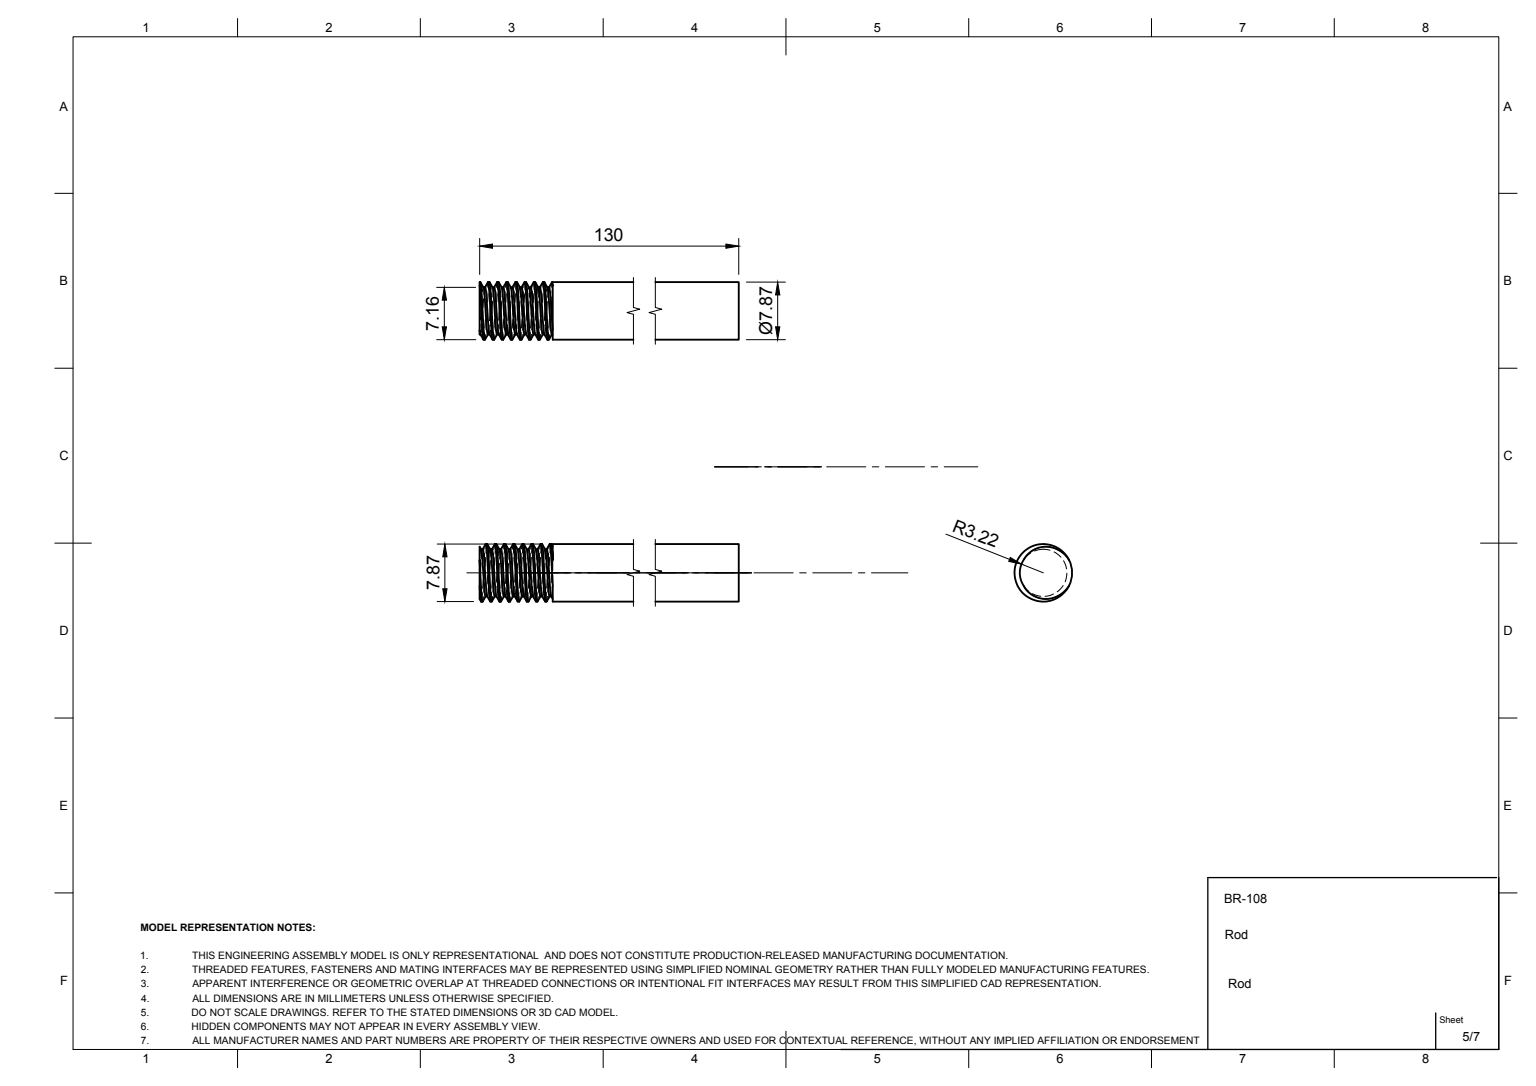
ISO-10303-21;
HEADER;
/* Generated by software containing ST-Developer
 * from STEP Tools, Inc. (www.steptools.com) 
 */

FILE_DESCRIPTION(
/* description */ (''),
/* implementation_level */ '2;1');

FILE_NAME(
/* name */ 'Rod.step',
/* time_stamp */ '2026-11-14T03:52:36-08:00',
/* author */ (''),
/* organization */ (''),
/* preprocessor_version */ 'ST-DEVELOPER v20.2',
/* originating_system */ 'Autodesk Translation Framework v15.17.0.0',
/* authorisation */ '');

FILE_SCHEMA (('AUTOMOTIVE_DESIGN { 1 0 10303 214 3 1 1 }'));
ENDSEC;

DATA;
#10=MECHANICAL_DESIGN_GEOMETRIC_PRESENTATION_REPRESENTATION('',(#193),#19443);
#43=B_SPLINE_SURFACE_WITH_KNOTS('',3,3,((#8954,#8955,#8956,#8957,#8958,
#8959,#8960,#8961,#8962,#8963,#8964,#8965,#8966,#8967,#8968,#8969,#8970,
#8971,#8972,#8973,#8974,#8975,#8976,#8977,#8978,#8979,#8980,#8981,#8982,
#8983,#8984,#8985,#8986,#8987,#8988,#8989,#8990,#8991,#8992,#8993,#8994,
#8995,#8996,#8997,#8998,#8999,#9000,#9001,#9002,#9003,#9004,#9005,#9006,
#9007,#9008,#9009),(#9010,#9011,#9012,#9013,#9014,#9015,#9016,#9017,#9018,
#9019,#9020,#9021,#9022,#9023,#9024,#9025,#9026,#9027,#9028,#9029,#9030,
#9031,#9032,#9033,#9034,#9035,#9036,#9037,#9038,#9039,#9040,#9041,#9042,
#9043,#9044,#9045,#9046,#9047,#9048,#9049,#9050,#9051,#9052,#9053,#9054,
#9055,#9056,#9057,#9058,#9059,#9060,#9061,#9062,#9063,#9064,#9065),(#9066,
#9067,#9068,#9069,#9070,#9071,#9072,#9073,#9074,#9075,#9076,#9077,#9078,
#9079,#9080,#9081,#9082,#9083,#9084,#9085,#9086,#9087,#9088,#9089,#9090,
#9091,#9092,#9093,#9094,#9095,#9096,#9097,#9098,#9099,#9100,#9101,#9102,
#9103,#9104,#9105,#9106,#9107,#9108,#9109,#9110,#9111,#9112,#9113,#9114,
#9115,#9116,#9117,#9118,#9119,#9120,#9121),(#9122,#9123,#9124,#9125,#9126,
#9127,#9128,#9129,#9130,#9131,#9132,#9133,#9134,#9135,#9136,#9137,#9138,
#9139,#9140,#9141,#9142,#9143,#9144,#9145,#9146,#9147,#9148,#9149,#9150,
#9151,#9152,#9153,#9154,#9155,#9156,#9157,#9158,#9159,#9160,#9161,#9162,
#9163,#9164,#9165,#9166,#9167,#9168,#9169,#9170,#9171,#9172,#9173,#9174,
#9175,#9176,#9177)),.UNSPECIFIED.,.F.,.F.,.F.,(4,4),(4,1,1,1,1,1,1,1,1,
1,1,1,1,1,1,1,1,1,1,1,1,1,1,1,1,1,1,1,1,1,1,1,1,1,1,1,1,1,1,1,1,1,1,1,1,
1,1,1,1,1,1,1,1,4),(-0.000657437329809864,0.0823479142293904),(8.31473274985805,
9.30202867542319,10.2893246009883,11.2766205265535,12.2639164521186,13.2512123776837,
14.2385083032489,15.225804228814,16.2131001543792,17.2003960799443,18.1876920055094,
19.1749879310746,20.1622838566397,21.1495797822049,22.13687570777,23.1241716333351,
24.1114675589003,25.0987634844654,26.0860594100306,27.0733553355957,28.0606512611608,
29.047947186726,30.0352431122911,31.0225390378563,32.0098349634214,32.9971308889865,
33.9844268145517,34.9717227401168,35.959018665682,36.9463145912471,37.9336105168122,
38.9209064423774,39.9082023679425,40.8954982935077,41.8827942190728,42.8700901446379,
43.8573860702031,44.8446819957682,45.8319779213334,46.8192738468985,47.8065697724636,
48.7938656980288,49.7811616235939,50.7684575491591,51.7557534747242,52.7430494002893,
53.7303453258545,54.7176412514196,55.7049371769848,56.6922331025499,57.679529028115,
58.6668249536802,59.6541208792453,60.6420742421403),.UNSPECIFIED.);
#44=B_SPLINE_SURFACE_WITH_KNOTS('',3,3,((#9461,#9462,#9463,#9464,#9465,
#9466,#9467,#9468,#9469,#9470,#9471,#9472,#9473,#9474,#9475,#9476,#9477,
#9478,#9479,#9480,#9481,#9482,#9483,#9484,#9485,#9486,#9487,#9488,#9489,
#9490,#9491,#9492,#9493,#9494,#9495,#9496,#9497,#9498,#9499,#9500,#9501,
#9502,#9503,#9504,#9505,#9506,#9507,#9508,#9509,#9510,#9511,#9512,#9513,
#9514,#9515,#9516),(#9517,#9518,#9519,#9520,#9521,#9522,#9523,#9524,#9525,
#9526,#9527,#9528,#9529,#9530,#9531,#9532,#9533,#9534,#9535,#9536,#9537,
#9538,#9539,#9540,#9541,#9542,#9543,#9544,#9545,#9546,#9547,#9548,#9549,
#9550,#9551,#9552,#9553,#9554,#9555,#9556,#9557,#9558,#9559,#9560,#9561,
#9562,#9563,#9564,#9565,#9566,#9567,#9568,#9569,#9570,#9571,#9572),(#9573,
#9574,#9575,#9576,#9577,#9578,#9579,#9580,#9581,#9582,#9583,#9584,#9585,
#9586,#9587,#9588,#9589,#9590,#9591,#9592,#9593,#9594,#9595,#9596,#9597,
#9598,#9599,#9600,#9601,#9602,#9603,#9604,#9605,#9606,#9607,#9608,#9609,
#9610,#9611,#9612,#9613,#9614,#9615,#9616,#9617,#9618,#9619,#9620,#9621,
#9622,#9623,#9624,#9625,#9626,#9627,#9628),(#9629,#9630,#9631,#9632,#9633,
#9634,#9635,#9636,#9637,#9638,#9639,#9640,#9641,#9642,#9643,#9644,#9645,
#9646,#9647,#9648,#9649,#9650,#9651,#9652,#9653,#9654,#9655,#9656,#9657,
#9658,#9659,#9660,#9661,#9662,#9663,#9664,#9665,#9666,#9667,#9668,#9669,
#9670,#9671,#9672,#9673,#9674,#9675,#9676,#9677,#9678,#9679,#9680,#9681,
#9682,#9683,#9684)),.UNSPECIFIED.,.F.,.F.,.F.,(4,4),(4,1,1,1,1,1,1,1,1,
1,1,1,1,1,1,1,1,1,1,1,1,1,1,1,1,1,1,1,1,1,1,1,1,1,1,1,1,1,1,1,1,1,1,1,1,
1,1,1,1,1,1,1,1,4),(-0.00040521448804481,0.0826859266002323),(11.6145409068929,
12.6025101533199,13.589806078885,14.5771020044501,15.5643979300153,16.5516938555804,
17.5389897811456,18.5262857067107,19.5135816322758,20.500877557841,21.4881734834061,
22.4754694089713,23.4627653345364,24.4500612601015,25.4373571856667,26.4246531112318,
27.411949036797,28.3992449623621,29.3865408879273,30.3738368134924,31.3611327390575,
32.3484286646227,33.3357245901878,34.323020515753,35.3103164413181,36.2976123668832,
37.2849082924484,38.2722042180135,39.2595001435787,40.2467960691438,41.2340919947089,
42.2213879202741,43.2086838458392,44.1959797714044,45.1832756969695,46.1705716225347,
47.1578675480998,48.1451634736649,49.1324593992301,50.1197553247952,51.1070512503604,
52.0943471759255,53.0816431014906,54.0689390270558,55.0562349526209,56.0435308781861,
57.0308268037512,58.0181227293163,59.0054186548815,59.9927145804466,60.9800105060118,
61.9673064315769,62.954602357142,63.9418982827072),.UNSPECIFIED.);
#49=B_SPLINE_CURVE_WITH_KNOTS('',3,(#2726,#2727,#2728,#2729,#2730,#2731,
#2732,#2733,#2734,#2735,#2736,#2737,#2738,#2739,#2740,#2741,#2742,#2743,
#2744,#2745,#2746,#2747,#2748,#2749,#2750,#2751,#2752,#2753,#2754,#2755,
#2756,#2757,#2758,#2759,#2760,#2761,#2762,#2763,#2764,#2765,#2766,#2767,
#2768,#2769,#2770,#2771,#2772,#2773,#2774,#2775,#2776,#2777,#2778,#2779,
#2780,#2781,#2782,#2783,#2784,#2785,#2786,#2787,#2788,#2789,#2790,#2791,
#2792,#2793,#2794,#2795,#2796,#2797,#2798,#2799,#2800,#2801,#2802,#2803,
#2804,#2805,#2806,#2807,#2808,#2809,#2810,#2811,#2812,#2813,#2814,#2815,
#2816,#2817,#2818,#2819,#2820,#2821,#2822,#2823,#2824,#2825,#2826,#2827,
#2828,#2829,#2830,#2831,#2832,#2833,#2834,#2835,#2836,#2837),
 .UNSPECIFIED.,.F.,.F.,(4,3,3,3,3,3,3,3,3,3,3,3,3,3,3,3,3,3,3,3,3,3,3,3,
3,3,3,3,3,3,3,3,3,3,3,3,3,4),(10.3764175401129,10.4684762321019,10.560419481767,
10.6522725450313,10.7440770571527,10.8358588565194,10.9276437548813,11.0195141021843,
11.1114281051697,11.2034893563628,11.2766205265535,11.3699699521422,11.4631985738672,
11.5563335991914,11.6494062321449,11.7424472221572,11.8354810277323,11.9285320946886,
12.0216816252994,12.11488490924,12.2082354140953,12.2639164521186,12.3570693480044,
12.4500982166783,12.5430305679426,12.6358970169529,12.7287297400997,12.8215534563738,
12.9143928706346,13.0073296432903,13.1003192457673,13.1934566991756,13.2512123776837,
13.3444476686996,13.4375356185427,13.5305385459024,13.6234740197825,13.6618555532241),
 .UNSPECIFIED.);
#50=B_SPLINE_CURVE_WITH_KNOTS('',3,(#2840,#2841,#2842,#2843,#2844,#2845,
#2846,#2847,#2848,#2849,#2850,#2851,#2852,#2853,#2854,#2855,#2856,#2857,
#2858,#2859,#2860,#2861,#2862,#2863,#2864,#2865,#2866,#2867,#2868,#2869,
#2870,#2871,#2872,#2873,#2874,#2875,#2876,#2877,#2878,#2879,#2880,#2881,
#2882,#2883,#2884,#2885,#2886,#2887,#2888,#2889,#2890,#2891,#2892,#2893,
#2894,#2895,#2896,#2897),.UNSPECIFIED.,.F.,.F.,(4,2,2,2,2,2,2,2,2,2,2,2,
2,2,2,2,2,2,2,2,2,2,2,2,2,2,2,2,4),(-3.35276873050689,-3.34541163931656,
-3.33454410942102,-3.28988621968237,-3.2367451420787,-3.21797771526182,
-3.20584415076294,-3.19380116055654,-3.17568959207908,-3.10036172591383,
-3.06621207860194,-3.05209120789862,-3.04101266877526,-3.03450717101804,
-3.02822963770033,-3.01796361528236,-2.95640611952485,-2.90263005834274,
-2.88767690300836,-2.87719641995359,-2.86629447482556,-2.84906124499233,
-2.78107728025335,-2.72943250313414,-2.7194202959918,-2.71333138514061,
-2.70696516579511,-2.6963401900384,-2.69172026756216),.UNSPECIFIED.);
#51=B_SPLINE_CURVE_WITH_KNOTS('',3,(#2903,#2904,#2905,#2906,#2907,#2908,
#2909,#2910,#2911,#2912,#2913,#2914,#2915,#2916,#2917,#2918,#2919,#2920,
#2921,#2922,#2923,#2924,#2925,#2926,#2927,#2928,#2929,#2930,#2931,#2932,
#2933,#2934,#2935,#2936,#2937,#2938,#2939,#2940,#2941,#2942,#2943,#2944,
#2945,#2946,#2947,#2948,#2949,#2950,#2951,#2952,#2953,#2954,#2955,#2956,
#2957,#2958,#2959,#2960,#2961,#2962,#2963,#2964,#2965,#2966,#2967,#2968,
#2969,#2970,#2971,#2972,#2973,#2974,#2975,#2976,#2977,#2978,#2979,#2980,
#2981,#2982,#2983,#2984,#2985,#2986,#2987,#2988,#2989,#2990,#2991,#2992,
#2993,#2994,#2995,#2996,#2997,#2998,#2999,#3000,#3001,#3002,#3003,#3004,
#3005,#3006,#3007,#3008,#3009,#3010,#3011,#3012,#3013,#3014,#3015,#3016,
#3017,#3018),.UNSPECIFIED.,.F.,.F.,(4,2,2,2,2,2,2,2,2,2,2,2,2,2,2,2,2,2,
2,2,2,2,2,2,2,2,2,2,2,2,2,2,2,2,2,2,2,2,2,2,2,2,2,2,2,2,2,2,2,2,2,2,2,2,
2,2,2,4),(-1.36964803891745,-1.30750439248835,-1.29117702151389,-1.28131054610571,
-1.27046681979769,-1.25480347710278,-1.19411610031767,-1.13876432373534,
-1.12764923556203,-1.12116620037127,-1.11483314340789,-1.10444786024198,
-1.09141491148914,-1.06110808838298,-0.988304024651697,-0.972093214280928,
-0.962245862176411,-0.951384177567935,-0.93561404698589,-0.876136217249594,
-0.819739530316951,-0.808663581702881,-0.802188694069041,-0.795848406891141,
-0.785428692256478,-0.772337850319824,-0.741796767684607,-0.669493053605558,
-0.653213006000507,-0.643353819682297,-0.632501979477615,-0.61679356347468,
-0.598449431655796,-0.560112935304642,-0.500216729476669,-0.489459341196301,
-0.483049710050318,-0.476646785775137,-0.465925187741241,-0.452320896136076,
-0.419631521650988,-0.351744719600656,-0.334921971516567,-0.323870468080585,
-0.312913218242703,-0.296609562925145,-0.237881919328277,-0.18192230055348,
-0.170826288952788,-0.164346905178106,-0.15801332963989,-0.147617386068845,
-0.134565346412738,-0.104177970967796,-0.0340764265464484,-0.0169290231420096,
-0.00796895088548166,-0.000909006770802341),.UNSPECIFIED.);
#52=B_SPLINE_CURVE_WITH_KNOTS('',3,(#3019,#3020,#3021,#3022,#3023,#3024,
#3025,#3026,#3027,#3028,#3029,#3030,#3031,#3032,#3033,#3034,#3035,#3036,
#3037,#3038,#3039,#3040,#3041,#3042,#3043,#3044,#3045,#3046,#3047,#3048,
#3049,#3050,#3051,#3052,#3053,#3054,#3055,#3056,#3057,#3058,#3059,#3060,
#3061,#3062,#3063,#3064,#3065,#3066,#3067,#3068,#3069,#3070,#3071,#3072,
#3073,#3074,#3075,#3076,#3077,#3078,#3079,#3080,#3081,#3082,#3083,#3084,
#3085,#3086,#3087,#3088),.UNSPECIFIED.,.F.,.F.,(4,3,3,3,3,3,3,3,3,3,3,3,
3,3,3,3,3,3,3,3,3,3,3,4),(13.6618555532241,13.7547559501353,13.8476578284241,
13.9453704471303,14.0384037073382,14.1315001278033,14.2247319191675,14.2385083032489,
14.3317395576815,14.4248478824819,14.5178606701666,14.6108086845596,14.7037236383471,
14.7966301491715,14.8895528209867,14.9825730552894,15.0756463542335,15.1688670547424,
15.225804228814,15.3242048935619,15.422335295086,15.5203045747014,15.6180521915914,
15.7079632677538),.UNSPECIFIED.);
#53=B_SPLINE_CURVE_WITH_KNOTS('',3,(#3089,#3090,#3091,#3092,#3093,#3094,
#3095,#3096,#3097,#3098,#3099,#3100,#3101,#3102,#3103,#3104,#3105,#3106,
#3107,#3108,#3109,#3110,#3111,#3112,#3113,#3114,#3115,#3116,#3117,#3118,
#3119,#3120,#3121,#3122,#3123,#3124,#3125,#3126,#3127,#3128,#3129,#3130,
#3131,#3132,#3133,#3134,#3135,#3136,#3137,#3138,#3139,#3140,#3141,#3142,
#3143,#3144,#3145,#3146,#3147,#3148,#3149,#3150,#3151,#3152,#3153,#3154,
#3155,#3156,#3157,#3158,#3159,#3160,#3161,#3162,#3163,#3164,#3165,#3166,
#3167,#3168,#3169,#3170,#3171,#3172,#3173,#3174,#3175,#3176,#3177,#3178,
#3179,#3180,#3181,#3182,#3183,#3184,#3185,#3186,#3187,#3188,#3189,#3190,
#3191,#3192,#3193,#3194,#3195,#3196,#3197,#3198,#3199,#3200,#3201,#3202,
#3203,#3204,#3205,#3206,#3207,#3208,#3209,#3210,#3211,#3212,#3213,#3214,
#3215,#3216,#3217,#3218,#3219,#3220,#3221,#3222,#3223,#3224,#3225,#3226,
#3227,#3228,#3229,#3230,#3231,#3232,#3233,#3234,#3235,#3236,#3237,#3238,
#3239,#3240,#3241,#3242,#3243,#3244,#3245,#3246,#3247,#3248),
 .UNSPECIFIED.,.F.,.F.,(4,2,2,2,2,2,2,2,2,2,2,2,2,2,2,2,2,2,2,2,2,2,2,2,
2,2,2,2,2,2,2,2,2,2,2,2,2,2,2,2,2,2,2,2,2,2,2,2,2,2,2,2,2,2,2,2,2,2,2,2,
2,2,2,2,2,2,2,2,2,2,2,2,2,2,2,2,2,2,2,4),(-2.69172026756216,-2.6352719778585,
-2.58053932952011,-2.56403952316667,-2.55298302906342,-2.54184725993664,
-2.52489765210718,-2.46049400488895,-2.4134571930637,-2.40261993901256,
-2.39612873883492,-2.3896297153635,-2.37859563248551,-2.32113463283633,
-2.26300703893396,-2.24709631499146,-2.23615960029177,-2.2262535246208,
-2.20995871418767,-2.13731879481618,-2.10689703379286,-2.09381670889935,
-2.08339320333483,-2.07703103205796,-2.07055590922739,-2.05943586161933,
-2.00451879050627,-1.94524564423088,-1.92879744188377,-1.91784270207866,
-1.90687315290747,-1.89034526278203,-1.81964968414538,-1.77336629031843,
-1.76352733265447,-1.75731584664119,-1.75069706235437,-1.73893559740849,
-1.67703680599441,-1.62753135510787,-1.61022061477051,-1.59906379949906,
-1.58815412521391,-1.57220494550319,-1.55348415739971,-1.51368071751401,
-1.45693404941784,-1.44588190611916,-1.43940053463916,-1.43303563482373,
-1.4225301442536,-1.37391976247168,-1.30842245398281,-1.29135232087876,
-1.28024526635582,-1.26930938300003,-1.2531824727869,-1.19460878790403,
-1.1380281402389,-1.1269544534409,-1.12047486614745,-1.11412652524273,-1.10368073934768,
-1.09054784637145,-1.05984279983027,-0.987904838680315,-0.97157369331838,
-0.961702447578007,-0.950851274858951,-0.93517204277001,-0.91687745879115,
-0.878744533463983,-0.818394879822658,-0.807684334784296,-0.801282660555561,
-0.794863494461416,-0.784079266325534,-0.736541400956773,-0.670341716572371,
-0.662034792948836),.UNSPECIFIED.);
#54=B_SPLINE_CURVE_WITH_KNOTS('',3,(#3253,#3254,#3255,#3256,#3257,#3258,
#3259,#3260,#3261,#3262,#3263,#3264,#3265,#3266,#3267,#3268,#3269,#3270,
#3271,#3272,#3273,#3274,#3275,#3276,#3277,#3278,#3279,#3280,#3281,#3282,
#3283,#3284,#3285,#3286,#3287,#3288,#3289,#3290,#3291,#3292,#3293,#3294,
#3295,#3296,#3297,#3298,#3299,#3300,#3301,#3302,#3303,#3304,#3305,#3306,
#3307,#3308,#3309,#3310,#3311,#3312,#3313,#3314,#3315,#3316,#3317,#3318,
#3319,#3320,#3321,#3322,#3323,#3324,#3325,#3326,#3327,#3328,#3329,#3330,
#3331,#3332,#3333,#3334,#3335,#3336,#3337,#3338,#3339,#3340,#3341,#3342,
#3343,#3344,#3345,#3346,#3347,#3348,#3349,#3350,#3351,#3352,#3353,#3354,
#3355,#3356,#3357,#3358,#3359,#3360,#3361,#3362,#3363,#3364,#3365,#3366,
#3367,#3368,#3369,#3370,#3371,#3372,#3373,#3374,#3375,#3376,#3377,#3378,
#3379,#3380,#3381,#3382,#3383,#3384,#3385,#3386,#3387,#3388,#3389,#3390,
#3391,#3392,#3393,#3394,#3395,#3396,#3397,#3398,#3399,#3400,#3401,#3402,
#3403,#3404,#3405,#3406,#3407,#3408,#3409,#3410,#3411,#3412,#3413,#3414,
#3415,#3416,#3417,#3418,#3419,#3420,#3421,#3422,#3423,#3424,#3425,#3426,
#3427,#3428,#3429,#3430),.UNSPECIFIED.,.F.,.F.,(4,2,2,2,2,2,2,2,2,2,2,2,
2,2,2,2,2,2,2,2,2,2,2,2,2,2,2,2,2,2,2,2,2,2,2,2,2,2,2,2,2,2,2,2,2,2,2,2,
2,2,2,2,2,2,2,2,2,2,2,2,2,2,2,2,2,2,2,2,2,2,2,2,2,2,2,2,2,2,2,2,2,2,2,2,
2,2,2,2,4),(-3.39903664743057,-3.36922949716159,-3.35907016472613,-3.35278253154188,
-3.34624369901061,-3.33485442673028,-3.28197372785829,-3.21962138318406,
-3.20385669522807,-3.19299651463027,-3.18314892719787,-3.16693426233528,
-3.09411928565292,-3.06379295586029,-3.05075490729438,-3.04036761404322,
-3.03403448904572,-3.02755269167242,-3.01644165787922,-2.96108432315832,
-2.90045754548251,-2.88480463462061,-2.87396358925092,-2.86409652646892,
-2.84776137026498,-2.77584054112386,-2.74509775457727,-2.73195758796762,
-2.72150990534484,-2.7151645690845,-2.70869698255478,-2.69765504586794,
-2.64078732021274,-2.58206388998048,-2.56617714578574,-2.55529582090197,
-2.54415894673355,-2.5268644748549,-2.47932311619691,-2.43272354330095,
-2.41636129984253,-2.40408963303116,-2.39737281942042,-2.3912707165942,
-2.38177347981764,-2.3481760968759,-2.29029580853658,-2.26789630846598,
-2.24972523294346,-2.23842305127295,-2.22776912237473,-2.21260571020353,
-2.16248563807822,-2.11434921241432,-2.09773424810769,-2.08532581046688,
-2.07858164020483,-2.07249240692179,-2.06307048429426,-2.03081936839389,
-1.97559527017083,-1.9405180689747,-1.92767654069113,-1.91700738834137,
-1.90573216466856,-1.88770565492006,-1.86555124005718,-1.80919432109441,
-1.77362524087514,-1.76405303472052,-1.75793753584351,-1.75124596386142,
-1.73910228569866,-1.7229773003303,-1.67776166540375,-1.62843024292933,
-1.61114088252377,-1.60000448577954,-1.58912150796141,-1.57322857549015,
-1.51442843009721,-1.45758331869308,-1.44653422535539,-1.44006485634313,
-1.43371982394962,-1.42327628194991,-1.41014495002222,-1.37943716657379,
-1.36964803891745),.UNSPECIFIED.);
#55=B_SPLINE_CURVE_WITH_KNOTS('',3,(#3432,#3433,#3434,#3435,#3436,#3437,
#3438,#3439,#3440,#3441,#3442,#3443,#3444,#3445,#3446,#3447,#3448,#3449,
#3450,#3451,#3452,#3453,#3454,#3455,#3456,#3457,#3458,#3459,#3460,#3461,
#3462,#3463,#3464,#3465,#3466,#3467,#3468,#3469,#3470,#3471,#3472,#3473,
#3474,#3475,#3476,#3477,#3478,#3479,#3480,#3481,#3482,#3483,#3484,#3485,
#3486,#3487,#3488,#3489),.UNSPECIFIED.,.F.,.F.,(4,2,2,2,2,2,2,2,2,2,2,2,
2,2,2,2,2,2,2,2,2,2,2,2,2,2,2,2,4),(-0.662034792948836,-0.653334308078723,
-0.642240876193188,-0.631298979652384,-0.615126147845094,-0.558854990744257,
-0.499712483035183,-0.488868934274772,-0.482436762461079,-0.476041922576952,
-0.465376724725386,-0.451872151391653,-0.419622602034269,-0.350862918782535,
-0.334130010188623,-0.32308782579176,-0.312102313169959,-0.295681606448517,
-0.240217946299654,-0.180688818274785,-0.169885524452651,-0.163462444525048,
-0.157060866801764,-0.146361255485615,-0.100197793993894,-0.0337464379318014,
-0.0164341699529654,-0.00773988275201024,-0.000934617407798161),
 .UNSPECIFIED.);
#56=B_SPLINE_CURVE_WITH_KNOTS('',3,(#3490,#3491,#3492,#3493,#3494,#3495,
#3496,#3497,#3498,#3499,#3500,#3501,#3502,#3503,#3504,#3505,#3506,#3507,
#3508,#3509,#3510,#3511,#3512,#3513,#3514,#3515,#3516,#3517,#3518,#3519,
#3520,#3521,#3522,#3523,#3524,#3525,#3526,#3527,#3528,#3529,#3530,#3531,
#3532,#3533,#3534,#3535,#3536,#3537,#3538,#3539,#3540,#3541,#3542,#3543,
#3544,#3545,#3546,#3547,#3548,#3549,#3550,#3551,#3552,#3553,#3554,#3555,
#3556,#3557,#3558,#3559,#3560,#3561,#3562,#3563,#3564,#3565,#3566,#3567,
#3568,#3569,#3570,#3571,#3572,#3573,#3574,#3575,#3576,#3577,#3578,#3579,
#3580,#3581,#3582,#3583,#3584,#3585,#3586,#3587,#3588,#3589,#3590,#3591,
#3592,#3593,#3594,#3595,#3596,#3597,#3598,#3599,#3600,#3601,#3602,#3603,
#3604,#3605),.UNSPECIFIED.,.F.,.F.,(4,2,2,2,2,2,2,2,2,2,2,2,2,2,2,2,2,2,
2,2,2,2,2,2,2,2,2,2,2,2,2,2,2,2,2,2,2,2,2,2,2,2,2,2,2,2,2,2,2,2,2,2,2,2,
2,2,2,4),(-4.05961831363024,-4.04941971591903,-4.03366125775226,-3.96879386302192,
-3.91912535132764,-3.90901225897516,-3.90272988290464,-3.89616876119144,
-3.88468934003338,-3.84670355831125,-3.79478196793746,-3.77341541293937,
-3.75585035176678,-3.74465509405993,-3.73392111606877,-3.71831307817265,
-3.6412008837597,-3.6127881932907,-3.60022959663044,-3.59012613039812,-3.58384522078611,
-3.57728091650738,-3.56578654616062,-3.51421207719407,-3.4715275359027,
-3.45210730791552,-3.43572344931073,-3.42474592312127,-3.41369891317093,
-3.39693282190431,-3.32842069065548,-3.29601708814427,-3.28247633892739,
-3.27179131459786,-3.26539331721021,-3.25896832690889,-3.24815289206938,
-3.18881927595919,-3.15025592705087,-3.13185057655645,-3.11609959348404,
-3.10523330941385,-3.09536970008021,-3.0791020399664,-3.00662330877959,
-2.97614498858093,-2.9630661899283,-2.95265273570601,-2.94631003919231,
-2.93982389023707,-2.9287122749783,-2.87320510605371,-2.81281539045674,
-2.79711436097577,-2.78625657025535,-2.77638416514615,-2.76006237935573,
-2.69113860699559),.UNSPECIFIED.);
#57=B_SPLINE_CURVE_WITH_KNOTS('',3,(#3611,#3612,#3613,#3614,#3615,#3616,
#3617,#3618,#3619,#3620,#3621,#3622,#3623,#3624,#3625,#3626,#3627,#3628,
#3629,#3630,#3631,#3632,#3633,#3634,#3635,#3636,#3637,#3638,#3639,#3640,
#3641,#3642,#3643,#3644,#3645,#3646,#3647,#3648,#3649,#3650,#3651,#3652,
#3653,#3654,#3655,#3656,#3657,#3658,#3659,#3660,#3661,#3662,#3663,#3664,
#3665,#3666,#3667,#3668,#3669,#3670,#3671,#3672,#3673,#3674,#3675,#3676,
#3677,#3678,#3679,#3680,#3681,#3682,#3683,#3684,#3685,#3686,#3687,#3688,
#3689,#3690,#3691,#3692,#3693,#3694,#3695,#3696,#3697,#3698,#3699,#3700,
#3701,#3702,#3703,#3704,#3705,#3706,#3707,#3708,#3709,#3710,#3711,#3712,
#3713,#3714,#3715,#3716,#3717,#3718,#3719,#3720,#3721,#3722,#3723,#3724,
#3725,#3726,#3727,#3728),.UNSPECIFIED.,.F.,.F.,(4,2,2,2,2,2,2,2,2,2,2,2,
2,2,2,2,2,2,2,2,2,2,2,2,2,2,2,2,2,2,2,2,2,2,2,2,2,2,2,2,2,2,2,2,2,2,2,2,
2,2,2,2,2,2,2,2,2,2,4),(-1.36981720180546,-1.3681188713628,-1.35725933449787,
-1.34150327593904,-1.32308317578451,-1.28445166156793,-1.22516009572961,
-1.21433640455159,-1.2079134779239,-1.20152601902886,-1.190874523418,-1.17738952808723,
-1.14520749098011,-1.07630348163935,-1.05959482152721,-1.04856560236975,
-1.03759164402872,-1.02118730242328,-1.00172714162737,-0.958863918280977,
-0.907422055019664,-0.895958161473722,-0.889403779861678,-0.88312663373266,
-0.873022947901647,-0.823002531995589,-0.758255589547942,-0.741127825549499,
-0.730021179212323,-0.719114203482184,-0.703086216509602,-0.640850055396504,
-0.588556123135333,-0.577047491753894,-0.570483825607396,-0.564212954139896,
-0.554142194544246,-0.54163678578329,-0.513418231789095,-0.435885961905594,
-0.420350257017512,-0.409635435298454,-0.398435739804043,-0.380811447536338,
-0.359338444274976,-0.306848831696698,-0.266233271860153,-0.256517046568699,
-0.250925382457069,-0.244473536378757,-0.233510144547139,-0.219488471898311,
-0.184965325355446,-0.119927069565731,-0.103025005849182,-0.0919601728866959,
-0.0810182857079528,-0.0647931581572279,-0.000906520888964826),
 .UNSPECIFIED.);
#58=B_SPLINE_CURVE_WITH_KNOTS('',3,(#3729,#3730,#3731,#3732,#3733,#3734,
#3735,#3736,#3737,#3738,#3739,#3740,#3741,#3742,#3743,#3744,#3745,#3746,
#3747,#3748,#3749,#3750,#3751,#3752,#3753,#3754,#3755,#3756,#3757,#3758,
#3759,#3760,#3761,#3762,#3763,#3764,#3765,#3766,#3767,#3768,#3769,#3770,
#3771,#3772,#3773,#3774,#3775,#3776,#3777,#3778,#3779,#3780,#3781,#3782,
#3783,#3784),.UNSPECIFIED.,.F.,.F.,(4,2,2,2,2,2,2,2,2,2,2,2,2,2,2,2,2,2,
2,2,2,2,2,2,2,2,2,4),(-4.05976150379792,-4.01900511118112,-4.00372888568568,
-3.99706579203473,-3.99074157164933,-3.98424909733907,-3.97308615513119,
-3.91656945385962,-3.85725742797153,-3.84157728669245,-3.83073156957618,
-3.82086928707462,-3.80456378366424,-3.73242006563606,-3.70178160465181,
-3.68866690442563,-3.67823425697505,-3.67189195132403,-3.66542082629823,
-3.65436176824041,-3.59775916499977,-3.53918587468513,-3.5231233860214,
-3.51221123784039,-3.50111365189575,-3.48403034160817,-3.41870744663764,
-3.39903664743057),.UNSPECIFIED.);
#59=B_SPLINE_CURVE_WITH_KNOTS('',3,(#3785,#3786,#3787,#3788,#3789,#3790,
#3791,#3792,#3793,#3794,#3795,#3796,#3797,#3798,#3799,#3800,#3801,#3802,
#3803,#3804,#3805,#3806,#3807,#3808,#3809,#3810,#3811,#3812,#3813,#3814,
#3815,#3816,#3817,#3818,#3819,#3820,#3821,#3822,#3823,#3824,#3825,#3826,
#3827,#3828,#3829,#3830,#3831,#3832,#3833,#3834,#3835,#3836,#3837,#3838,
#3839,#3840,#3841,#3842,#3843,#3844,#3845,#3846,#3847,#3848,#3849,#3850,
#3851,#3852,#3853,#3854,#3855,#3856,#3857,#3858,#3859,#3860,#3861,#3862,
#3863,#3864,#3865,#3866,#3867,#3868,#3869,#3870,#3871,#3872,#3873,#3874,
#3875,#3876,#3877,#3878,#3879,#3880,#3881,#3882,#3883,#3884,#3885,#3886,
#3887,#3888,#3889,#3890,#3891,#3892,#3893,#3894,#3895,#3896,#3897,#3898,
#3899,#3900,#3901,#3902,#3903,#3904,#3905,#3906,#3907,#3908,#3909,#3910,
#3911,#3912,#3913,#3914,#3915,#3916,#3917,#3918,#3919,#3920,#3921,#3922,
#3923,#3924,#3925,#3926,#3927,#3928,#3929,#3930,#3931,#3932,#3933,#3934,
#3935,#3936,#3937,#3938,#3939,#3940,#3941,#3942,#3943,#3944,#3945,#3946,
#3947,#3948,#3949,#3950,#3951,#3952,#3953,#3954,#3955,#3956,#3957,#3958,
#3959,#3960,#3961,#3962,#3963,#3964),.UNSPECIFIED.,.F.,.F.,(4,2,2,2,2,2,
2,2,2,2,2,2,2,2,2,2,2,2,2,2,2,2,2,2,2,2,2,2,2,2,2,2,2,2,2,2,2,2,2,2,2,2,
2,2,2,2,2,2,2,2,2,2,2,2,2,2,2,2,2,2,2,2,2,2,2,2,2,2,2,2,2,2,2,2,2,2,2,2,
2,2,2,2,2,2,2,2,2,2,2,4),(-2.69113860699559,-2.68798641270898,-2.65732048758469,
-2.6441957050177,-2.63375504946037,-2.62740682579674,-2.62092706332233,
-2.60984650514142,-2.55354048871653,-2.49436614744855,-2.47845167620463,
-2.46755708279682,-2.45641033162421,-2.43910649863235,-2.38942595349833,
-2.34444481724778,-2.32835480078381,-2.31622898493564,-2.30953702939491,
-2.30341145852001,-2.29380726516983,-2.25763113264322,-2.20182075057012,
-2.17975829556766,-2.16178098829088,-2.15050742299244,-2.13981979878661,
-2.12693032583511,-2.09136959620799,-2.03000581693164,-2.00345394327482,
-1.99448025809388,-1.98839852765128,-1.98143124757679,-1.96789403242635,
-1.94913114223327,-1.88490277518901,-1.85197717243011,-1.83816279184475,
-1.82755156107063,-1.81577379888628,-1.79512201956957,-1.76828506562415,
-1.72308524164038,-1.6860054757428,-1.67636393420948,-1.6707812387932,-1.66429854220551,
-1.65320306393962,-1.63895485811311,-1.60341497517815,-1.54061867241779,
-1.52334944633781,-1.51220937656063,-1.50131012230862,-1.48536808094627,
-1.42556276183992,-1.36993616332764,-1.35882588238135,-1.35234009620102,
-1.34599709334049,-1.33558250789777,-1.32250316497891,-1.29201938113414,
-1.21962447199833,-1.20335376357977,-1.19348971912112,-1.18262382552945,
-1.16687554439054,-1.10608193557756,-1.05104877082362,-1.03991809875167,
-1.03342803251385,-1.02708841092747,-1.0166910281483,-1.0036408448629,-0.973276175239219,
-0.900621350267408,-0.884385297518919,-0.874526685836425,-0.863654915143497,
-0.847873423334712,-0.787349729372831,-0.7321027352839,-0.720979885217171,
-0.714491338462904,-0.708150183255675,-0.697745635827008,-0.684683444874573,
-0.661711247179129),.UNSPECIFIED.);
#60=B_SPLINE_CURVE_WITH_KNOTS('',3,(#3969,#3970,#3971,#3972,#3973,#3974,
#3975,#3976,#3977,#3978,#3979,#3980,#3981,#3982,#3983,#3984,#3985,#3986,
#3987,#3988,#3989,#3990,#3991,#3992,#3993,#3994,#3995,#3996,#3997,#3998,
#3999,#4000,#4001,#4002,#4003,#4004,#4005,#4006,#4007,#4008,#4009,#4010,
#4011,#4012,#4013,#4014,#4015,#4016,#4017,#4018,#4019,#4020,#4021,#4022,
#4023,#4024,#4025,#4026,#4027,#4028,#4029,#4030,#4031,#4032,#4033,#4034,
#4035,#4036,#4037,#4038,#4039,#4040,#4041,#4042,#4043,#4044,#4045,#4046,
#4047,#4048,#4049,#4050,#4051,#4052,#4053,#4054,#4055,#4056,#4057,#4058,
#4059,#4060,#4061,#4062,#4063,#4064,#4065,#4066,#4067,#4068,#4069,#4070,
#4071,#4072,#4073,#4074,#4075,#4076,#4077,#4078,#4079,#4080,#4081,#4082,
#4083,#4084,#4085,#4086,#4087,#4088,#4089,#4090,#4091,#4092,#4093,#4094,
#4095,#4096,#4097,#4098,#4099,#4100,#4101,#4102,#4103,#4104,#4105,#4106,
#4107,#4108,#4109,#4110,#4111,#4112,#4113,#4114,#4115,#4116,#4117,#4118,
#4119,#4120,#4121,#4122,#4123,#4124,#4125,#4126,#4127,#4128,#4129,#4130,
#4131,#4132,#4133,#4134,#4135,#4136),.UNSPECIFIED.,.F.,.F.,(4,2,2,2,2,2,
2,2,2,2,2,2,2,2,2,2,2,2,2,2,2,2,2,2,2,2,2,2,2,2,2,2,2,2,2,2,2,2,2,2,2,2,
2,2,2,2,2,2,2,2,2,2,2,2,2,2,2,2,2,2,2,2,2,2,2,2,2,2,2,2,2,2,2,2,2,2,2,2,
2,2,2,2,2,4),(-3.39942278040286,-3.36860646077918,-3.30661711098668,-3.29089667379652,
-3.28004385360924,-3.27018829158702,-3.25392549459415,-3.181459301777,-3.15096955861408,
-3.13789115452488,-3.12747989811296,-3.12114181025084,-3.11466542925515,
-3.10358134826762,-3.04744846003736,-2.9891769177977,-2.97277475043909,
-2.96180178103899,-2.95077308870415,-2.93406452113314,-2.86510808270885,
-2.83292156853096,-2.8194349560482,-2.80878352066393,-2.80239642731346,
-2.79597398138058,-2.7851516586564,-2.72591483166686,-2.68729596296793,
-2.66888070043975,-2.65312665475517,-2.64226783058902,-2.63241769664277,
-2.61618983721396,-2.54346049584816,-2.51309087869975,-2.50004184354062,
-2.48964788974661,-2.48331317394372,-2.47683243672944,-2.46572775980563,
-2.4101427310699,-2.34974837996218,-2.33408374219892,-2.32324021701081,
-2.31337449294839,-2.29705021717626,-2.2250362562185,-2.19433343314705,
-2.1812026904133,-2.17076041568238,-2.16441592584437,-2.15794655445302,
-2.14689714833195,-2.09012809837676,-2.03094814088529,-2.01522472499628,
-2.00447907371533,-1.99332736545466,-1.9759559845059,-1.92496161228227,
-1.86225808614346,-1.85182627721601,-1.8454838684314,-1.83901197204939,
-1.82795048098781,-1.8137582331815,-1.7784616874252,-1.71524122589339,-1.69800344107717,
-1.68687659084232,-1.67598615600202,-1.66005090821033,-1.60022607650516,
-1.54460087284301,-1.53349452438244,-1.52701335837661,-1.52067855549214,
-1.51028531743975,-1.49723902395652,-1.46687822163521,-1.39419612160138,
-1.37796907845977,-1.36981720180546),.UNSPECIFIED.);
#61=B_SPLINE_CURVE_WITH_KNOTS('',3,(#4138,#4139,#4140,#4141,#4142,#4143,
#4144,#4145,#4146,#4147,#4148,#4149,#4150,#4151,#4152,#4153,#4154,#4155,
#4156,#4157,#4158,#4159,#4160,#4161,#4162,#4163,#4164,#4165,#4166,#4167,
#4168,#4169,#4170,#4171,#4172,#4173,#4174,#4175,#4176,#4177,#4178,#4179,
#4180,#4181,#4182,#4183,#4184,#4185,#4186,#4187,#4188,#4189,#4190,#4191),
 .UNSPECIFIED.,.F.,.F.,(4,2,2,2,2,2,2,2,2,2,2,2,2,2,2,2,2,2,2,2,2,2,2,2,
2,2,4),(-0.661711247179129,-0.654270438906596,-0.581717180746494,-0.565466795777757,
-0.555605724287503,-0.544735994000254,-0.528967360918269,-0.468992020429739,
-0.413129166744064,-0.402025820592833,-0.395541194624966,-0.389196450444212,
-0.378774569908438,-0.365683181090854,-0.335151734656965,-0.262850577953034,
-0.246565590468353,-0.236698783708754,-0.225834321032208,-0.210097398454042,
-0.150731747581798,-0.0941220267533644,-0.0830532554658109,-0.0765756499766033,
-0.0702245991095249,-0.0597719941297826,-0.000906261498553894),
 .UNSPECIFIED.);
#62=B_SPLINE_CURVE_WITH_KNOTS('',3,(#4192,#4193,#4194,#4195,#4196,#4197,
#4198,#4199,#4200,#4201,#4202,#4203,#4204,#4205,#4206,#4207,#4208,#4209,
#4210,#4211,#4212,#4213,#4214,#4215,#4216,#4217,#4218,#4219,#4220,#4221,
#4222,#4223,#4224,#4225,#4226,#4227,#4228,#4229,#4230,#4231,#4232,#4233,
#4234,#4235,#4236,#4237,#4238,#4239,#4240,#4241,#4242,#4243,#4244,#4245,
#4246,#4247,#4248,#4249,#4250,#4251,#4252,#4253,#4254,#4255,#4256,#4257,
#4258,#4259,#4260,#4261,#4262,#4263,#4264,#4265,#4266,#4267,#4268,#4269,
#4270,#4271,#4272,#4273,#4274,#4275,#4276,#4277,#4278,#4279,#4280,#4281,
#4282,#4283,#4284,#4285,#4286,#4287,#4288,#4289,#4290,#4291,#4292,#4293,
#4294,#4295,#4296,#4297,#4298,#4299,#4300,#4301,#4302,#4303,#4304,#4305,
#4306,#4307),.UNSPECIFIED.,.F.,.F.,(4,2,2,2,2,2,2,2,2,2,2,2,2,2,2,2,2,2,
2,2,2,2,2,2,2,2,2,2,2,2,2,2,2,2,2,2,2,2,2,2,2,2,2,2,2,2,2,2,2,2,2,2,2,2,
2,2,2,4),(-4.06006106737699,-4.01750335279925,-3.99679661475175,-3.98597230434252,
-3.97513721085419,-3.96524400160451,-3.94878727173729,-3.87701512354494,
-3.84635395252591,-3.83323120657681,-3.82279217357101,-3.81644494367554,
-3.80996619369454,-3.79888739309778,-3.74258921628807,-3.68298461951677,
-3.66727133834649,-3.65641272700456,-3.64654443939987,-3.6302411468607,
-3.55805664022011,-3.52745122944711,-3.51434211880632,-3.5039111418175,
-3.49756553738962,-3.49108488766042,-3.47999686921938,-3.42389233184436,
-3.38364093332244,-3.36480936582705,-3.34879168219368,-3.33788008897764,
-3.32675855470048,-3.30958460206247,-3.2453173690025,-3.19512318986539,
-3.18488631148219,-3.17857952331764,-3.17205112158684,-3.16073081605242,
-3.09153482140168,-3.04526653381446,-3.02954790578215,-3.01868825256711,
-3.00882070279101,-2.99252267151132,-2.9202959297447,-2.88970923791968,
-2.87660462294926,-2.86617626172096,-2.85983112000475,-2.85334971532542,
-2.84225834448629,-2.78622659086253,-2.72621098959534,-2.71057131022136,
-2.69972510548116,-2.69144328541572),.UNSPECIFIED.);
#63=B_SPLINE_CURVE_WITH_KNOTS('',3,(#4313,#4314,#4315,#4316,#4317,#4318,
#4319,#4320,#4321,#4322,#4323,#4324,#4325,#4326,#4327,#4328,#4329,#4330,
#4331,#4332,#4333,#4334,#4335,#4336,#4337,#4338,#4339,#4340,#4341,#4342,
#4343,#4344,#4345,#4346,#4347,#4348,#4349,#4350,#4351,#4352,#4353,#4354,
#4355,#4356,#4357,#4358,#4359,#4360,#4361,#4362,#4363,#4364,#4365,#4366,
#4367,#4368,#4369,#4370,#4371,#4372,#4373,#4374,#4375,#4376,#4377,#4378,
#4379,#4380,#4381,#4382,#4383,#4384,#4385,#4386,#4387,#4388,#4389,#4390,
#4391,#4392,#4393,#4394,#4395,#4396,#4397,#4398,#4399,#4400,#4401,#4402,
#4403,#4404,#4405,#4406,#4407,#4408,#4409,#4410,#4411,#4412,#4413,#4414,
#4415,#4416,#4417,#4418,#4419,#4420,#4421,#4422,#4423,#4424,#4425,#4426,
#4427,#4428,#4429,#4430,#4431,#4432,#4433,#4434,#4435,#4436,#4437,#4438,
#4439,#4440,#4441,#4442),.UNSPECIFIED.,.F.,.F.,(4,2,2,2,2,2,2,2,2,2,2,2,
2,2,2,2,2,2,2,2,2,2,2,2,2,2,2,2,2,2,2,2,2,2,2,2,2,2,2,2,2,2,2,2,2,2,2,2,
2,2,2,2,2,2,2,2,2,2,2,2,2,2,2,2,4),(-1.36945801245357,-1.31142024483846,
-1.30064223896015,-1.29422830883802,-1.28783078031624,-1.27713254417671,
-1.26356810040954,-1.23105027367383,-1.16279279380772,-1.14600723349723,
-1.13496307828971,-1.12400073344613,-1.10766562054501,-1.08831820292282,
-1.04593815898459,-0.99387169077095,-0.982330811192836,-0.975760293128391,
-0.969493552026457,-0.959445472599736,-0.946978091374135,-0.918907391364276,
-0.841015863050523,-0.825531436441148,-0.814824528981982,-0.803610376227102,
-0.785912074939119,-0.764314985243115,-0.711154153356489,-0.671449111270555,
-0.661742398995181,-0.656152076178251,-0.649696954949905,-0.638719033331854,
-0.624672506223117,-0.590039617324983,-0.525679578965086,-0.508519715582898,
-0.497406577252715,-0.486503466719564,-0.470500512594571,-0.451687123957076,
-0.411505667934827,-0.35516082373592,-0.344081429726595,-0.337605473764751,
-0.331265281005552,-0.320847026760153,-0.307758819139739,-0.277229206573372,
-0.204899998177409,-0.18862312446602,-0.178764301512738,-0.167911687930887,
-0.152199756021093,-0.13385028428509,-0.0954945839976622,-0.078738321637529,
-0.0782343598820795,-0.0540345406664802,-0.0311753977701198,-0.0226064955066162,
-0.0166883237025578,-0.0110430614363735,-0.000905562748328462),
 .UNSPECIFIED.);
#64=B_SPLINE_CURVE_WITH_KNOTS('',3,(#4443,#4444,#4445,#4446,#4447,#4448,
#4449,#4450,#4451,#4452,#4453,#4454,#4455,#4456,#4457,#4458,#4459,#4460,
#4461,#4462,#4463,#4464,#4465,#4466,#4467,#4468,#4469,#4470,#4471,#4472,
#4473,#4474,#4475,#4476,#4477,#4478,#4479,#4480,#4481,#4482,#4483,#4484,
#4485,#4486,#4487,#4488,#4489,#4490,#4491,#4492,#4493,#4494,#4495,#4496,
#4497,#4498,#4499,#4500),.UNSPECIFIED.,.F.,.F.,(4,2,2,2,2,2,2,2,2,2,2,2,
2,2,2,2,2,2,2,2,2,2,2,2,2,2,2,2,4),(-4.06049499041426,-4.00144584921642,
-3.96288024512554,-3.94447915811091,-3.92873425089659,-3.91787742515527,
-3.90802638356343,-3.89179053725541,-3.8191300166447,-3.78873192773811,
-3.77567617873277,-3.76527839089358,-3.75894312369514,-3.75246376712777,
-3.74136473286814,-3.68562532702502,-3.6451432106023,-3.62625800758028,
-3.61020961699309,-3.5992997388205,-3.58819870002538,-3.5710979320657,-3.50597092402198,
-3.45651578954256,-3.44626001988021,-3.4399531399171,-3.43343884263639,
-3.42217007433208,-3.39942278040286),.UNSPECIFIED.);
#65=B_SPLINE_CURVE_WITH_KNOTS('',3,(#4501,#4502,#4503,#4504,#4505,#4506,
#4507,#4508,#4509,#4510,#4511,#4512,#4513,#4514,#4515,#4516,#4517,#4518,
#4519,#4520,#4521,#4522,#4523,#4524,#4525,#4526,#4527,#4528,#4529,#4530,
#4531,#4532,#4533,#4534,#4535,#4536,#4537,#4538,#4539,#4540,#4541,#4542,
#4543,#4544,#4545,#4546,#4547,#4548,#4549,#4550,#4551,#4552,#4553,#4554,
#4555,#4556,#4557,#4558,#4559,#4560,#4561,#4562,#4563,#4564,#4565,#4566,
#4567,#4568,#4569,#4570,#4571,#4572,#4573,#4574,#4575,#4576,#4577,#4578,
#4579,#4580,#4581,#4582,#4583,#4584,#4585,#4586,#4587,#4588,#4589,#4590,
#4591,#4592,#4593,#4594,#4595,#4596,#4597,#4598,#4599,#4600,#4601,#4602,
#4603,#4604,#4605,#4606,#4607,#4608,#4609,#4610,#4611,#4612,#4613,#4614,
#4615,#4616,#4617,#4618,#4619,#4620,#4621,#4622,#4623,#4624,#4625,#4626,
#4627,#4628,#4629,#4630,#4631,#4632,#4633,#4634,#4635,#4636,#4637,#4638,
#4639,#4640,#4641,#4642,#4643,#4644,#4645,#4646,#4647,#4648,#4649,#4650,
#4651,#4652,#4653,#4654,#4655,#4656,#4657,#4658,#4659,#4660,#4661,#4662,
#4663,#4664,#4665,#4666,#4667,#4668,#4669,#4670),.UNSPECIFIED.,.F.,.F.,
(4,2,2,2,2,2,2,2,2,2,2,2,2,2,2,2,2,2,2,2,2,2,2,2,2,2,2,2,2,2,2,2,2,2,2,
2,2,2,2,2,2,2,2,2,2,2,2,2,2,2,2,2,2,2,2,2,2,2,2,2,2,2,2,2,2,2,2,2,2,2,2,
2,2,2,2,2,2,2,2,2,2,2,2,2,4),(-2.69144328541572,-2.68984354191311,-2.6734590655946,
-2.60188261593871,-2.57099026285687,-2.5578110604289,-2.54733864671877,
-2.54098458216743,-2.53451345177249,-2.52347202960527,-2.46655502948031,
-2.42675887634366,-2.40804080870372,-2.39209402188225,-2.38119471500536,
-2.37005703621845,-2.35279703322566,-2.2897867238274,-2.25434268394012,
-2.24011463291027,-2.22903182543274,-2.22255217296172,-2.21696857426285,
-2.20731965679741,-2.16998655160728,-2.12990077757589,-2.08645651695713,
-2.07171127318128,-2.06100766230234,-2.04952231521939,-2.0304225382796,
-1.95320558070817,-1.9182698872082,-1.90872424528372,-1.90260931108544,
-1.8958978379517,-1.88367357207352,-1.8674042989991,-1.82136134023027,-1.77321295786483,
-1.7558882821052,-1.7447380060636,-1.73384682361741,-1.71795030763093,-1.6592432013438,
-1.60230439078201,-1.59125824821918,-1.58478572683239,-1.57843146322911,
-1.56796088219368,-1.554786700059,-1.52391432331564,-1.45235070424489,-1.43596962916131,
-1.42608783923466,-1.41523947059035,-1.3995930622834,-1.33873655493508,
-1.28352895692786,-1.27240522765314,-1.26591665706296,-1.25957596371069,
-1.24917292186661,-1.2361131060364,-1.2057089125561,-1.13314178524207,-1.11689425384144,
-1.10703391210559,-1.09616422354748,-1.08039406338827,-1.01840076745309,
-0.96491192182675,-0.953617134107769,-0.947093377713306,-0.940781185641492,
-0.930520787210808,-0.880910983917029,-0.816043382298155,-0.798919574871243,
-0.787806083072503,-0.776884739936868,-0.760819508783053,-0.741910938442555,
-0.701360367414784,-0.662002611929399),.UNSPECIFIED.);
#66=B_SPLINE_CURVE_WITH_KNOTS('',3,(#4675,#4676,#4677,#4678,#4679,#4680,
#4681,#4682,#4683,#4684,#4685,#4686,#4687,#4688,#4689,#4690,#4691,#4692,
#4693,#4694,#4695,#4696,#4697,#4698,#4699,#4700,#4701,#4702,#4703,#4704,
#4705,#4706,#4707,#4708,#4709,#4710,#4711,#4712,#4713,#4714,#4715,#4716,
#4717,#4718,#4719,#4720,#4721,#4722,#4723,#4724,#4725,#4726,#4727,#4728,
#4729,#4730,#4731,#4732,#4733,#4734,#4735,#4736,#4737,#4738,#4739,#4740,
#4741,#4742,#4743,#4744,#4745,#4746,#4747,#4748,#4749,#4750,#4751,#4752,
#4753,#4754,#4755,#4756,#4757,#4758,#4759,#4760,#4761,#4762,#4763,#4764,
#4765,#4766,#4767,#4768,#4769,#4770,#4771,#4772,#4773,#4774,#4775,#4776,
#4777,#4778,#4779,#4780,#4781,#4782,#4783,#4784,#4785,#4786,#4787,#4788,
#4789,#4790,#4791,#4792,#4793,#4794,#4795,#4796,#4797,#4798,#4799,#4800,
#4801,#4802,#4803,#4804,#4805,#4806,#4807,#4808,#4809,#4810,#4811,#4812,
#4813,#4814,#4815,#4816,#4817,#4818,#4819,#4820,#4821,#4822,#4823,#4824,
#4825,#4826,#4827,#4828,#4829,#4830,#4831,#4832,#4833,#4834,#4835,#4836,
#4837,#4838,#4839,#4840,#4841,#4842,#4843,#4844,#4845,#4846,#4847,#4848,
#4849,#4850,#4851,#4852,#4853,#4854),.UNSPECIFIED.,.F.,.F.,(4,2,2,2,2,2,
2,2,2,2,2,2,2,2,2,2,2,2,2,2,2,2,2,2,2,2,2,2,2,2,2,2,2,2,2,2,2,2,2,2,2,2,
2,2,2,2,2,2,2,2,2,2,2,2,2,2,2,2,2,2,2,2,2,2,2,2,2,2,2,2,2,2,2,2,2,2,2,2,
2,2,2,2,2,2,2,2,2,2,2,4),(-3.39931823127231,-3.39333264987127,-3.37756827591752,
-3.36670620862625,-3.35685556675115,-3.34063265312326,-3.26783032142072,
-3.23748196806637,-3.22443722634335,-3.21404537554358,-3.20771043435399,
-3.20122812368755,-3.19011814782567,-3.13464457245426,-3.07398882591856,
-3.05838385281095,-3.0475495776618,-3.03767179376624,-3.02127810996635,
-2.94975835780466,-2.91881082611094,-2.90561973271878,-2.89514150456081,
-2.88878926325972,-2.88232696973456,-2.87131519171508,-2.81399875021888,
-2.75560750759241,-2.73973186427994,-2.72885060565196,-2.71770773700242,
-2.70039086481708,-2.63847598162576,-2.60232605128182,-2.58794665558805,
-2.57677834537134,-2.57028388514838,-2.56395871948222,-2.5536158045003,
-2.4901750847304,-2.43966620504835,-2.42235596467229,-2.41121441925878,
-2.40045844217865,-2.38468223245109,-2.30871712696938,-2.27978735843464,
-2.26709804253308,-2.25691762101437,-2.2506248533669,-2.24408947435361,
-2.23272172362556,-2.16630689634555,-2.12634380276431,-2.10600922698734,
-2.09429691446114,-2.08368046666383,-2.06976763500726,-2.03638687518432,
-2.03024396124456,-1.98802964114676,-1.94725005922582,-1.93753186880774,
-1.93193951805665,-1.92548737399093,-1.91452445214204,-1.90050406163128,
-1.86598932803968,-1.80142067547124,-1.7842765179594,-1.77316607936646,
-1.76226027148026,-1.74624324958776,-1.72740752156719,-1.6871371509107,
-1.63094392166677,-1.61985703293382,-1.61337941640967,-1.60704032057634,
-1.59662804178187,-1.58355005322157,-1.55306269092771,-1.4806391556512,
-1.46437433870505,-1.45451727871944,-1.44366240155752,-1.42793847442011,
-1.40957012536622,-1.37114240909329,-1.36945801245357),.UNSPECIFIED.);
#67=B_SPLINE_CURVE_WITH_KNOTS('',3,(#4856,#4857,#4858,#4859,#4860,#4861,
#4862,#4863,#4864,#4865,#4866,#4867,#4868,#4869,#4870,#4871,#4872,#4873,
#4874,#4875,#4876,#4877,#4878,#4879,#4880,#4881,#4882,#4883,#4884,#4885,
#4886,#4887,#4888,#4889,#4890,#4891,#4892,#4893,#4894,#4895,#4896,#4897,
#4898,#4899,#4900,#4901,#4902,#4903,#4904,#4905,#4906,#4907,#4908,#4909,
#4910,#4911,#4912,#4913),.UNSPECIFIED.,.F.,.F.,(4,2,2,2,2,2,2,2,2,2,2,2,
2,2,2,2,2,2,2,2,2,2,2,2,2,2,2,2,4),(-0.662002611929399,-0.645673022059062,
-0.634564153273406,-0.628078498344257,-0.621734934376972,-0.611318364231216,
-0.598235837861409,-0.567739945548748,-0.495365854606088,-0.479091350770045,
-0.469226419918645,-0.458360624311453,-0.442614716404333,-0.382164873145699,
-0.326752710107995,-0.315635002362123,-0.309147441075794,-0.302805245738295,
-0.292395906945934,-0.279325698342569,-0.248880459281276,-0.176394415429904,
-0.16013448638823,-0.15027175151832,-0.13940332751517,-0.123643119994858,
-0.061539183838578,-0.0147529766196489,-0.000906767077203394),
 .UNSPECIFIED.);
#68=B_SPLINE_CURVE_WITH_KNOTS('',3,(#4914,#4915,#4916,#4917,#4918,#4919,
#4920,#4921,#4922,#4923,#4924,#4925,#4926,#4927,#4928,#4929,#4930,#4931,
#4932,#4933,#4934,#4935,#4936,#4937,#4938,#4939,#4940,#4941,#4942,#4943,
#4944,#4945,#4946,#4947,#4948,#4949,#4950,#4951,#4952,#4953,#4954,#4955,
#4956,#4957,#4958,#4959,#4960,#4961,#4962,#4963,#4964,#4965,#4966,#4967,
#4968,#4969,#4970,#4971,#4972,#4973,#4974,#4975,#4976,#4977,#4978,#4979,
#4980,#4981,#4982,#4983,#4984,#4985,#4986,#4987,#4988,#4989,#4990,#4991,
#4992,#4993,#4994,#4995,#4996,#4997,#4998,#4999,#5000,#5001,#5002,#5003,
#5004,#5005,#5006,#5007,#5008,#5009,#5010,#5011,#5012,#5013,#5014,#5015,
#5016,#5017,#5018,#5019,#5020,#5021,#5022,#5023,#5024,#5025,#5026,#5027,
#5028,#5029,#5030,#5031,#5032,#5033,#5034,#5035,#5036,#5037,#5038,#5039,
#5040,#5041,#5042,#5043,#5044,#5045,#5046,#5047,#5048,#5049,#5050,#5051,
#5052,#5053,#5054,#5055,#5056,#5057,#5058),.UNSPECIFIED.,.F.,.F.,(4,3,3,
3,3,3,3,3,3,3,3,3,3,3,3,3,3,3,3,3,3,3,3,3,3,3,3,3,3,3,3,3,3,3,3,3,3,3,3,
3,3,3,3,3,3,3,3,3,4),(47.1238898038469,47.1578675480998,47.2510868451706,
47.3441829801613,47.4371833640954,47.5301187067581,47.6230208283606,47.7159143623725,
47.8088239284592,47.9018309388297,47.994890928453,48.0880983142331,48.1451634736649,
48.2383827858837,48.3314789359493,48.4244793348657,48.5174146923123,48.6103168285705,
48.7032103770924,48.7961199575261,48.8891269819078,48.9821869853736,49.0753943845935,
49.1324593992301,49.2256787299236,49.3187748986893,49.4117753165029,49.5047106930589,
49.5976128485495,49.6905064164021,49.7834160162398,49.8764230600177,49.9694830829029,
50.0626905013858,50.1197553247952,50.2129745435564,50.3060706001924,50.3990709058328,
50.4920061706172,50.5849082146287,50.6778016714316,50.7707111607865,50.8637180956196,
50.95677801027,51.0499853227089,51.1070512503604,51.2002688732808,51.293351331344,
51.3612711115601),.UNSPECIFIED.);
#69=B_SPLINE_CURVE_WITH_KNOTS('',3,(#5064,#5065,#5066,#5067,#5068,#5069,
#5070,#5071,#5072,#5073,#5074,#5075,#5076,#5077,#5078,#5079,#5080,#5081,
#5082,#5083,#5084,#5085,#5086,#5087,#5088,#5089,#5090,#5091,#5092,#5093,
#5094,#5095,#5096,#5097,#5098,#5099,#5100,#5101,#5102,#5103,#5104,#5105,
#5106,#5107,#5108,#5109,#5110,#5111,#5112,#5113,#5114,#5115,#5116,#5117,
#5118,#5119,#5120,#5121,#5122,#5123,#5124,#5125,#5126,#5127,#5128,#5129,
#5130,#5131,#5132,#5133,#5134,#5135,#5136,#5137,#5138,#5139,#5140,#5141,
#5142,#5143,#5144,#5145,#5146,#5147,#5148,#5149,#5150,#5151,#5152,#5153,
#5154,#5155,#5156,#5157,#5158,#5159,#5160,#5161,#5162,#5163,#5164,#5165,
#5166,#5167,#5168,#5169,#5170,#5171,#5172,#5173,#5174,#5175,#5176,#5177,
#5178,#5179,#5180,#5181,#5182,#5183,#5184,#5185,#5186,#5187,#5188,#5189,
#5190,#5191,#5192,#5193,#5194,#5195,#5196,#5197,#5198,#5199,#5200,#5201,
#5202,#5203,#5204,#5205),.UNSPECIFIED.,.F.,.F.,(4,3,3,3,3,3,3,3,3,3,3,3,
3,3,3,3,3,3,3,3,3,3,3,3,3,3,3,3,3,3,3,3,3,3,3,3,3,3,3,3,3,3,3,3,3,3,3,4),
(53.4070751113264,53.5154608823167,53.6249212271248,53.7303453258545,53.8235779004443,
53.9166872770643,54.009700849372,54.1026492469518,54.1955643359709,54.2884707342843,
54.3813930458559,54.474412543289,54.5674848923327,54.6607043142074,54.7176412514196,
54.8108646662176,54.903965072386,54.9969698728911,55.0899098282812,55.1828166815042,
55.2757150592943,55.3686295746718,55.4616416636342,55.5547068117602,55.6479194305051,
55.7049371769848,55.7980868069411,55.8911130729797,55.9840434820572,56.076908981525,
56.1697413679859,56.2625653599032,56.3554056621105,56.448344254422,56.5413362031023,
56.6344768169055,56.6922331025499,56.7855972844833,56.8788375378924,56.9744559017533,
57.0675295291053,57.1605689969723,57.2535987650433,57.3511451859774,57.4442771053405,
57.537462070741,57.630767641988,57.6437844487799),.UNSPECIFIED.);
#70=B_SPLINE_CURVE_WITH_KNOTS('',3,(#5206,#5207,#5208,#5209,#5210,#5211,
#5212,#5213,#5214,#5215,#5216,#5217,#5218,#5219,#5220,#5221,#5222,#5223,
#5224,#5225,#5226,#5227,#5228,#5229,#5230,#5231,#5232,#5233,#5234,#5235,
#5236,#5237,#5238,#5239,#5240,#5241,#5242,#5243,#5244,#5245,#5246,#5247,
#5248,#5249,#5250,#5251,#5252,#5253,#5254,#5255,#5256,#5257,#5258,#5259,
#5260,#5261,#5262,#5263),.UNSPECIFIED.,.F.,.F.,(4,2,2,2,2,2,2,2,2,2,2,2,
2,2,2,2,2,2,2,2,2,2,2,2,2,2,2,2,4),(-4.06067588059912,-4.04069247019934,
-4.02617376395736,-4.01534753129665,-4.00544410492176,-3.99444491625099,
-3.97788641249948,-3.90579227222274,-3.87542989373594,-3.86238290113527,
-3.85199059780189,-3.84565758040844,-3.83917673322251,-3.82807514836664,
-3.77232653875084,-3.71201227279839,-3.69636762635081,-3.68552511088964,
-3.6756519977026,-3.65929508343662,-3.58751727900746,-3.55670727552532,
-3.54354924171794,-3.53309014022462,-3.52674073670713,-3.52027266087198,
-3.50923391192641,-3.45227204802997,-3.39931823127231),.UNSPECIFIED.);
#71=B_SPLINE_CURVE_WITH_KNOTS('',3,(#5265,#5266,#5267,#5268,#5269,#5270,
#5271,#5272,#5273,#5274,#5275,#5276,#5277,#5278,#5279,#5280,#5281,#5282,
#5283,#5284,#5285,#5286,#5287,#5288,#5289,#5290,#5291,#5292,#5293,#5294,
#5295,#5296,#5297,#5298,#5299,#5300,#5301,#5302,#5303,#5304,#5305,#5306,
#5307,#5308,#5309,#5310,#5311,#5312,#5313,#5314,#5315,#5316,#5317,#5318,
#5319,#5320,#5321,#5322,#5323,#5324,#5325,#5326,#5327,#5328,#5329,#5330,
#5331),.UNSPECIFIED.,.F.,.F.,(4,3,3,3,3,3,3,3,3,3,3,3,3,3,3,3,3,3,3,3,3,
3,4),(51.3612711115601,51.4542197461849,51.5471285042568,51.6400220262204,
51.7329249334203,51.8259215363716,51.9189651439704,52.0121635352636,52.0943471759255,
52.1875666611415,52.2806629858775,52.3736635608775,52.4665990957627,52.559501410222,
52.6523951374807,52.7453048969597,52.8383120997537,52.9313722815292,53.0245798571289,
53.0816431014906,53.1910683080732,53.299486149192,53.4070751107236),
 .UNSPECIFIED.);
#72=B_SPLINE_CURVE_WITH_KNOTS('',3,(#5332,#5333,#5334,#5335,#5336,#5337,
#5338,#5339,#5340,#5341,#5342,#5343,#5344,#5345,#5346,#5347,#5348,#5349,
#5350,#5351,#5352,#5353,#5354,#5355,#5356,#5357,#5358,#5359,#5360,#5361,
#5362,#5363,#5364,#5365,#5366,#5367,#5368,#5369,#5370,#5371,#5372,#5373,
#5374,#5375,#5376,#5377,#5378,#5379,#5380,#5381,#5382,#5383,#5384,#5385,
#5386,#5387,#5388,#5389,#5390,#5391,#5392,#5393,#5394,#5395,#5396,#5397,
#5398,#5399,#5400,#5401,#5402,#5403,#5404,#5405,#5406,#5407,#5408,#5409,
#5410,#5411,#5412,#5413,#5414,#5415,#5416,#5417,#5418,#5419,#5420,#5421,
#5422,#5423,#5424,#5425,#5426,#5427,#5428,#5429,#5430,#5431,#5432,#5433,
#5434,#5435,#5436,#5437,#5438,#5439,#5440,#5441,#5442,#5443,#5444,#5445,
#5446,#5447,#5448,#5449,#5450,#5451,#5452,#5453,#5454,#5455),
 .UNSPECIFIED.,.F.,.F.,(4,2,2,2,2,2,2,2,2,2,2,2,2,2,2,2,2,2,2,2,2,2,2,2,
2,2,2,2,2,2,2,2,2,2,2,2,2,2,2,2,2,2,2,2,2,2,2,2,2,2,2,2,2,2,2,2,2,2,2,2,
2,4),(1.36958410658186,1.3918117919107,1.40402272121196,1.41456715400893,
1.42790276929566,1.4580462745132,1.50752852260155,1.54885081199774,1.56042948267245,
1.56701194542835,1.57327886096385,1.58331693394143,1.59576779742258,1.62376905121261,
1.70186095396046,1.71732178254663,1.72802773397601,1.73925394769026,1.75700207751367,
1.77867870716166,1.83228882631052,1.87132868801542,1.88102350568051,1.8866132536601,
1.89307842287806,1.90408956688519,1.91819266087862,1.95306614410452,2.01704247204898,
2.03424075566318,2.04536832594078,2.056279055785,2.0722830490121,2.09109201382839,
2.13125112005048,2.18749585070491,2.19857739702684,2.20505780450936,2.2114061390268,
2.22184804390554,2.23497519938454,2.26565242660347,2.33768752688447,2.35401187972869,
2.36388413422627,2.37474048669759,2.39043682060175,2.40875581975962,2.44698783953403,
2.50699268527341,2.51773193949008,2.52414078926535,2.5305531787131,2.54131076559637,
2.58832711885829,2.65531565789145,2.67222863836378,2.68330135424359,2.69323641474989,
2.70400871752801,2.71841062714054,2.73813407747398),.UNSPECIFIED.);
#73=B_SPLINE_CURVE_WITH_KNOTS('',3,(#5463,#5464,#5465,#5466,#5467),
 .UNSPECIFIED.,.F.,.F.,(4,1,4),(0.,0.98729592556514,1.11004521091133),
 .UNSPECIFIED.);
#74=B_SPLINE_CURVE_WITH_KNOTS('',3,(#5469,#5470,#5471,#5472,#5473,#5474,
#5475,#5476,#5477,#5478,#5479,#5480,#5481,#5482,#5483,#5484,#5485,#5486,
#5487,#5488,#5489,#5490,#5491,#5492,#5493,#5494,#5495,#5496,#5497,#5498,
#5499,#5500,#5501,#5502,#5503,#5504,#5505,#5506,#5507,#5508,#5509,#5510,
#5511,#5512,#5513,#5514,#5515,#5516,#5517,#5518,#5519,#5520,#5521,#5522,
#5523,#5524,#5525,#5526,#5527,#5528,#5529,#5530,#5531,#5532,#5533,#5534,
#5535,#5536,#5537,#5538,#5539,#5540,#5541,#5542,#5543,#5544,#5545,#5546,
#5547,#5548,#5549,#5550,#5551,#5552,#5553,#5554,#5555,#5556,#5557,#5558,
#5559,#5560,#5561,#5562,#5563,#5564,#5565,#5566,#5567,#5568,#5569,#5570,
#5571,#5572,#5573,#5574,#5575,#5576,#5577,#5578,#5579,#5580,#5581,#5582,
#5583,#5584,#5585,#5586,#5587,#5588,#5589,#5590,#5591,#5592,#5593,#5594,
#5595,#5596,#5597,#5598,#5599,#5600,#5601,#5602,#5603,#5604,#5605,#5606,
#5607,#5608,#5609,#5610,#5611,#5612,#5613,#5614,#5615,#5616,#5617,#5618,
#5619,#5620,#5621,#5622,#5623,#5624,#5625,#5626,#5627,#5628,#5629,#5630,
#5631,#5632,#5633,#5634,#5635,#5636,#5637,#5638,#5639,#5640,#5641,#5642,
#5643,#5644,#5645,#5646,#5647,#5648,#5649,#5650,#5651,#5652,#5653,#5654,
#5655,#5656,#5657,#5658,#5659,#5660,#5661,#5662,#5663,#5664,#5665,#5666,
#5667,#5668,#5669,#5670,#5671,#5672,#5673,#5674,#5675,#5676,#5677,#5678,
#5679,#5680,#5681,#5682,#5683,#5684,#5685),.UNSPECIFIED.,.F.,.F.,(4,3,3,
3,3,3,3,3,3,3,3,3,3,3,3,3,3,3,3,3,3,3,3,3,3,3,3,3,3,3,3,3,3,3,3,3,3,3,3,
3,3,3,3,3,3,3,3,3,3,3,3,3,3,3,3,3,3,3,3,3,3,3,3,3,3,3,3,3,3,3,3,3,4),(1.11004521091133,
1.19701335709339,1.28388235776292,1.37067611049039,1.45742933866679,1.54416470100031,
1.63090483587999,1.71772660085398,1.80458826523957,1.89159097544962,1.97459185113028,
2.06327101673013,2.15183613894509,2.24031086414059,2.33050797820994,2.41888072738085,
2.50723956600992,2.59560572419145,2.68717623731744,2.77566875995805,2.86877826832673,
2.96188777669542,3.05070298067973,3.13940823562147,3.22802697630534,3.31817156704974,
3.40669695771299,3.49521138256791,3.58373589624672,3.67509784775018,3.763754169158,
3.85646893570928,3.94918370226056,4.03781192249501,4.12632726936861,4.21475343818185,
4.30496921188733,4.39329671388509,4.48161161804857,4.56993520231051,4.66157130868931,
4.75002503908855,4.83853951085294,4.92717738846736,4.9364796278257,5.02517599892575,
5.11376021655063,5.20225588477605,5.2924458433529,5.38084394577703,5.46922973586957,
5.55762441245108,5.64916219768602,5.73768688045483,5.83073121692283,5.92377555339084,
6.0124783260962,6.10106922151394,6.18957183388173,6.27975928951601,6.36816495208386,
6.45655851974142,6.54496118346079,6.63648875733459,6.72502188060573,6.81804667978086,
6.91107147895598,7.00469257042698,7.10182705728842,7.19504650274243,7.28812775330745,
7.38103834802377,7.39323051787274),.UNSPECIFIED.);
#75=B_SPLINE_CURVE_WITH_KNOTS('',3,(#5687,#5688,#5689,#5690,#5691,#5692,
#5693,#5694,#5695,#5696,#5697,#5698,#5699,#5700,#5701,#5702,#5703,#5704,
#5705,#5706,#5707,#5708,#5709,#5710,#5711,#5712,#5713,#5714,#5715,#5716,
#5717,#5718,#5719,#5720,#5721,#5722,#5723,#5724,#5725,#5726,#5727,#5728,
#5729,#5730,#5731,#5732,#5733,#5734,#5735,#5736,#5737,#5738,#5739,#5740,
#5741,#5742,#5743,#5744,#5745,#5746,#5747,#5748,#5749,#5750,#5751,#5752,
#5753,#5754,#5755,#5756,#5757,#5758,#5759,#5760,#5761,#5762,#5763,#5764,
#5765,#5766,#5767,#5768,#5769,#5770,#5771,#5772,#5773,#5774,#5775,#5776,
#5777,#5778,#5779,#5780,#5781,#5782,#5783,#5784,#5785,#5786,#5787,#5788,
#5789,#5790,#5791,#5792,#5793,#5794,#5795,#5796,#5797,#5798,#5799,#5800,
#5801,#5802,#5803,#5804,#5805,#5806,#5807,#5808,#5809,#5810,#5811,#5812,
#5813,#5814,#5815,#5816,#5817,#5818,#5819,#5820,#5821,#5822,#5823,#5824,
#5825,#5826,#5827,#5828,#5829,#5830,#5831,#5832,#5833,#5834,#5835,#5836,
#5837,#5838,#5839,#5840,#5841,#5842,#5843,#5844,#5845,#5846,#5847,#5848,
#5849,#5850,#5851,#5852,#5853,#5854,#5855,#5856,#5857,#5858,#5859,#5860,
#5861,#5862,#5863,#5864,#5865,#5866,#5867,#5868,#5869,#5870,#5871,#5872,
#5873,#5874,#5875,#5876,#5877,#5878,#5879,#5880,#5881,#5882,#5883,#5884,
#5885,#5886,#5887,#5888,#5889,#5890,#5891,#5892,#5893,#5894,#5895,#5896,
#5897,#5898,#5899,#5900),.UNSPECIFIED.,.F.,.F.,(4,3,3,3,3,3,3,3,3,3,3,3,
3,3,3,3,3,3,3,3,3,3,3,3,3,3,3,3,3,3,3,3,3,3,3,3,3,3,3,3,3,3,3,3,3,3,3,3,
3,3,3,3,3,3,3,3,3,3,3,3,3,3,3,3,3,3,3,3,3,3,3,4),(7.39323051809092,7.48529307319253,
7.57746426680113,7.66983555106452,7.76231599136604,7.85499249188307,7.89836740452112,
7.9870599121303,8.07564033387518,8.1641322784918,8.25432365994111,8.34271824396276,
8.43110059916474,8.51949192877706,8.61103477910436,8.699556367841,8.79260984896363,
8.88566333008626,8.97435570299709,9.06293600738605,9.15142785206477,9.2416192775131,
9.33001380561846,9.41839612152961,9.50678742860532,9.59833038536684,9.68685199398323,
9.77990562481732,9.8729592556514,9.96164991525048,10.0502284761189,10.1387185494565,
10.2289106284265,10.3173033279091,10.405683797039,10.4940732412073,10.5856187262096,
10.6741384486948,10.7671968149556,10.8602551812165,10.9489467575841,11.0375262470332,
11.1260172595102,11.2162089904191,11.304602648982,11.3929840829243,11.4813744965563,
11.5729186491126,11.6614393437252,11.7544952252534,11.8475511067817,11.9362425867459,
12.0248219803444,12.1133128976455,12.2035046644832,12.2918982301909,12.3802795723187,
12.4686698952878,12.5602141795525,12.6487347872506,12.7417909097987,12.8348470323468,
12.9222626009469,13.0095667024862,13.0967750381868,13.1839306454997,13.2710559453825,
13.3581733274571,13.4453456514344,13.5325468425587,13.6198538539382,13.6764158250785),
 .UNSPECIFIED.);
#76=B_SPLINE_CURVE_WITH_KNOTS('',3,(#5902,#5903,#5904,#5905,#5906,#5907,
#5908,#5909,#5910,#5911,#5912,#5913,#5914,#5915,#5916,#5917,#5918,#5919,
#5920,#5921,#5922,#5923,#5924,#5925,#5926,#5927,#5928,#5929,#5930,#5931,
#5932,#5933,#5934,#5935,#5936,#5937,#5938,#5939,#5940,#5941,#5942,#5943,
#5944,#5945,#5946,#5947,#5948,#5949,#5950,#5951,#5952,#5953,#5954,#5955,
#5956,#5957,#5958,#5959,#5960,#5961,#5962,#5963,#5964,#5965,#5966,#5967,
#5968,#5969,#5970,#5971,#5972,#5973,#5974,#5975,#5976,#5977,#5978,#5979,
#5980,#5981,#5982,#5983,#5984,#5985,#5986,#5987,#5988,#5989,#5990,#5991,
#5992,#5993,#5994,#5995,#5996,#5997,#5998,#5999,#6000,#6001,#6002,#6003,
#6004,#6005,#6006,#6007,#6008,#6009,#6010,#6011,#6012,#6013,#6014,#6015,
#6016,#6017,#6018,#6019,#6020,#6021,#6022,#6023,#6024,#6025,#6026,#6027,
#6028,#6029,#6030,#6031,#6032,#6033,#6034,#6035,#6036,#6037,#6038,#6039,
#6040,#6041,#6042,#6043,#6044,#6045,#6046,#6047,#6048,#6049,#6050,#6051,
#6052,#6053,#6054,#6055,#6056,#6057,#6058,#6059,#6060,#6061,#6062,#6063,
#6064,#6065,#6066,#6067,#6068,#6069,#6070,#6071,#6072,#6073,#6074,#6075,
#6076,#6077,#6078,#6079,#6080,#6081,#6082,#6083,#6084,#6085,#6086,#6087,
#6088,#6089,#6090,#6091,#6092,#6093,#6094,#6095,#6096,#6097,#6098,#6099,
#6100,#6101,#6102,#6103,#6104,#6105,#6106,#6107,#6108,#6109),
 .UNSPECIFIED.,.F.,.F.,(4,3,3,3,3,3,3,3,3,3,3,3,3,3,3,3,3,3,3,3,3,3,3,3,
3,3,3,3,3,3,3,3,3,3,3,3,3,3,3,3,3,3,3,3,3,3,3,3,3,3,3,3,3,3,3,3,3,3,3,3,
3,3,3,3,3,3,3,3,3,4),(13.6764158252705,13.822142957912,13.910834385622,
13.9994137254484,14.087904587536,14.1780963745286,14.2664898818076,14.3548711644067,
14.4432614268103,14.534805790977,14.6233263360623,14.7163826097697,14.8094388834771,
14.8981302929591,14.9867096144838,15.0752004582202,15.1653922520729,15.2537857410009,
15.3421670052827,15.4305572494239,15.5221016393285,15.6106221664602,15.7036784877512,
15.7967348090422,15.8854262058353,15.9740055144055,16.0624963449394,16.1526881436479,
16.2410816188459,16.3294628692249,16.4178530993054,16.5093975081309,16.5979180209356,
16.6909743777715,16.7840307346074,16.872722141994,16.9613014613115,17.049792302732,
17.139984097412,17.2283775837697,17.3167588453903,17.4051490867822,17.4966934801298,
17.5852140043155,17.678270332244,17.7713266601725,17.8600180648758,17.948597381489,
18.0370882201877,18.1272800158815,18.2156734994925,18.3040547583622,18.3924449970019,
18.4839893941859,18.5725099156422,18.6655662506899,18.7586225857377,18.8473139894916,
18.9358933051323,19.0243841428369,19.1145759388951,19.2029694214646,19.2913506792768,
19.3797409168442,19.4712853154589,19.5598058358158,19.6528621735593,19.7459185113028,
19.8669494233805,19.9596011324501),.UNSPECIFIED.);
#77=B_SPLINE_CURVE_WITH_KNOTS('',3,(#6111,#6112,#6113,#6114,#6115,#6116,
#6117,#6118,#6119,#6120,#6121,#6122,#6123,#6124,#6125,#6126,#6127,#6128,
#6129,#6130,#6131,#6132,#6133,#6134,#6135,#6136,#6137,#6138,#6139,#6140,
#6141,#6142,#6143,#6144,#6145,#6146,#6147,#6148,#6149,#6150,#6151,#6152,
#6153,#6154,#6155,#6156,#6157,#6158,#6159,#6160,#6161,#6162,#6163,#6164,
#6165,#6166,#6167,#6168,#6169,#6170,#6171,#6172,#6173,#6174,#6175,#6176,
#6177,#6178,#6179,#6180,#6181,#6182,#6183,#6184,#6185,#6186,#6187,#6188,
#6189,#6190,#6191,#6192,#6193,#6194,#6195,#6196,#6197,#6198,#6199,#6200,
#6201,#6202,#6203,#6204,#6205,#6206,#6207,#6208,#6209,#6210,#6211,#6212,
#6213,#6214,#6215,#6216,#6217,#6218,#6219,#6220,#6221,#6222,#6223,#6224,
#6225,#6226,#6227,#6228,#6229,#6230,#6231,#6232,#6233,#6234,#6235,#6236,
#6237,#6238,#6239,#6240,#6241,#6242,#6243,#6244,#6245,#6246,#6247,#6248,
#6249,#6250,#6251,#6252,#6253,#6254,#6255,#6256,#6257,#6258,#6259,#6260,
#6261,#6262,#6263,#6264,#6265,#6266,#6267,#6268,#6269,#6270,#6271,#6272,
#6273,#6274,#6275,#6276,#6277,#6278,#6279,#6280,#6281,#6282,#6283,#6284,
#6285,#6286,#6287,#6288,#6289,#6290,#6291,#6292,#6293,#6294,#6295,#6296,
#6297,#6298,#6299,#6300,#6301,#6302,#6303,#6304,#6305,#6306,#6307,#6308,
#6309,#6310,#6311,#6312,#6313,#6314,#6315,#6316,#6317,#6318,#6319,#6320,
#6321,#6322,#6323,#6324),.UNSPECIFIED.,.F.,.F.,(4,3,3,3,3,3,3,3,3,3,3,3,
3,3,3,3,3,3,3,3,3,3,3,3,3,3,3,3,3,3,3,3,3,3,3,3,3,3,3,3,3,3,3,3,3,3,3,3,
3,3,3,3,3,3,3,3,3,3,3,3,3,3,3,3,3,3,3,3,3,3,3,4),(19.9596011326718,20.0469237800727,
20.1341771968951,20.2213938721846,20.3085961433456,20.3958063314767,20.4830999449737,
20.570435755381,20.6579098238915,20.7332144368679,20.8219058413541,20.9104851577402,
20.9989759962022,21.0891677919811,21.1775612753329,21.2659425339355,21.3543327723005,
21.4458771698336,21.5343976909983,21.6274540267157,21.7205103624331,21.809201766862,
21.8977810831887,21.9862719215897,22.0764637173908,22.1648572006777,22.253238459214,
22.3416286975111,22.4331730951328,22.5216936162272,22.6147499521127,22.7078062879982,
22.7964976925349,22.8850770089713,22.9735678474835,23.0637596432435,23.1521531266447,
23.2405343852962,23.3289246237095,23.4204690211729,23.5089895423846,23.602045877974,
23.6951022135634,23.7837936180562,23.8723729344482,23.9608637729156,24.0510555686922,
24.1394490520478,24.2278303106535,24.316220549021,24.4077649465478,24.4962854677135,
24.589341803421,24.6823981391285,24.7710895436196,24.8596688600099,24.9481596984755,
25.0383514942527,25.126744977606,25.2151262362092,25.3035164745745,25.3950608721043,
25.4835813932671,25.5766377289804,25.6696940646936,25.7601596923641,25.8504978540204,
25.9407269674771,26.0308459404358,26.1209002292553,26.2109023846584,26.2427864396297),
 .UNSPECIFIED.);
#78=B_SPLINE_CURVE_WITH_KNOTS('',3,(#6326,#6327,#6328,#6329,#6330,#6331,
#6332,#6333,#6334,#6335,#6336,#6337,#6338,#6339,#6340,#6341,#6342,#6343,
#6344,#6345,#6346,#6347,#6348,#6349,#6350,#6351,#6352,#6353,#6354,#6355,
#6356,#6357,#6358,#6359,#6360,#6361,#6362,#6363,#6364,#6365,#6366,#6367,
#6368,#6369,#6370,#6371,#6372,#6373,#6374,#6375,#6376,#6377,#6378,#6379,
#6380,#6381,#6382,#6383,#6384,#6385,#6386,#6387,#6388,#6389,#6390,#6391,
#6392,#6393,#6394,#6395,#6396,#6397,#6398,#6399,#6400,#6401,#6402,#6403,
#6404,#6405,#6406,#6407,#6408,#6409,#6410,#6411,#6412,#6413,#6414,#6415,
#6416,#6417,#6418,#6419,#6420,#6421,#6422,#6423,#6424,#6425,#6426,#6427,
#6428,#6429,#6430,#6431,#6432,#6433,#6434,#6435,#6436,#6437,#6438,#6439,
#6440,#6441,#6442,#6443,#6444,#6445,#6446,#6447,#6448,#6449,#6450,#6451,
#6452,#6453,#6454,#6455,#6456,#6457,#6458,#6459,#6460,#6461,#6462,#6463,
#6464,#6465,#6466,#6467,#6468,#6469,#6470,#6471,#6472,#6473,#6474,#6475,
#6476,#6477,#6478,#6479,#6480,#6481,#6482,#6483,#6484,#6485,#6486,#6487,
#6488,#6489,#6490,#6491,#6492,#6493,#6494,#6495,#6496,#6497,#6498,#6499,
#6500,#6501,#6502,#6503,#6504,#6505,#6506,#6507,#6508,#6509,#6510,#6511,
#6512,#6513,#6514,#6515,#6516,#6517,#6518,#6519,#6520,#6521,#6522,#6523,
#6524,#6525,#6526,#6527,#6528,#6529,#6530,#6531,#6532,#6533,#6534,#6535,
#6536,#6537,#6538,#6539),.UNSPECIFIED.,.F.,.F.,(4,3,3,3,3,3,3,3,3,3,3,3,
3,3,3,3,3,3,3,3,3,3,3,3,3,3,3,3,3,3,3,3,3,3,3,3,3,3,3,3,3,3,3,3,3,3,3,3,
3,3,3,3,3,3,3,3,3,3,3,3,3,3,3,3,3,3,3,3,3,3,3,4),(26.242786439791,26.3389678131502,
26.4355814021047,26.5324211410047,26.6295674855356,26.6569899902588,26.7456813947491,
26.8342607111387,26.9227515496036,27.0129433453811,27.1013368287343,27.1897180873376,
27.2781083257026,27.3696527232329,27.4581732443964,27.5512295801101,27.6442859158239,
27.7329773203172,27.8215566367098,27.9100474751774,28.0002392709539,28.0886327543096,
28.1770140129154,28.2654042512827,28.3569486488093,28.4454691699747,28.5385255056819,
28.6315818413891,28.7202732459279,28.808852562366,28.8973434008794,28.9875351966388,
29.0759286800403,29.1643099386917,29.2527001771046,29.344244574567,29.4327650957773,
29.5258214313657,29.6188777669542,29.7075691713759,29.7961484876969,29.8846393260935,
29.9748311218968,30.0632246051826,30.1516058637191,30.2399961020178,30.3315404996432,
30.4200610207422,30.5131173566308,30.6061736925193,30.6948650970128,30.7834444134047,
30.8719352518711,30.9621270476478,31.0505205310006,31.1389017896029,31.2272920279661,
31.3188364254957,31.4073569466556,31.5004132823701,31.5934696180845,31.6814401592432,
31.7692990613542,31.857070757937,31.9447815725409,32.0324610760959,32.1201312161915,
32.2078139283142,32.29558092047,32.3833936954151,32.4713359381952,32.5259717466392),
 .UNSPECIFIED.);
#79=B_SPLINE_CURVE_WITH_KNOTS('',3,(#6541,#6542,#6543,#6544,#6545,#6546,
#6547,#6548,#6549,#6550,#6551,#6552,#6553,#6554,#6555,#6556,#6557,#6558,
#6559,#6560,#6561,#6562,#6563,#6564,#6565,#6566,#6567,#6568,#6569,#6570,
#6571,#6572,#6573,#6574,#6575,#6576,#6577,#6578,#6579,#6580,#6581,#6582,
#6583,#6584,#6585,#6586,#6587,#6588,#6589,#6590,#6591,#6592,#6593,#6594,
#6595,#6596,#6597,#6598,#6599,#6600,#6601,#6602,#6603,#6604,#6605,#6606,
#6607,#6608,#6609,#6610,#6611,#6612,#6613,#6614,#6615,#6616,#6617,#6618,
#6619,#6620,#6621,#6622,#6623,#6624,#6625,#6626,#6627,#6628,#6629,#6630,
#6631,#6632,#6633,#6634,#6635,#6636,#6637,#6638,#6639,#6640,#6641,#6642,
#6643,#6644,#6645,#6646,#6647,#6648,#6649,#6650,#6651,#6652,#6653,#6654,
#6655,#6656,#6657,#6658,#6659,#6660,#6661,#6662,#6663,#6664,#6665,#6666,
#6667,#6668,#6669,#6670,#6671,#6672,#6673,#6674,#6675,#6676,#6677,#6678,
#6679,#6680,#6681,#6682,#6683,#6684,#6685,#6686,#6687,#6688,#6689,#6690,
#6691,#6692,#6693,#6694,#6695,#6696,#6697,#6698,#6699,#6700,#6701,#6702,
#6703,#6704,#6705,#6706,#6707,#6708,#6709,#6710,#6711,#6712,#6713,#6714,
#6715,#6716,#6717,#6718,#6719,#6720,#6721,#6722,#6723,#6724,#6725,#6726,
#6727,#6728,#6729,#6730,#6731,#6732,#6733,#6734,#6735,#6736,#6737,#6738,
#6739,#6740,#6741,#6742,#6743,#6744,#6745,#6746,#6747,#6748,#6749,#6750,
#6751),.UNSPECIFIED.,.F.,.F.,(4,3,3,3,3,3,3,3,3,3,3,3,3,3,3,3,3,3,3,3,3,
3,3,3,3,3,3,3,3,3,3,3,3,3,3,3,3,3,3,3,3,3,3,3,3,3,3,3,3,3,3,3,3,3,3,3,3,
3,3,3,3,3,3,3,3,3,3,3,3,3,4),(32.5259717468093,32.5807655436496,32.6694569473346,
32.7580362629197,32.8465271005819,32.936718896661,33.0251123792211,33.1134936370362,
33.2018838746188,33.2934282732678,33.3819487936705,33.4750051314427,33.5680614692148,
33.6567528740102,33.7453321906977,33.833823029453,33.9240148251188,34.0124083087424,
34.1007895676081,34.1891798062273,34.2807242033654,34.3692447247604,34.4623010597702,
34.5553573947799,34.6440488022623,34.7326281216572,34.8211189631364,34.9113107577875,
34.9997042441582,35.0880855057747,35.1764757471452,35.2680201404452,35.3565406645672,
35.4495969924561,35.542653320345,35.6313447164961,35.7199240245483,35.8084148546879,
35.8986066535907,35.9870001287016,36.0753813791082,36.163771609331,36.2553160184758,
36.3438365317079,36.436892888809,36.5299492459102,36.618640656464,36.7072199788533,
36.7957108232477,36.8859026167761,36.9742961058495,37.0626773700851,37.1510676139887,
37.2426120033603,37.3311325297788,37.424188850627,37.5172451714753,37.6059365995803,
37.6945159397253,37.7830068020554,37.8731985889285,37.9615920962611,38.0499733788434,
38.1383636411596,38.2299080051299,38.3184285499525,38.4114848234965,38.5045410970405,
38.6109616044168,38.7162352571934,38.8091570538353),.UNSPECIFIED.);
#80=B_SPLINE_CURVE_WITH_KNOTS('',3,(#6753,#6754,#6755,#6756,#6757,#6758,
#6759,#6760,#6761,#6762,#6763,#6764,#6765,#6766,#6767,#6768,#6769,#6770,
#6771,#6772,#6773,#6774,#6775,#6776,#6777,#6778,#6779,#6780,#6781,#6782,
#6783,#6784,#6785,#6786,#6787,#6788,#6789,#6790,#6791,#6792,#6793,#6794,
#6795,#6796,#6797,#6798,#6799,#6800,#6801,#6802,#6803,#6804,#6805,#6806,
#6807,#6808,#6809,#6810,#6811,#6812,#6813,#6814,#6815,#6816,#6817,#6818,
#6819,#6820,#6821,#6822,#6823,#6824,#6825,#6826,#6827,#6828,#6829,#6830,
#6831,#6832,#6833,#6834,#6835,#6836,#6837,#6838,#6839,#6840,#6841,#6842,
#6843,#6844,#6845,#6846,#6847,#6848,#6849,#6850,#6851,#6852,#6853,#6854,
#6855,#6856,#6857,#6858,#6859,#6860,#6861,#6862,#6863,#6864,#6865,#6866,
#6867,#6868,#6869,#6870,#6871,#6872,#6873,#6874,#6875,#6876,#6877,#6878,
#6879,#6880,#6881,#6882,#6883,#6884,#6885,#6886,#6887,#6888,#6889,#6890,
#6891,#6892,#6893,#6894,#6895,#6896,#6897,#6898,#6899,#6900,#6901,#6902,
#6903,#6904,#6905,#6906,#6907,#6908,#6909,#6910,#6911,#6912,#6913,#6914,
#6915,#6916,#6917,#6918,#6919,#6920,#6921,#6922,#6923,#6924,#6925,#6926,
#6927,#6928,#6929,#6930,#6931,#6932,#6933,#6934,#6935,#6936,#6937,#6938,
#6939,#6940,#6941,#6942,#6943,#6944,#6945,#6946,#6947,#6948,#6949,#6950,
#6951,#6952,#6953,#6954,#6955,#6956,#6957,#6958,#6959,#6960,#6961,#6962,
#6963,#6964,#6965,#6966),.UNSPECIFIED.,.F.,.F.,(4,3,3,3,3,3,3,3,3,3,3,3,
3,3,3,3,3,3,3,3,3,3,3,3,3,3,3,3,3,3,3,3,3,3,3,3,3,3,3,3,3,3,3,3,3,3,3,3,
3,3,3,3,3,3,3,3,3,3,3,3,3,3,3,3,3,3,3,3,3,3,3,4),(38.8091570539888,38.8971609962568,
38.9851394954773,39.0731141630393,39.1611066024483,39.2491930905398,39.3373291738814,
39.4256069554307,39.4918370226056,39.580528514339,39.6691079174307,39.7575988419588,
39.8477906052353,39.9361841725392,40.0245655141604,40.1129558345204,40.2045001129329,
40.2930207127995,40.3860768304851,40.4791329481707,40.5678245231247,40.6564040114336,
40.7448950230426,40.8350867543793,40.9234804127504,41.0118618467536,41.1002522606992,
41.1917964139584,41.2803171095116,41.3733729916237,41.4664288737359,41.5551194833438,
41.6436980038881,41.7321880465287,41.8223801406253,41.9107728333273,41.9991533046095,
42.0875427598615,42.1790882697214,42.2676080254717,42.3606664123863,42.453724799301,
42.5424172958676,42.6309977000003,42.7194896206085,42.8096810086407,42.8980755535172,
42.9864578641023,43.074849143759,43.1663920390358,43.2549135653677,43.347967145117,
43.4410207248662,43.529713168881,43.6182935393289,43.7067854448956,43.7969768455876,
43.8853714209839,43.973753778925,44.062145122639,44.1536880045871,44.2422096356415,
44.3352631430364,44.4283166504313,44.5168547259066,44.6052841782716,44.6936265092543,
44.7819031478381,44.870142582569,44.9583597887507,45.0465968796254,45.0923423611684),
 .UNSPECIFIED.);
#81=B_SPLINE_CURVE_WITH_KNOTS('',3,(#6968,#6969,#6970,#6971,#6972,#6973,
#6974,#6975,#6976,#6977,#6978,#6979,#6980,#6981,#6982,#6983,#6984,#6985,
#6986,#6987,#6988,#6989,#6990,#6991,#6992,#6993,#6994,#6995,#6996,#6997,
#6998,#6999,#7000,#7001,#7002,#7003,#7004,#7005,#7006,#7007,#7008,#7009,
#7010,#7011,#7012,#7013,#7014,#7015,#7016,#7017,#7018,#7019,#7020,#7021,
#7022,#7023,#7024,#7025,#7026,#7027,#7028,#7029,#7030,#7031,#7032,#7033,
#7034,#7035,#7036,#7037,#7038,#7039,#7040,#7041,#7042,#7043,#7044,#7045,
#7046,#7047,#7048,#7049,#7050,#7051,#7052,#7053,#7054,#7055,#7056,#7057,
#7058,#7059,#7060,#7061,#7062,#7063,#7064,#7065,#7066,#7067,#7068,#7069,
#7070,#7071,#7072,#7073,#7074,#7075,#7076,#7077,#7078,#7079,#7080,#7081,
#7082,#7083,#7084,#7085,#7086,#7087,#7088,#7089,#7090,#7091,#7092,#7093,
#7094,#7095,#7096,#7097,#7098,#7099,#7100,#7101,#7102,#7103,#7104,#7105,
#7106,#7107,#7108,#7109,#7110,#7111,#7112,#7113,#7114,#7115,#7116,#7117,
#7118,#7119,#7120,#7121,#7122,#7123,#7124,#7125,#7126,#7127,#7128,#7129,
#7130,#7131,#7132,#7133,#7134,#7135,#7136,#7137,#7138,#7139,#7140,#7141,
#7142,#7143,#7144,#7145,#7146,#7147,#7148),.UNSPECIFIED.,.F.,.F.,(4,3,3,
3,3,3,3,3,3,3,3,3,3,3,3,3,3,3,3,3,3,3,3,3,3,3,3,3,3,3,3,3,3,3,3,3,3,3,3,
3,3,3,3,3,3,3,3,3,3,3,3,3,3,3,3,3,3,3,3,3,4),(45.0923423613472,45.1954635567779,
45.2992248310576,45.4036717304518,45.4156125759964,45.5043166047354,45.5929085132717,
45.6814118968335,45.7715989724245,45.8600048052718,45.9483983187276,46.0368007038082,
46.1283276532466,46.216859940611,46.3098842210863,46.4029085015616,46.4916038154234,
46.5801871802618,46.6686821993189,46.7588724777948,46.8472704368479,46.9356562725042,
47.0240511835473,47.1155894944421,47.2041148807565,47.2971596539416,47.3902044271267,
47.4788295400663,47.5673423800983,47.6557666400549,47.7459833541346,47.8343104336168,
47.9226254701026,48.0109497414159,48.1025873942349,48.1910431907813,48.2795602065755,
48.3682012831507,48.3775003526918,48.4663274941079,48.5550423748666,48.6436684390571,
48.7338094189571,48.8223364205068,48.910850319811,48.9993721719169,49.0907281985019,
49.1793765648354,49.2720864215462,49.364796278257,49.4524061344098,49.5399061070432,
49.6305462355617,49.7179014996095,49.8052286593192,49.8925499496824,49.9798875964482,
50.0673084984293,50.154779220223,50.2423674345182,50.2650271351914),
 .UNSPECIFIED.);
#82=B_SPLINE_CURVE_WITH_KNOTS('',3,(#7152,#7153,#7154,#7155,#7156,#7157,
#7158,#7159),.UNSPECIFIED.,.F.,.F.,(4,1,1,1,1,4),(-52.3266840549524,-51.3393881293873,
-50.3520922038222,-49.3647962782571,-48.3775003526919,-48.075051328453),
 .UNSPECIFIED.);
#83=B_SPLINE_CURVE_WITH_KNOTS('',3,(#7161,#7162,#7163,#7164,#7165,#7166,
#7167,#7168,#7169,#7170,#7171,#7172,#7173,#7174,#7175,#7176,#7177,#7178,
#7179,#7180,#7181,#7182,#7183,#7184,#7185,#7186,#7187,#7188,#7189,#7190,
#7191,#7192,#7193,#7194,#7195,#7196,#7197,#7198,#7199,#7200,#7201,#7202,
#7203,#7204,#7205,#7206,#7207,#7208,#7209,#7210,#7211,#7212,#7213,#7214,
#7215,#7216,#7217,#7218,#7219,#7220,#7221,#7222,#7223,#7224,#7225,#7226,
#7227,#7228,#7229,#7230,#7231,#7232,#7233,#7234,#7235,#7236,#7237,#7238,
#7239,#7240,#7241,#7242,#7243,#7244,#7245,#7246,#7247,#7248,#7249,#7250,
#7251,#7252,#7253,#7254,#7255,#7256,#7257,#7258,#7259,#7260,#7261,#7262,
#7263,#7264,#7265,#7266,#7267,#7268,#7269,#7270,#7271,#7272,#7273,#7274,
#7275,#7276,#7277,#7278,#7279,#7280,#7281,#7282,#7283,#7284,#7285,#7286,
#7287,#7288,#7289,#7290,#7291,#7292,#7293,#7294,#7295,#7296,#7297,#7298,
#7299,#7300,#7301,#7302,#7303,#7304,#7305,#7306,#7307,#7308,#7309,#7310,
#7311,#7312,#7313,#7314,#7315,#7316,#7317,#7318,#7319,#7320,#7321,#7322,
#7323,#7324,#7325,#7326,#7327,#7328,#7329,#7330,#7331,#7332,#7333,#7334,
#7335,#7336,#7337,#7338,#7339,#7340,#7341,#7342,#7343,#7344,#7345,#7346,
#7347,#7348,#7349,#7350,#7351,#7352,#7353,#7354,#7355,#7356,#7357,#7358,
#7359,#7360,#7361,#7362,#7363,#7364,#7365,#7366,#7367,#7368,#7369,#7370,
#7371,#7372,#7373,#7374),.UNSPECIFIED.,.F.,.F.,(4,3,3,3,3,3,3,3,3,3,3,3,
3,3,3,3,3,3,3,3,3,3,3,3,3,3,3,3,3,3,3,3,3,3,3,3,3,3,3,3,3,3,3,3,3,3,3,3,
3,3,3,3,3,3,3,3,3,3,3,3,3,3,3,3,3,3,3,3,3,3,3,4),(-48.0750461904513,-47.9871108288014,
-47.8992019431481,-47.8112978527581,-47.7233768854568,-47.6353623691097,
-47.5472989379262,-47.4590929505688,-47.3902044271268,-47.3015080469572,
-47.2129238201834,-47.1244281427414,-47.0342381875939,-46.9458400758472,
-46.8574542764087,-46.7690595904687,-46.6775218182419,-46.5889971261679,
-46.4959528138647,-46.4029085015616,-46.3142057267072,-46.2256148290899,
-46.1371122144743,-46.0469247596645,-45.9585190947443,-45.8701255246994,
-45.78172285856,-45.6901952879191,-45.6016621621677,-45.5086373690821,-45.4156125759965,
-45.3269281466859,-45.2383558993655,-45.1498722143147,-45.0596777688293,
-44.9712916005818,-44.8829177044209,-44.7945348676157,-44.7029803133196,
-44.6144672231741,-44.5213919368027,-44.4283166504313,-44.3396241415134,
-44.2510437184474,-44.1625517724985,-44.0723603915444,-43.9839658061715,
-43.8955834496137,-43.8071921186426,-43.7156492701985,-43.6271276801083,
-43.5340742024872,-43.4410207248662,-43.3523283516816,-43.2637480470117,
-43.1752562020449,-43.0850647767019,-42.9966702482929,-42.9082879320725,
-42.819896624683,-42.7283536683375,-42.6398320593977,-42.5467784293494,
-42.4537247993011,-42.3651482619786,-42.2766806281153,-42.1883004393225,
-42.0999863100107,-42.0117102946501,-41.9234568731682,-41.8351849856978,
-41.7918608832717),.UNSPECIFIED.);
#84=B_SPLINE_CURVE_WITH_KNOTS('',3,(#7376,#7377,#7378,#7379,#7380,#7381,
#7382,#7383,#7384,#7385,#7386,#7387,#7388,#7389,#7390,#7391,#7392,#7393,
#7394,#7395,#7396,#7397,#7398,#7399,#7400,#7401,#7402,#7403,#7404,#7405,
#7406,#7407,#7408,#7409,#7410,#7411,#7412,#7413,#7414,#7415,#7416,#7417,
#7418,#7419,#7420,#7421,#7422,#7423,#7424,#7425,#7426,#7427,#7428,#7429,
#7430,#7431,#7432,#7433,#7434,#7435,#7436,#7437,#7438,#7439,#7440,#7441,
#7442,#7443,#7444,#7445,#7446,#7447,#7448,#7449,#7450,#7451,#7452,#7453,
#7454,#7455,#7456,#7457,#7458,#7459,#7460,#7461,#7462,#7463,#7464,#7465,
#7466,#7467,#7468,#7469,#7470,#7471,#7472,#7473,#7474,#7475,#7476,#7477,
#7478,#7479,#7480,#7481,#7482,#7483,#7484,#7485,#7486,#7487,#7488,#7489,
#7490,#7491,#7492,#7493,#7494,#7495,#7496,#7497,#7498,#7499,#7500,#7501,
#7502,#7503,#7504,#7505,#7506,#7507,#7508,#7509,#7510,#7511,#7512,#7513,
#7514,#7515,#7516,#7517,#7518,#7519,#7520,#7521,#7522,#7523,#7524,#7525,
#7526,#7527,#7528,#7529,#7530,#7531,#7532,#7533,#7534,#7535,#7536,#7537,
#7538,#7539,#7540,#7541,#7542,#7543,#7544,#7545,#7546,#7547,#7548,#7549,
#7550,#7551,#7552,#7553,#7554,#7555,#7556,#7557,#7558,#7559,#7560,#7561,
#7562,#7563,#7564,#7565,#7566,#7567,#7568,#7569,#7570,#7571,#7572,#7573,
#7574,#7575,#7576,#7577,#7578,#7579,#7580,#7581,#7582,#7583,#7584,#7585,
#7586,#7587,#7588,#7589),.UNSPECIFIED.,.F.,.F.,(4,3,3,3,3,3,3,3,3,3,3,3,
3,3,3,3,3,3,3,3,3,3,3,3,3,3,3,3,3,3,3,3,3,3,3,3,3,3,3,3,3,3,3,3,3,3,3,3,
3,3,3,3,3,3,3,3,3,3,3,3,3,3,3,3,3,3,3,3,3,3,3,4),(-41.7918608830911,-41.6889257523798,
-41.5853660103364,-41.4811306934174,-41.4664288737359,-41.3777372971778,
-41.2891578075365,-41.2006667948651,-41.1104750640283,-41.0220814052683,
-40.9336999711282,-40.8453095572976,-40.7537654050159,-40.6652447102054,
-40.5721888291881,-40.4791329481708,-40.3904414681829,-40.3018620745599,
-40.2133711572333,-40.1231793904049,-40.0347858246699,-39.9464044825142,
-39.8580141595162,-39.7664698752886,-39.6779492675608,-39.5848931450832,
-39.4918370226056,-39.4031456951822,-39.3145664570197,-39.2260756978358,
-39.1358838727364,-39.0474904707518,-38.959109294152,-38.8707191383343,
-38.7791746280108,-38.6906541899937,-38.5975976435171,-38.5045410970405,
-38.4158496693036,-38.32727032945,-38.2387794673349,-38.1485876803525,-38.0601941730456,
-37.9718128904184,-37.8834226279865,-37.7918782638588,-37.7033577187453,
-37.6103014451104,-37.5172451714754,-37.4285537619925,-37.3399744404667,
-37.2514835967294,-37.161291802877,-37.0728983139477,-36.9845170496646,
-36.896126805522,-36.804582415619,-36.7160618884858,-36.623005567198,-36.5299492459102,
-36.4412578491243,-36.3526785405615,-36.2641877100351,-36.1739959113238,
-36.0856024361335,-35.9972211857622,-35.9088309556895,-35.8172865468534,
-35.7287660340565,-35.6357096772008,-35.5426533203451,-35.5086755760921),
 .UNSPECIFIED.);
#85=B_SPLINE_CURVE_WITH_KNOTS('',3,(#7591,#7592,#7593,#7594,#7595,#7596,
#7597,#7598,#7599,#7600,#7601,#7602,#7603,#7604,#7605,#7606,#7607,#7608,
#7609,#7610,#7611,#7612,#7613,#7614,#7615,#7616,#7617,#7618,#7619,#7620,
#7621,#7622,#7623,#7624,#7625,#7626,#7627,#7628,#7629,#7630,#7631,#7632,
#7633,#7634,#7635,#7636,#7637,#7638,#7639,#7640,#7641,#7642,#7643,#7644,
#7645,#7646,#7647,#7648,#7649,#7650,#7651,#7652,#7653,#7654,#7655,#7656,
#7657,#7658,#7659,#7660,#7661,#7662,#7663,#7664,#7665,#7666,#7667,#7668,
#7669,#7670,#7671,#7672,#7673,#7674,#7675,#7676,#7677,#7678,#7679,#7680,
#7681,#7682,#7683,#7684,#7685,#7686,#7687,#7688,#7689,#7690,#7691,#7692,
#7693,#7694,#7695,#7696,#7697,#7698,#7699,#7700,#7701,#7702,#7703,#7704,
#7705,#7706,#7707,#7708,#7709,#7710,#7711,#7712,#7713,#7714,#7715,#7716,
#7717,#7718,#7719,#7720,#7721,#7722,#7723,#7724,#7725,#7726,#7727,#7728,
#7729,#7730,#7731,#7732,#7733,#7734,#7735,#7736,#7737,#7738,#7739,#7740,
#7741,#7742,#7743,#7744,#7745,#7746,#7747,#7748,#7749,#7750,#7751,#7752,
#7753,#7754,#7755,#7756,#7757,#7758,#7759,#7760,#7761,#7762,#7763,#7764,
#7765,#7766,#7767,#7768,#7769,#7770,#7771,#7772,#7773,#7774,#7775,#7776,
#7777,#7778,#7779,#7780,#7781,#7782,#7783,#7784,#7785,#7786,#7787,#7788,
#7789,#7790,#7791,#7792,#7793,#7794,#7795,#7796,#7797,#7798,#7799,#7800,
#7801),.UNSPECIFIED.,.F.,.F.,(4,3,3,3,3,3,3,3,3,3,3,3,3,3,3,3,3,3,3,3,3,
3,3,3,3,3,3,3,3,3,3,3,3,3,3,3,3,3,3,3,3,3,3,3,3,3,3,3,3,3,3,3,3,3,3,3,3,
3,3,3,3,3,3,3,3,3,3,3,3,3,4),(-35.5086755758622,-35.4204742205616,-35.3323832445334,
-35.2443784702568,-35.1564329342824,-35.0685181555091,-34.9806124069457,
-34.8926939733897,-34.8046873075424,-34.7166353007272,-34.6284436413324,
-34.5553573947799,-34.4666659900769,-34.378086673464,-34.2895958347657,
-34.1994040390718,-34.111010555461,-34.0226292965915,-33.934239057952,-33.8426946607677,
-33.7541741393116,-33.6611178042632,-33.5680614692148,-33.4793700654617,
-33.390790749822,-33.3022999121181,-33.2121081160596,-33.123714633491,-33.0353333756797,
-32.9469431381131,-32.8553987394972,-32.7668782191413,-32.6738218813955,
-32.5807655436497,-32.4920741388114,-32.4034948220695,-32.3150039832488,
-32.2248121876033,-32.1364187038877,-32.04803744492,-31.9596472061894,-31.8681028091632,
-31.7795822876339,-31.6865259528592,-31.5934696180845,-31.5047782135983,
-31.4161988972124,-31.3277080587505,-31.2375162629716,-31.1491227796198,
-31.0607415210174,-30.9723512826528,-30.8808068851194,-30.7922863639549,
-30.6992300282371,-30.6061736925194,-30.5174822880907,-30.4289029717636,
-30.3404121333621,-30.2502203375611,-30.1618268542744,-30.0734455957383,
-29.985055357441,-29.8935109598193,-29.8049904387251,-29.7119341028397,
-29.6188777669542,-29.5204908512767,-29.4223663703384,-29.3239283197183,
-29.2254902690982),.UNSPECIFIED.);
#86=B_SPLINE_CURVE_WITH_KNOTS('',3,(#7803,#7804,#7805,#7806,#7807,#7808,
#7809,#7810,#7811,#7812,#7813,#7814,#7815,#7816,#7817,#7818,#7819,#7820,
#7821,#7822,#7823,#7824,#7825,#7826,#7827,#7828,#7829,#7830,#7831,#7832,
#7833,#7834,#7835,#7836,#7837,#7838,#7839,#7840,#7841,#7842,#7843,#7844,
#7845,#7846,#7847,#7848,#7849,#7850,#7851,#7852,#7853,#7854,#7855,#7856,
#7857,#7858,#7859,#7860,#7861,#7862,#7863,#7864,#7865,#7866,#7867,#7868,
#7869,#7870,#7871,#7872,#7873,#7874,#7875,#7876,#7877,#7878,#7879,#7880,
#7881,#7882,#7883,#7884,#7885,#7886,#7887,#7888,#7889,#7890,#7891,#7892,
#7893,#7894,#7895,#7896,#7897,#7898,#7899,#7900,#7901,#7902,#7903,#7904,
#7905,#7906,#7907,#7908,#7909,#7910,#7911,#7912,#7913,#7914,#7915,#7916,
#7917,#7918,#7919,#7920,#7921,#7922,#7923,#7924,#7925,#7926,#7927,#7928,
#7929,#7930,#7931,#7932,#7933,#7934,#7935,#7936,#7937,#7938,#7939,#7940,
#7941,#7942,#7943,#7944,#7945,#7946,#7947,#7948,#7949,#7950,#7951,#7952,
#7953,#7954,#7955,#7956,#7957,#7958,#7959,#7960,#7961,#7962,#7963,#7964,
#7965,#7966,#7967,#7968,#7969,#7970,#7971,#7972,#7973,#7974,#7975,#7976,
#7977,#7978,#7979,#7980,#7981,#7982,#7983,#7984,#7985,#7986,#7987,#7988,
#7989,#7990,#7991,#7992,#7993,#7994,#7995,#7996,#7997,#7998,#7999,#8000,
#8001,#8002,#8003,#8004,#8005,#8006,#8007,#8008,#8009,#8010,#8011,#8012,
#8013,#8014,#8015,#8016),.UNSPECIFIED.,.F.,.F.,(4,3,3,3,3,3,3,3,3,3,3,3,
3,3,3,3,3,3,3,3,3,3,3,3,3,3,3,3,3,3,3,3,3,3,3,3,3,3,3,3,3,3,3,3,3,3,3,3,
3,3,3,3,3,3,3,3,3,3,3,3,3,3,3,3,3,3,3,3,3,3,3,4),(-29.2254902689125,-29.1359721824779,
-29.04643034499,-28.9568455388693,-28.8671374694578,-28.7773621997721,-28.6874306548523,
-28.6315818413891,-28.5428904368963,-28.4543111205044,-28.3658202820372,
-28.2756284862605,-28.1872350029049,-28.0988537442991,-28.0104635059315,
-27.9189191084046,-27.8303985872388,-27.7373422515314,-27.644285915824,
-27.555594511333,-27.4670151949429,-27.3785243564775,-27.2883325607001,
-27.1999390773468,-27.1115578187434,-27.0231675803786,-26.9316231828486,
-26.8431026616856,-26.7500463259722,-26.6569899902588,-26.5682985857523,
-26.4797192693466,-26.3912284308653,-26.3010366350939,-26.2126431517244,
-26.1242618931048,-26.0358716547238,-25.9443272572163,-25.8558067360371,
-25.7627504003654,-25.6696940646937,-25.5810026602034,-25.4924233438138,
-25.4039325053489,-25.3137407095713,-25.2253472262182,-25.1369659676149,
-25.0485757292499,-24.9570313317196,-24.8685108105561,-24.7754544748423,
-24.6823981391285,-24.5937067346351,-24.5051274182426,-24.416636579775,
-24.3264447839985,-24.2380513006428,-24.149670042037,-24.0612798036693,
-23.9697354061428,-23.8812148849775,-23.7881585492704,-23.6951022135634,
-23.607487371775,-23.5200096733413,-23.4326102403471,-23.3452667382789,
-23.2579568864533,-23.1706322164053,-23.0833009401675,-22.995900281291,
-22.9423049619356),.UNSPECIFIED.);
#87=B_SPLINE_CURVE_WITH_KNOTS('',3,(#8018,#8019,#8020,#8021,#8022,#8023,
#8024,#8025,#8026,#8027,#8028,#8029,#8030,#8031,#8032,#8033,#8034,#8035,
#8036,#8037,#8038,#8039,#8040,#8041,#8042,#8043,#8044,#8045,#8046,#8047,
#8048,#8049,#8050,#8051,#8052,#8053,#8054,#8055,#8056,#8057,#8058,#8059,
#8060,#8061,#8062,#8063,#8064,#8065,#8066,#8067,#8068,#8069,#8070,#8071,
#8072,#8073,#8074,#8075,#8076,#8077,#8078,#8079,#8080,#8081,#8082,#8083,
#8084,#8085,#8086,#8087,#8088,#8089,#8090,#8091,#8092,#8093,#8094,#8095,
#8096,#8097,#8098,#8099,#8100,#8101,#8102,#8103,#8104,#8105,#8106,#8107,
#8108,#8109,#8110,#8111,#8112,#8113,#8114,#8115,#8116,#8117,#8118,#8119,
#8120,#8121,#8122,#8123,#8124,#8125,#8126,#8127,#8128,#8129,#8130,#8131,
#8132,#8133,#8134,#8135,#8136,#8137,#8138,#8139,#8140,#8141,#8142,#8143,
#8144,#8145,#8146,#8147,#8148,#8149,#8150,#8151,#8152,#8153,#8154,#8155,
#8156,#8157,#8158,#8159,#8160,#8161,#8162,#8163,#8164,#8165,#8166,#8167,
#8168,#8169,#8170,#8171,#8172,#8173,#8174,#8175,#8176,#8177,#8178,#8179,
#8180,#8181,#8182,#8183,#8184,#8185,#8186,#8187,#8188,#8189,#8190,#8191,
#8192,#8193,#8194,#8195,#8196,#8197,#8198,#8199,#8200,#8201,#8202,#8203,
#8204,#8205,#8206,#8207,#8208,#8209,#8210,#8211,#8212,#8213,#8214,#8215,
#8216,#8217,#8218,#8219,#8220,#8221,#8222,#8223,#8224,#8225),
 .UNSPECIFIED.,.F.,.F.,(4,3,3,3,3,3,3,3,3,3,3,3,3,3,3,3,3,3,3,3,3,3,3,3,
3,3,3,3,3,3,3,3,3,3,3,3,3,3,3,3,3,3,3,3,3,3,3,3,3,3,3,3,3,3,3,3,3,3,3,3,
3,3,3,3,3,3,3,3,3,4),(-22.9423049617329,-22.8250556248655,-22.7078062879982,
-22.6191148835766,-22.5305355672557,-22.4420447288591,-22.3518529330559,
-22.2634594497701,-22.1750781912337,-22.086687952935,-21.9951435553095,
-21.9066230342105,-21.8135666983218,-21.7205103624331,-21.6318189579397,
-21.5432396415478,-21.4547488030814,-21.3645570073048,-21.276163523952,
-21.1877822653498,-21.0993920269868,-21.0078476294571,-20.9193271082973,
-20.8262707725827,-20.733214436868,-20.6445230320143,-20.5559437152602,
-20.4674528764303,-20.3772610807893,-20.2888675970716,-20.2004863381047,
-20.1120960993774,-20.0205517023588,-19.9320311808397,-19.8389748460713,
-19.7459185113028,-19.6572271076187,-19.5686477920344,-19.4801569543731,
-19.3899651582937,-19.3015716757345,-19.2131904179202,-19.1248001803384,
-19.0332557816882,-18.9447352612863,-18.851678923512,-18.7586225857377,
-18.6699311809424,-18.581351864255,-18.4928610254998,-18.4026692298339,
-18.3142757462105,-18.2258944873449,-18.1375042487258,-18.0459598515875,
-17.9574393301927,-17.8643829951826,-17.7713266601725,-17.6826352526863,
-17.5940559332877,-17.5055650918046,-17.4153732971549,-17.3269798107805,
-17.2385985491602,-17.1502083077859,-17.0586639144913,-16.9701433903655,
-16.8770870624864,-16.7840307346074,-16.6591196545534),.UNSPECIFIED.);
#88=B_SPLINE_CURVE_WITH_KNOTS('',3,(#8227,#8228,#8229,#8230,#8231,#8232,
#8233,#8234,#8235,#8236,#8237,#8238,#8239,#8240,#8241,#8242,#8243,#8244,
#8245,#8246,#8247,#8248,#8249,#8250,#8251,#8252,#8253,#8254,#8255,#8256,
#8257,#8258,#8259,#8260,#8261,#8262,#8263,#8264,#8265,#8266,#8267,#8268,
#8269,#8270,#8271,#8272,#8273,#8274,#8275,#8276,#8277,#8278,#8279,#8280,
#8281,#8282,#8283,#8284,#8285,#8286,#8287,#8288,#8289,#8290,#8291,#8292,
#8293,#8294,#8295,#8296,#8297,#8298,#8299,#8300,#8301,#8302,#8303,#8304,
#8305,#8306,#8307,#8308,#8309,#8310,#8311,#8312,#8313,#8314,#8315,#8316,
#8317,#8318,#8319,#8320,#8321,#8322,#8323,#8324,#8325,#8326,#8327,#8328,
#8329,#8330,#8331,#8332,#8333,#8334,#8335,#8336,#8337,#8338,#8339,#8340,
#8341,#8342,#8343,#8344,#8345,#8346,#8347,#8348,#8349,#8350,#8351,#8352,
#8353,#8354,#8355,#8356,#8357,#8358,#8359,#8360,#8361,#8362,#8363,#8364,
#8365,#8366,#8367,#8368,#8369,#8370,#8371,#8372,#8373,#8374,#8375,#8376,
#8377,#8378,#8379,#8380,#8381,#8382,#8383,#8384,#8385,#8386,#8387,#8388,
#8389,#8390,#8391,#8392,#8393,#8394,#8395,#8396,#8397,#8398,#8399,#8400,
#8401,#8402,#8403,#8404,#8405,#8406,#8407,#8408,#8409,#8410,#8411,#8412,
#8413,#8414,#8415,#8416,#8417,#8418,#8419,#8420,#8421,#8422,#8423,#8424,
#8425,#8426,#8427,#8428,#8429,#8430,#8431,#8432,#8433,#8434,#8435,#8436,
#8437,#8438,#8439,#8440),.UNSPECIFIED.,.F.,.F.,(4,3,3,3,3,3,3,3,3,3,3,3,
3,3,3,3,3,3,3,3,3,3,3,3,3,3,3,3,3,3,3,3,3,3,3,3,3,3,3,3,3,3,3,3,3,3,3,3,
3,3,3,3,3,3,3,3,3,3,3,3,3,3,3,3,3,3,3,3,3,3,3,4),(-16.6591196543414,-16.5717200910651,
-16.4844154992113,-16.3971811873345,-16.3099842840513,-16.2228024345668,
-16.1356133009829,-16.0483412871192,-15.9610276096757,-15.87357546279,-15.7967348090423,
-15.7080433984867,-15.6194640760958,-15.5309732317001,-15.4407814381722,
-15.3523879490976,-15.2640066848607,-15.1756164409559,-15.0840720515862,
-14.9955515251667,-14.9024952043219,-14.8094388834771,-14.7207474553443,
-14.6321681151713,-14.543677252813,-14.4534854659504,-14.3650919585897,
-14.2767106759796,-14.1883204136354,-14.0967760497045,-14.0082555048544,
-13.9151992313832,-13.822142957912,-13.7334516362746,-13.6448724027792,
-13.5563816471481,-13.4661898202979,-13.3777964190981,-13.2894152422491,
-13.2010250851483,-13.1094805719479,-13.0209601300808,-12.9279035812138,
-12.8348470323468,-12.7461555405831,-12.6575761374613,-12.5690852129039,
-12.4788934496386,-12.3904998823065,-12.302118540658,-12.2137282202711,
-12.1221839418987,-12.033663342007,-11.9406072243944,-11.8475511067817,
-11.7588595316319,-11.6702800431268,-11.5817890313202,-11.4915973000572,
-11.4032036414882,-11.3148222072874,-11.2264317931444,-11.1348876401625,
-11.0463669444147,-10.9533110628157,-10.8602551812166,-10.7667161797742,
-10.6690207217186,-10.5758796685901,-10.4828745688088,-10.3900370539,-10.3759343475515),
 .UNSPECIFIED.);
#89=B_SPLINE_CURVE_WITH_KNOTS('',3,(#8442,#8443,#8444,#8445,#8446,#8447,
#8448,#8449,#8450,#8451,#8452,#8453,#8454,#8455,#8456,#8457,#8458,#8459,
#8460,#8461,#8462,#8463,#8464,#8465,#8466,#8467,#8468,#8469,#8470,#8471,
#8472,#8473,#8474,#8475,#8476,#8477,#8478,#8479,#8480,#8481,#8482,#8483,
#8484,#8485,#8486,#8487,#8488,#8489,#8490,#8491,#8492,#8493,#8494,#8495,
#8496,#8497,#8498,#8499,#8500,#8501,#8502,#8503,#8504,#8505,#8506,#8507,
#8508,#8509,#8510,#8511,#8512,#8513,#8514,#8515,#8516,#8517,#8518,#8519,
#8520,#8521,#8522,#8523,#8524,#8525,#8526,#8527,#8528,#8529,#8530,#8531,
#8532,#8533,#8534,#8535,#8536,#8537,#8538,#8539,#8540,#8541,#8542,#8543,
#8544,#8545,#8546,#8547,#8548,#8549,#8550,#8551,#8552,#8553,#8554,#8555,
#8556,#8557,#8558,#8559,#8560,#8561,#8562,#8563,#8564,#8565,#8566,#8567,
#8568,#8569,#8570,#8571,#8572,#8573,#8574,#8575,#8576,#8577,#8578,#8579,
#8580,#8581,#8582,#8583,#8584,#8585,#8586,#8587,#8588,#8589,#8590,#8591,
#8592,#8593,#8594,#8595,#8596,#8597,#8598,#8599,#8600,#8601,#8602,#8603,
#8604,#8605,#8606,#8607,#8608,#8609,#8610,#8611,#8612,#8613,#8614,#8615,
#8616,#8617,#8618,#8619,#8620,#8621,#8622,#8623,#8624,#8625,#8626,#8627,
#8628,#8629,#8630,#8631,#8632,#8633,#8634,#8635,#8636,#8637,#8638,#8639,
#8640,#8641,#8642,#8643,#8644,#8645,#8646,#8647,#8648,#8649,#8650,#8651,
#8652,#8653,#8654,#8655),.UNSPECIFIED.,.F.,.F.,(4,3,3,3,3,3,3,3,3,3,3,3,
3,3,3,3,3,3,3,3,3,3,3,3,3,3,3,3,3,3,3,3,3,3,3,3,3,3,3,3,3,3,3,3,3,3,3,3,
3,3,3,3,3,3,3,3,3,3,3,3,3,3,3,3,3,3,3,3,3,3,3,4),(-10.3759343473738,-10.2837902926352,
-10.1915347289495,-10.0990763528878,-10.0065069835266,-9.91374116071349,
-9.87295925565141,-9.78426675875657,-9.69568635429885,-9.6071944333689,
-9.51700304545857,-9.42860850027105,-9.34022618937909,-9.25183490942041,
-9.16029201458688,-9.07177048796738,-8.97871690902682,-8.88566333008627,
-8.79697088473413,-8.70839051294174,-8.61989860602454,-8.52970720583661,
-8.44131262908495,-8.35293026978913,-8.26453892472304,-8.17299604467257,
-8.08447441228348,-7.99142090840231,-7.89836740452113,-7.8096833862846,
-7.72111147055351,-7.63262803793188,-7.54243346805989,-7.45404735558313,
-7.36567344174141,-7.2772905138185,-7.18573575510288,-7.09722239144174,
-7.00414693519887,-6.91107147895599,-6.82236744771185,-6.73377553668861,
-6.64527215066049,-6.55508507600178,-6.46667924075407,-6.37828572492622,
-6.28988333750439,-6.19835639147601,-6.10982410186788,-6.01679982762936,
-5.92377555339085,-5.83508023034925,-5.74649685627311,-5.65800182793224,
-5.56781155291893,-5.47941358452827,-5.39102773953078,-5.30263281915304,
-5.2110945213212,-5.1225691257749,-5.0295243768003,-4.93647962782571,-4.84911293708853,
-4.76185786747162,-4.67469860752171,-4.58759212279799,-4.50051596030311,
-4.41344769861368,-4.32632380717673,-4.23917101078679,-4.15191074349811,
-4.09274904038576),.UNSPECIFIED.);
#90=B_SPLINE_CURVE_WITH_KNOTS('',3,(#8657,#8658,#8659,#8660,#8661,#8662,
#8663,#8664,#8665,#8666,#8667,#8668,#8669,#8670,#8671,#8672,#8673,#8674,
#8675,#8676,#8677,#8678,#8679,#8680,#8681,#8682,#8683,#8684,#8685,#8686,
#8687,#8688,#8689,#8690,#8691,#8692,#8693,#8694,#8695,#8696,#8697,#8698,
#8699,#8700,#8701,#8702,#8703,#8704,#8705,#8706,#8707,#8708,#8709,#8710,
#8711,#8712,#8713,#8714,#8715,#8716,#8717,#8718,#8719,#8720,#8721,#8722,
#8723,#8724,#8725,#8726),.UNSPECIFIED.,.F.,.F.,(4,3,3,3,3,3,3,3,3,3,3,3,
3,3,3,3,3,3,3,3,3,3,3,4),(-4.09274904019418,-3.94918370226056,-3.86035654056811,
-3.77164163979092,-3.68301555586337,-3.59287458346738,-3.50434756300603,
-3.41583364513408,-3.32731177482659,-3.23595577529379,-3.14730739184115,
-3.05459758426828,-2.96188777669542,-2.87427787878097,-2.78677785774721,
-2.69608082521827,-2.60872550184669,-2.52139825894373,-2.43407686158953,
-2.34673908408296,-2.25931792435971,-2.17184692832522,-2.08425819340456,
-2.06120159751572),.UNSPECIFIED.);
#91=B_SPLINE_CURVE_WITH_KNOTS('',3,(#8727,#8728,#8729,#8730),
 .UNSPECIFIED.,.F.,.F.,(4,4),(-0.072372269045696,0.),.UNSPECIFIED.);
#92=B_SPLINE_CURVE_WITH_KNOTS('',3,(#8733,#8734,#8735,#8736,#8737,#8738,
#8739,#8740,#8741,#8742,#8743,#8744,#8745,#8746,#8747,#8748,#8749,#8750,
#8751,#8752,#8753,#8754,#8755,#8756,#8757,#8758,#8759,#8760,#8761,#8762,
#8763,#8764,#8765,#8766,#8767,#8768,#8769,#8770,#8771,#8772,#8773,#8774,
#8775,#8776,#8777,#8778,#8779,#8780,#8781,#8782,#8783,#8784,#8785,#8786,
#8787,#8788,#8789,#8790,#8791,#8792,#8793,#8794,#8795,#8796,#8797,#8798,
#8799,#8800,#8801,#8802,#8803,#8804,#8805,#8806,#8807,#8808,#8809,#8810,
#8811,#8812,#8813,#8814,#8815,#8816,#8817,#8818,#8819,#8820,#8821,#8822,
#8823,#8824,#8825,#8826,#8827,#8828,#8829,#8830,#8831,#8832,#8833,#8834,
#8835,#8836,#8837,#8838,#8839,#8840,#8841,#8842,#8843,#8844,#8845,#8846),
 .UNSPECIFIED.,.F.,.F.,(4,2,2,2,2,2,2,2,2,2,2,2,2,2,2,2,2,2,2,2,2,2,2,2,
2,2,2,2,2,2,2,2,2,2,2,2,2,2,2,2,2,2,2,2,2,2,2,2,2,2,2,2,2,2,2,2,4),(0.00517588011749154,
0.0875141621631935,0.1072706806158,0.123898613541391,0.134977664171004,
0.146087914916193,0.162900557465675,0.228641946111849,0.261168889263247,
0.274746197705738,0.285471908997522,0.291939864102497,0.298462335881067,
0.309614023097136,0.364820704487681,0.425322433259706,0.441105163970217,
0.452019069280532,0.46194567537565,0.478373502018443,0.549934333746339,
0.580819940517539,0.594012306981921,0.604502551232618,0.61087812943858,
0.617336449958275,0.628377441025916,0.685194213828864,0.725105755974606,
0.743833800434163,0.759770403011422,0.770632792912601,0.781704316206637,
0.798789989678684,0.864256114052101,0.914045413230296,0.924124080113808,
0.930380572452451,0.936930425784211,0.94835586165298,0.997887594077727,
1.04205592407398,1.06182765375212,1.07843147619386,1.0894570464359,1.10047842456566,
1.11706052554884,1.19615510002758,1.22179936635024,1.2385511971755,1.24609236952287,
1.2520834659821,1.26001903276934,1.27804395155722,1.33884421240203,1.36947904313667,
1.36958410658186),.UNSPECIFIED.);
#93=B_SPLINE_CURVE_WITH_KNOTS('',3,(#8850,#8851,#8852,#8853,#8854,#8855,
#8856,#8857,#8858,#8859,#8860,#8861,#8862,#8863,#8864,#8865,#8866,#8867,
#8868,#8869,#8870,#8871,#8872,#8873,#8874,#8875,#8876,#8877,#8878,#8879,
#8880),.UNSPECIFIED.,.F.,.F.,(4,3,3,3,3,3,3,3,3,3,4),(59.6902604184353,
59.7850915941644,59.8797805115036,59.974985048167,60.0694493384788,60.1638535857091,
60.2582198196451,60.3540190659364,60.4484022729338,60.5449095388721,60.6414168048105),
 .UNSPECIFIED.);
#94=B_SPLINE_CURVE_WITH_KNOTS('',3,(#8881,#8882,#8883,#8884,#8885,#8886,
#8887,#8888,#8889,#8890,#8891,#8892,#8893,#8894,#8895,#8896,#8897,#8898,
#8899,#8900,#8901,#8902,#8903,#8904,#8905,#8906,#8907,#8908,#8909,#8910,
#8911,#8912,#8913,#8914,#8915,#8916,#8917,#8918,#8919,#8920,#8921,#8922,
#8923,#8924,#8925,#8926,#8927,#8928,#8929,#8930,#8931,#8932,#8933,#8934,
#8935,#8936,#8937,#8938,#8939,#8940,#8941,#8942,#8943,#8944,#8945,#8946,
#8947,#8948,#8949,#8950,#8951,#8952,#8953),.UNSPECIFIED.,.F.,.F.,(4,3,3,
3,3,3,3,3,3,3,3,3,3,3,3,3,3,3,3,3,3,3,3,3,4),(57.6437844487799,57.679529028115,
57.7727160127017,57.8657816296418,57.9587533150178,58.0516627927366,58.1445408088069,
58.2374120244759,58.3303010886529,58.4232905025462,58.5163345053069,58.6095286199085,
58.6668249536802,58.7594480760478,58.8519476038469,58.9443517374887,59.0366938367222,
59.1290047385551,59.2213097753034,59.3136342681026,59.406065060458,59.4985528952185,
59.5912004323442,59.6541208792453,59.6902604182061),.UNSPECIFIED.);
#95=B_SPLINE_CURVE_WITH_KNOTS('',3,(#9178,#9179,#9180,#9181,#9182,#9183,
#9184,#9185,#9186,#9187,#9188,#9189,#9190,#9191,#9192,#9193,#9194,#9195,
#9196,#9197,#9198,#9199,#9200,#9201,#9202,#9203,#9204,#9205,#9206,#9207,
#9208,#9209,#9210,#9211,#9212,#9213,#9214,#9215,#9216,#9217,#9218,#9219,
#9220,#9221,#9222,#9223,#9224,#9225,#9226,#9227,#9228,#9229,#9230,#9231,
#9232,#9233,#9234,#9235,#9236,#9237,#9238,#9239,#9240,#9241,#9242,#9243,
#9244,#9245,#9246,#9247,#9248,#9249,#9250,#9251,#9252,#9253,#9254,#9255,
#9256,#9257,#9258,#9259,#9260,#9261,#9262,#9263,#9264,#9265,#9266,#9267,
#9268,#9269,#9270,#9271,#9272,#9273,#9274),.UNSPECIFIED.,.F.,.F.,(4,3,3,
3,3,3,3,3,3,3,3,3,3,3,3,3,3,3,3,3,3,3,3,3,3,3,3,3,3,3,3,3,4),(0.,0.0341321776409722,
0.0705192623706805,0.107542570976747,0.144565879582813,0.149931073663995,
0.155296491832842,0.191163208000379,0.227007229395259,0.262199303377544,
0.280217642131302,0.294754884682934,0.299547789786458,0.334097809215398,
0.367754528664766,0.40125928746162,0.405952789054922,0.427105611562154,
0.435491119142354,0.439986573782363,0.473632216631017,0.507584951788435,
0.54129439870138,0.566464885397458,0.571999583646233,0.605097850922722,
0.637624306629265,0.65106250367107,0.658566610550264,0.664632956637089,
0.696440307584404,0.727381547156091,0.744397949170633),.UNSPECIFIED.);
#96=B_SPLINE_CURVE_WITH_KNOTS('',3,(#9275,#9276,#9277,#9278,#9279,#9280,
#9281,#9282,#9283,#9284,#9285,#9286,#9287,#9288,#9289,#9290,#9291,#9292,
#9293,#9294,#9295,#9296,#9297,#9298,#9299,#9300,#9301,#9302,#9303,#9304,
#9305,#9306,#9307,#9308,#9309,#9310,#9311,#9312,#9313,#9314,#9315,#9316,
#9317,#9318,#9319,#9320,#9321,#9322,#9323,#9324,#9325,#9326,#9327,#9328,
#9329,#9330,#9331,#9332,#9333,#9334,#9335,#9336,#9337,#9338,#9339,#9340,
#9341,#9342,#9343,#9344,#9345,#9346,#9347,#9348,#9349,#9350,#9351,#9352,
#9353,#9354,#9355,#9356,#9357,#9358,#9359,#9360,#9361,#9362,#9363,#9364,
#9365,#9366,#9367,#9368,#9369,#9370,#9371),.UNSPECIFIED.,.F.,.F.,(4,3,3,
3,3,3,3,3,3,3,3,3,3,3,3,3,3,3,3,3,3,3,3,3,3,3,3,3,3,3,3,3,4),(-0.744397949170565,
-0.716065321046432,-0.684738321171649,-0.6654500864001,-0.659676869837572,
-0.653635757178455,-0.621601508366302,-0.588770968384987,-0.576827016705555,
-0.571499825003365,-0.56657139186745,-0.533059953254888,-0.499151341272541,
-0.46530750476424,-0.442807387674953,-0.437357263297704,-0.433075739176151,
-0.398167633212208,-0.37462939230316,-0.340534007097898,-0.306438621892637,
-0.298945074622502,-0.291596664676506,-0.256768715632937,-0.221366271582615,
-0.185516523185835,-0.155715905664787,-0.150803540172397,-0.145702635476358,
-0.108970996938497,-0.0721764084372337,-0.0360779656303773,0.),
 .UNSPECIFIED.);
#97=B_SPLINE_CURVE_WITH_KNOTS('',3,(#9373,#9374,#9375,#9376,#9377,#9378,
#9379,#9380,#9381,#9382,#9383,#9384,#9385,#9386,#9387,#9388,#9389,#9390,
#9391,#9392,#9393,#9394,#9395,#9396,#9397,#9398,#9399,#9400,#9401,#9402,
#9403,#9404,#9405,#9406,#9407,#9408,#9409,#9410,#9411,#9412,#9413,#9414,
#9415,#9416,#9417,#9418,#9419,#9420,#9421,#9422,#9423,#9424,#9425,#9426,
#9427,#9428,#9429,#9430,#9431,#9432,#9433,#9434,#9435,#9436,#9437,#9438,
#9439,#9440,#9441,#9442,#9443,#9444,#9445,#9446,#9447,#9448,#9449,#9450,
#9451,#9452,#9453,#9454,#9455,#9456,#9457,#9458,#9459,#9460),
 .UNSPECIFIED.,.F.,.F.,(4,3,3,3,3,3,3,3,3,3,3,3,3,3,3,3,3,3,3,3,3,3,3,3,
3,3,3,3,3,4),(-0.733997891590042,-0.707293145123096,-0.670548287271981,
-0.642147796310554,-0.636048214010822,-0.599925325890975,-0.563776896277331,
-0.543414361784613,-0.537860670969721,-0.502475354749529,-0.46734667480714,
-0.433107818857019,-0.409213763332795,-0.400709630257953,-0.394895586282691,
-0.361258743023151,-0.3374092393429,-0.303003250040855,-0.268725072296995,
-0.262744346017593,-0.256126575954077,-0.222699029434053,-0.189225882444478,
-0.156353015875858,-0.127820019143976,-0.123154998639534,-0.0909627469967315,
-0.0592242090186183,-0.0284625885623667,-1.98144071232518E-14),
 .UNSPECIFIED.);
#98=B_SPLINE_CURVE_WITH_KNOTS('',3,(#9686,#9687,#9688,#9689,#9690,#9691,
#9692,#9693,#9694,#9695,#9696,#9697,#9698,#9699,#9700,#9701,#9702,#9703,
#9704,#9705,#9706,#9707,#9708,#9709,#9710,#9711,#9712,#9713,#9714,#9715,
#9716,#9717,#9718,#9719,#9720,#9721,#9722,#9723,#9724,#9725,#9726,#9727,
#9728,#9729,#9730,#9731,#9732,#9733,#9734,#9735,#9736,#9737,#9738,#9739,
#9740,#9741,#9742,#9743,#9744,#9745,#9746,#9747,#9748,#9749,#9750,#9751,
#9752,#9753,#9754,#9755,#9756,#9757,#9758,#9759,#9760,#9761,#9762,#9763,
#9764,#9765,#9766,#9767,#9768,#9769,#9770,#9771,#9772,#9773,#9774,#9775,
#9776,#9777,#9778,#9779),.UNSPECIFIED.,.F.,.F.,(4,3,3,3,3,3,3,3,3,3,3,3,
3,3,3,3,3,3,3,3,3,3,3,3,3,3,3,3,3,3,3,4),(0.,0.0282467707211759,0.0592219961171841,
0.0911380280626913,0.123004042670125,0.127503949869102,0.132209344868245,
0.164838598782075,0.19801075530928,0.231513292775733,0.24872740517319,0.259243491625486,
0.263909575847483,0.298276876796931,0.333438871725855,0.368600866654779,
0.391892735514256,0.397647024497331,0.4032074794018,0.437128166042211,0.47167569725459,
0.506916270840531,0.535816784344498,0.541150939210018,0.546425336305492,
0.58238966892319,0.6186029543621,0.634791593471035,0.645487823943227,0.682320445220175,
0.718671345234703,0.741270768406407),.UNSPECIFIED.);
#99=B_SPLINE_CURVE_WITH_KNOTS('',3,(#9780,#9781,#9782,#9783),
 .UNSPECIFIED.,.F.,.F.,(4,4),(0.,0.0132617047994356),.UNSPECIFIED.);
#177=SHAPE_REPRESENTATION_RELATIONSHIP('SRR','None',#19477,#185);
#185=ADVANCED_BREP_SHAPE_REPRESENTATION('',(#201),#19437);
#193=STYLED_ITEM('',(#19524),#201);
#201=MANIFOLD_SOLID_BREP('Body1',#2020);
#209=FACE_BOUND('',#387,.T.);
#224=PLANE('',#2147);
#225=PLANE('',#2148);
#226=PLANE('',#2149);
#280=FACE_OUTER_BOUND('',#378,.T.);
#281=FACE_OUTER_BOUND('',#379,.T.);
#282=FACE_OUTER_BOUND('',#380,.T.);
#283=FACE_OUTER_BOUND('',#381,.T.);
#284=FACE_OUTER_BOUND('',#382,.T.);
#285=FACE_OUTER_BOUND('',#383,.T.);
#286=FACE_OUTER_BOUND('',#384,.T.);
#287=FACE_OUTER_BOUND('',#385,.T.);
#288=FACE_OUTER_BOUND('',#386,.T.);
#289=FACE_OUTER_BOUND('',#388,.T.);
#290=FACE_OUTER_BOUND('',#389,.T.);
#291=FACE_OUTER_BOUND('',#390,.T.);
#292=FACE_OUTER_BOUND('',#391,.T.);
#293=FACE_OUTER_BOUND('',#392,.T.);
#294=FACE_OUTER_BOUND('',#393,.T.);
#378=EDGE_LOOP('',(#1309,#1310,#1311,#1312));
#379=EDGE_LOOP('',(#1313,#1314,#1315,#1316,#1317));
#380=EDGE_LOOP('',(#1318,#1319,#1320,#1321,#1322));
#381=EDGE_LOOP('',(#1323,#1324,#1325,#1326,#1327));
#382=EDGE_LOOP('',(#1328,#1329,#1330,#1331,#1332));
#383=EDGE_LOOP('',(#1333,#1334,#1335,#1336,#1337));
#384=EDGE_LOOP('',(#1338,#1339,#1340,#1341,#1342));
#385=EDGE_LOOP('',(#1343,#1344,#1345,#1346,#1347,#1348));
#386=EDGE_LOOP('',(#1349));
#387=EDGE_LOOP('',(#1350,#1351,#1352,#1353,#1354,#1355,#1356,#1357,#1358,
#1359,#1360,#1361,#1362,#1363,#1364,#1365,#1366,#1367,#1368,#1369,#1370));
#388=EDGE_LOOP('',(#1371,#1372,#1373,#1374,#1375));
#389=EDGE_LOOP('',(#1376,#1377,#1378,#1379,#1380,#1381,#1382,#1383,#1384,
#1385,#1386,#1387,#1388,#1389,#1390,#1391,#1392,#1393,#1394,#1395,#1396,
#1397,#1398,#1399,#1400));
#390=EDGE_LOOP('',(#1401,#1402,#1403,#1404));
#391=EDGE_LOOP('',(#1405,#1406,#1407,#1408,#1409,#1410,#1411,#1412,#1413,
#1414,#1415,#1416,#1417,#1418,#1419,#1420,#1421,#1422,#1423,#1424,#1425,
#1426,#1427,#1428,#1429,#1430));
#392=EDGE_LOOP('',(#1431,#1432,#1433,#1434,#1435));
#393=EDGE_LOOP('',(#1436));
#481=LINE('',#2724,#608);
#482=LINE('',#2901,#609);
#483=LINE('',#3252,#610);
#484=LINE('',#3609,#611);
#485=LINE('',#3968,#612);
#486=LINE('',#4311,#613);
#487=LINE('',#4674,#614);
#488=LINE('',#5062,#615);
#608=VECTOR('',#2305,3.22275);
#609=VECTOR('',#2310,3.22275);
#610=VECTOR('',#2313,3.22275);
#611=VECTOR('',#2316,3.22275);
#612=VECTOR('',#2319,3.22275);
#613=VECTOR('',#2322,3.22275);
#614=VECTOR('',#2325,3.22275);
#615=VECTOR('',#2328,3.22275);
#738=CIRCLE('',#2133,3.22275);
#739=CIRCLE('',#2142,3.933);
#740=CIRCLE('',#2143,3.933);
#741=CIRCLE('',#2144,3.933);
#742=CIRCLE('',#2146,3.22275);
#782=VERTEX_POINT('',#2722);
#783=VERTEX_POINT('',#2723);
#784=VERTEX_POINT('',#2725);
#785=VERTEX_POINT('',#2838);
#786=VERTEX_POINT('',#2899);
#787=VERTEX_POINT('',#2900);
#788=VERTEX_POINT('',#2902);
#789=VERTEX_POINT('',#3250);
#790=VERTEX_POINT('',#3251);
#791=VERTEX_POINT('',#3431);
#792=VERTEX_POINT('',#3607);
#793=VERTEX_POINT('',#3608);
#794=VERTEX_POINT('',#3610);
#795=VERTEX_POINT('',#3966);
#796=VERTEX_POINT('',#3967);
#797=VERTEX_POINT('',#4137);
#798=VERTEX_POINT('',#4309);
#799=VERTEX_POINT('',#4310);
#800=VERTEX_POINT('',#4312);
#801=VERTEX_POINT('',#4672);
#802=VERTEX_POINT('',#4673);
#803=VERTEX_POINT('',#4855);
#804=VERTEX_POINT('',#5060);
#805=VERTEX_POINT('',#5061);
#806=VERTEX_POINT('',#5063);
#807=VERTEX_POINT('',#5264);
#808=VERTEX_POINT('',#5457);
#809=VERTEX_POINT('',#5459);
#810=VERTEX_POINT('',#5460);
#811=VERTEX_POINT('',#5462);
#812=VERTEX_POINT('',#5468);
#813=VERTEX_POINT('',#5686);
#814=VERTEX_POINT('',#5901);
#815=VERTEX_POINT('',#6110);
#816=VERTEX_POINT('',#6325);
#817=VERTEX_POINT('',#6540);
#818=VERTEX_POINT('',#6752);
#819=VERTEX_POINT('',#6967);
#820=VERTEX_POINT('',#7149);
#821=VERTEX_POINT('',#7151);
#822=VERTEX_POINT('',#7160);
#823=VERTEX_POINT('',#7375);
#824=VERTEX_POINT('',#7590);
#825=VERTEX_POINT('',#7802);
#826=VERTEX_POINT('',#8017);
#827=VERTEX_POINT('',#8226);
#828=VERTEX_POINT('',#8441);
#829=VERTEX_POINT('',#8656);
#830=VERTEX_POINT('',#8732);
#831=VERTEX_POINT('',#8847);
#832=VERTEX_POINT('',#8849);
#833=VERTEX_POINT('',#9685);
#1003=EDGE_CURVE('',#782,#783,#481,.T.);
#1004=EDGE_CURVE('',#784,#782,#49,.T.);
#1005=EDGE_CURVE('',#785,#784,#738,.T.);
#1006=EDGE_CURVE('',#785,#783,#50,.T.);
#1007=EDGE_CURVE('',#786,#787,#482,.T.);
#1008=EDGE_CURVE('',#788,#786,#51,.F.);
#1009=EDGE_CURVE('',#782,#788,#52,.T.);
#1010=EDGE_CURVE('',#783,#787,#53,.T.);
#1011=EDGE_CURVE('',#789,#790,#483,.T.);
#1012=EDGE_CURVE('',#786,#789,#54,.F.);
#1013=EDGE_CURVE('',#787,#791,#55,.T.);
#1014=EDGE_CURVE('',#791,#790,#56,.T.);
#1015=EDGE_CURVE('',#792,#793,#484,.T.);
#1016=EDGE_CURVE('',#794,#792,#57,.F.);
#1017=EDGE_CURVE('',#789,#794,#58,.F.);
#1018=EDGE_CURVE('',#790,#793,#59,.T.);
#1019=EDGE_CURVE('',#795,#796,#485,.T.);
#1020=EDGE_CURVE('',#792,#795,#60,.F.);
#1021=EDGE_CURVE('',#793,#797,#61,.T.);
#1022=EDGE_CURVE('',#797,#796,#62,.T.);
#1023=EDGE_CURVE('',#798,#799,#486,.T.);
#1024=EDGE_CURVE('',#800,#798,#63,.F.);
#1025=EDGE_CURVE('',#795,#800,#64,.F.);
#1026=EDGE_CURVE('',#796,#799,#65,.T.);
#1027=EDGE_CURVE('',#801,#802,#487,.T.);
#1028=EDGE_CURVE('',#798,#801,#66,.F.);
#1029=EDGE_CURVE('',#799,#803,#67,.T.);
#1030=EDGE_CURVE('',#803,#802,#68,.T.);
#1031=EDGE_CURVE('',#804,#805,#488,.T.);
#1032=EDGE_CURVE('',#806,#804,#69,.T.);
#1033=EDGE_CURVE('',#801,#806,#70,.F.);
#1034=EDGE_CURVE('',#802,#807,#71,.T.);
#1035=EDGE_CURVE('',#807,#805,#72,.F.);
#1036=EDGE_CURVE('',#808,#808,#739,.F.);
#1037=EDGE_CURVE('',#809,#810,#740,.T.);
#1038=EDGE_CURVE('',#810,#811,#73,.T.);
#1039=EDGE_CURVE('',#811,#812,#74,.T.);
#1040=EDGE_CURVE('',#812,#813,#75,.T.);
#1041=EDGE_CURVE('',#813,#814,#76,.T.);
#1042=EDGE_CURVE('',#814,#815,#77,.T.);
#1043=EDGE_CURVE('',#815,#816,#78,.T.);
#1044=EDGE_CURVE('',#816,#817,#79,.T.);
#1045=EDGE_CURVE('',#817,#818,#80,.T.);
#1046=EDGE_CURVE('',#818,#819,#81,.T.);
#1047=EDGE_CURVE('',#820,#819,#741,.F.);
#1048=EDGE_CURVE('',#820,#821,#82,.T.);
#1049=EDGE_CURVE('',#821,#822,#83,.T.);
#1050=EDGE_CURVE('',#822,#823,#84,.T.);
#1051=EDGE_CURVE('',#823,#824,#85,.T.);
#1052=EDGE_CURVE('',#824,#825,#86,.T.);
#1053=EDGE_CURVE('',#825,#826,#87,.T.);
#1054=EDGE_CURVE('',#826,#827,#88,.T.);
#1055=EDGE_CURVE('',#827,#828,#89,.T.);
#1056=EDGE_CURVE('',#828,#829,#90,.T.);
#1057=EDGE_CURVE('',#829,#809,#91,.T.);
#1058=EDGE_CURVE('',#805,#830,#92,.F.);
#1059=EDGE_CURVE('',#831,#830,#742,.T.);
#1060=EDGE_CURVE('',#832,#831,#93,.T.);
#1061=EDGE_CURVE('',#804,#832,#94,.T.);
#1062=EDGE_CURVE('',#819,#831,#95,.T.);
#1063=EDGE_CURVE('',#784,#810,#96,.T.);
#1064=EDGE_CURVE('',#809,#785,#97,.T.);
#1065=EDGE_CURVE('',#833,#820,#98,.T.);
#1066=EDGE_CURVE('',#830,#833,#99,.T.);
#1309=ORIENTED_EDGE('',*,*,#1003,.F.);
#1310=ORIENTED_EDGE('',*,*,#1004,.F.);
#1311=ORIENTED_EDGE('',*,*,#1005,.F.);
#1312=ORIENTED_EDGE('',*,*,#1006,.T.);
#1313=ORIENTED_EDGE('',*,*,#1007,.F.);
#1314=ORIENTED_EDGE('',*,*,#1008,.F.);
#1315=ORIENTED_EDGE('',*,*,#1009,.F.);
#1316=ORIENTED_EDGE('',*,*,#1003,.T.);
#1317=ORIENTED_EDGE('',*,*,#1010,.T.);
#1318=ORIENTED_EDGE('',*,*,#1011,.F.);
#1319=ORIENTED_EDGE('',*,*,#1012,.F.);
#1320=ORIENTED_EDGE('',*,*,#1007,.T.);
#1321=ORIENTED_EDGE('',*,*,#1013,.T.);
#1322=ORIENTED_EDGE('',*,*,#1014,.T.);
#1323=ORIENTED_EDGE('',*,*,#1015,.F.);
#1324=ORIENTED_EDGE('',*,*,#1016,.F.);
#1325=ORIENTED_EDGE('',*,*,#1017,.F.);
#1326=ORIENTED_EDGE('',*,*,#1011,.T.);
#1327=ORIENTED_EDGE('',*,*,#1018,.T.);
#1328=ORIENTED_EDGE('',*,*,#1019,.F.);
#1329=ORIENTED_EDGE('',*,*,#1020,.F.);
#1330=ORIENTED_EDGE('',*,*,#1015,.T.);
#1331=ORIENTED_EDGE('',*,*,#1021,.T.);
#1332=ORIENTED_EDGE('',*,*,#1022,.T.);
#1333=ORIENTED_EDGE('',*,*,#1023,.F.);
#1334=ORIENTED_EDGE('',*,*,#1024,.F.);
#1335=ORIENTED_EDGE('',*,*,#1025,.F.);
#1336=ORIENTED_EDGE('',*,*,#1019,.T.);
#1337=ORIENTED_EDGE('',*,*,#1026,.T.);
#1338=ORIENTED_EDGE('',*,*,#1027,.F.);
#1339=ORIENTED_EDGE('',*,*,#1028,.F.);
#1340=ORIENTED_EDGE('',*,*,#1023,.T.);
#1341=ORIENTED_EDGE('',*,*,#1029,.T.);
#1342=ORIENTED_EDGE('',*,*,#1030,.T.);
#1343=ORIENTED_EDGE('',*,*,#1031,.F.);
#1344=ORIENTED_EDGE('',*,*,#1032,.F.);
#1345=ORIENTED_EDGE('',*,*,#1033,.F.);
#1346=ORIENTED_EDGE('',*,*,#1027,.T.);
#1347=ORIENTED_EDGE('',*,*,#1034,.T.);
#1348=ORIENTED_EDGE('',*,*,#1035,.T.);
#1349=ORIENTED_EDGE('',*,*,#1036,.T.);
#1350=ORIENTED_EDGE('',*,*,#1037,.T.);
#1351=ORIENTED_EDGE('',*,*,#1038,.T.);
#1352=ORIENTED_EDGE('',*,*,#1039,.T.);
#1353=ORIENTED_EDGE('',*,*,#1040,.T.);
#1354=ORIENTED_EDGE('',*,*,#1041,.T.);
#1355=ORIENTED_EDGE('',*,*,#1042,.T.);
#1356=ORIENTED_EDGE('',*,*,#1043,.T.);
#1357=ORIENTED_EDGE('',*,*,#1044,.T.);
#1358=ORIENTED_EDGE('',*,*,#1045,.T.);
#1359=ORIENTED_EDGE('',*,*,#1046,.T.);
#1360=ORIENTED_EDGE('',*,*,#1047,.F.);
#1361=ORIENTED_EDGE('',*,*,#1048,.T.);
#1362=ORIENTED_EDGE('',*,*,#1049,.T.);
#1363=ORIENTED_EDGE('',*,*,#1050,.T.);
#1364=ORIENTED_EDGE('',*,*,#1051,.T.);
#1365=ORIENTED_EDGE('',*,*,#1052,.T.);
#1366=ORIENTED_EDGE('',*,*,#1053,.T.);
#1367=ORIENTED_EDGE('',*,*,#1054,.T.);
#1368=ORIENTED_EDGE('',*,*,#1055,.T.);
#1369=ORIENTED_EDGE('',*,*,#1056,.T.);
#1370=ORIENTED_EDGE('',*,*,#1057,.T.);
#1371=ORIENTED_EDGE('',*,*,#1031,.T.);
#1372=ORIENTED_EDGE('',*,*,#1058,.T.);
#1373=ORIENTED_EDGE('',*,*,#1059,.F.);
#1374=ORIENTED_EDGE('',*,*,#1060,.F.);
#1375=ORIENTED_EDGE('',*,*,#1061,.F.);
#1376=ORIENTED_EDGE('',*,*,#1062,.F.);
#1377=ORIENTED_EDGE('',*,*,#1046,.F.);
#1378=ORIENTED_EDGE('',*,*,#1045,.F.);
#1379=ORIENTED_EDGE('',*,*,#1044,.F.);
#1380=ORIENTED_EDGE('',*,*,#1043,.F.);
#1381=ORIENTED_EDGE('',*,*,#1042,.F.);
#1382=ORIENTED_EDGE('',*,*,#1041,.F.);
#1383=ORIENTED_EDGE('',*,*,#1040,.F.);
#1384=ORIENTED_EDGE('',*,*,#1039,.F.);
#1385=ORIENTED_EDGE('',*,*,#1038,.F.);
#1386=ORIENTED_EDGE('',*,*,#1063,.F.);
#1387=ORIENTED_EDGE('',*,*,#1004,.T.);
#1388=ORIENTED_EDGE('',*,*,#1009,.T.);
#1389=ORIENTED_EDGE('',*,*,#1008,.T.);
#1390=ORIENTED_EDGE('',*,*,#1012,.T.);
#1391=ORIENTED_EDGE('',*,*,#1017,.T.);
#1392=ORIENTED_EDGE('',*,*,#1016,.T.);
#1393=ORIENTED_EDGE('',*,*,#1020,.T.);
#1394=ORIENTED_EDGE('',*,*,#1025,.T.);
#1395=ORIENTED_EDGE('',*,*,#1024,.T.);
#1396=ORIENTED_EDGE('',*,*,#1028,.T.);
#1397=ORIENTED_EDGE('',*,*,#1033,.T.);
#1398=ORIENTED_EDGE('',*,*,#1032,.T.);
#1399=ORIENTED_EDGE('',*,*,#1061,.T.);
#1400=ORIENTED_EDGE('',*,*,#1060,.T.);
#1401=ORIENTED_EDGE('',*,*,#1037,.F.);
#1402=ORIENTED_EDGE('',*,*,#1064,.T.);
#1403=ORIENTED_EDGE('',*,*,#1005,.T.);
#1404=ORIENTED_EDGE('',*,*,#1063,.T.);
#1405=ORIENTED_EDGE('',*,*,#1065,.F.);
#1406=ORIENTED_EDGE('',*,*,#1066,.F.);
#1407=ORIENTED_EDGE('',*,*,#1058,.F.);
#1408=ORIENTED_EDGE('',*,*,#1035,.F.);
#1409=ORIENTED_EDGE('',*,*,#1034,.F.);
#1410=ORIENTED_EDGE('',*,*,#1030,.F.);
#1411=ORIENTED_EDGE('',*,*,#1029,.F.);
#1412=ORIENTED_EDGE('',*,*,#1026,.F.);
#1413=ORIENTED_EDGE('',*,*,#1022,.F.);
#1414=ORIENTED_EDGE('',*,*,#1021,.F.);
#1415=ORIENTED_EDGE('',*,*,#1018,.F.);
#1416=ORIENTED_EDGE('',*,*,#1014,.F.);
#1417=ORIENTED_EDGE('',*,*,#1013,.F.);
#1418=ORIENTED_EDGE('',*,*,#1010,.F.);
#1419=ORIENTED_EDGE('',*,*,#1006,.F.);
#1420=ORIENTED_EDGE('',*,*,#1064,.F.);
#1421=ORIENTED_EDGE('',*,*,#1057,.F.);
#1422=ORIENTED_EDGE('',*,*,#1056,.F.);
#1423=ORIENTED_EDGE('',*,*,#1055,.F.);
#1424=ORIENTED_EDGE('',*,*,#1054,.F.);
#1425=ORIENTED_EDGE('',*,*,#1053,.F.);
#1426=ORIENTED_EDGE('',*,*,#1052,.F.);
#1427=ORIENTED_EDGE('',*,*,#1051,.F.);
#1428=ORIENTED_EDGE('',*,*,#1050,.F.);
#1429=ORIENTED_EDGE('',*,*,#1049,.F.);
#1430=ORIENTED_EDGE('',*,*,#1048,.F.);
#1431=ORIENTED_EDGE('',*,*,#1065,.T.);
#1432=ORIENTED_EDGE('',*,*,#1047,.T.);
#1433=ORIENTED_EDGE('',*,*,#1062,.T.);
#1434=ORIENTED_EDGE('',*,*,#1059,.T.);
#1435=ORIENTED_EDGE('',*,*,#1066,.T.);
#1436=ORIENTED_EDGE('',*,*,#1036,.F.);
#1888=CYLINDRICAL_SURFACE('',#2132,3.22275);
#1889=CYLINDRICAL_SURFACE('',#2134,3.22275);
#1890=CYLINDRICAL_SURFACE('',#2135,3.22275);
#1891=CYLINDRICAL_SURFACE('',#2136,3.22275);
#1892=CYLINDRICAL_SURFACE('',#2137,3.22275);
#1893=CYLINDRICAL_SURFACE('',#2138,3.22275);
#1894=CYLINDRICAL_SURFACE('',#2139,3.22275);
#1895=CYLINDRICAL_SURFACE('',#2140,3.22275);
#1896=CYLINDRICAL_SURFACE('',#2141,3.933);
#1897=CYLINDRICAL_SURFACE('',#2145,3.22275);
#1929=ADVANCED_FACE('',(#280),#1888,.T.);
#1930=ADVANCED_FACE('',(#281),#1889,.T.);
#1931=ADVANCED_FACE('',(#282),#1890,.T.);
#1932=ADVANCED_FACE('',(#283),#1891,.T.);
#1933=ADVANCED_FACE('',(#284),#1892,.T.);
#1934=ADVANCED_FACE('',(#285),#1893,.T.);
#1935=ADVANCED_FACE('',(#286),#1894,.T.);
#1936=ADVANCED_FACE('',(#287),#1895,.T.);
#1937=ADVANCED_FACE('',(#288,#209),#1896,.T.);
#1938=ADVANCED_FACE('',(#289),#1897,.T.);
#1939=ADVANCED_FACE('',(#290),#43,.F.);
#1940=ADVANCED_FACE('',(#291),#224,.T.);
#1941=ADVANCED_FACE('',(#292),#44,.F.);
#1942=ADVANCED_FACE('',(#293),#225,.T.);
#1943=ADVANCED_FACE('',(#294),#226,.F.);
#2020=CLOSED_SHELL('',(#1929,#1930,#1931,#1932,#1933,#1934,#1935,#1936,
#1937,#1938,#1939,#1940,#1941,#1942,#1943));
#2131=AXIS2_PLACEMENT_3D('',#2720,#2301,#2302);
#2132=AXIS2_PLACEMENT_3D('',#2721,#2303,#2304);
#2133=AXIS2_PLACEMENT_3D('',#2839,#2306,#2307);
#2134=AXIS2_PLACEMENT_3D('',#2898,#2308,#2309);
#2135=AXIS2_PLACEMENT_3D('',#3249,#2311,#2312);
#2136=AXIS2_PLACEMENT_3D('',#3606,#2314,#2315);
#2137=AXIS2_PLACEMENT_3D('',#3965,#2317,#2318);
#2138=AXIS2_PLACEMENT_3D('',#4308,#2320,#2321);
#2139=AXIS2_PLACEMENT_3D('',#4671,#2323,#2324);
#2140=AXIS2_PLACEMENT_3D('',#5059,#2326,#2327);
#2141=AXIS2_PLACEMENT_3D('',#5456,#2329,#2330);
#2142=AXIS2_PLACEMENT_3D('',#5458,#2331,#2332);
#2143=AXIS2_PLACEMENT_3D('',#5461,#2333,#2334);
#2144=AXIS2_PLACEMENT_3D('',#7150,#2335,#2336);
#2145=AXIS2_PLACEMENT_3D('',#8731,#2337,#2338);
#2146=AXIS2_PLACEMENT_3D('',#8848,#2339,#2340);
#2147=AXIS2_PLACEMENT_3D('',#9372,#2341,#2342);
#2148=AXIS2_PLACEMENT_3D('',#9784,#2343,#2344);
#2149=AXIS2_PLACEMENT_3D('',#9785,#2345,#2346);
#2301=DIRECTION('axis',(0.,0.,1.));
#2302=DIRECTION('refdir',(1.,0.,0.));
#2303=DIRECTION('center_axis',(0.,0.,1.));
#2304=DIRECTION('ref_axis',(-0.853786006595012,0.52062410138462,0.));
#2305=DIRECTION('',(0.,0.,-1.));
#2306=DIRECTION('center_axis',(0.,0.,-1.));
#2307=DIRECTION('ref_axis',(-1.,-2.19773242311135E-14,0.));
#2308=DIRECTION('center_axis',(0.,0.,1.));
#2309=DIRECTION('ref_axis',(0.457827632423448,0.88904097711497,0.));
#2310=DIRECTION('',(0.,0.,-1.));
#2311=DIRECTION('center_axis',(0.,0.,1.));
#2312=DIRECTION('ref_axis',(0.457827632423448,0.88904097711497,0.));
#2313=DIRECTION('',(0.,0.,-1.));
#2314=DIRECTION('center_axis',(0.,0.,1.));
#2315=DIRECTION('ref_axis',(0.457827632423448,0.88904097711497,0.));
#2316=DIRECTION('',(0.,0.,-1.));
#2317=DIRECTION('center_axis',(0.,0.,1.));
#2318=DIRECTION('ref_axis',(0.457827632423448,0.88904097711497,0.));
#2319=DIRECTION('',(0.,0.,-1.));
#2320=DIRECTION('center_axis',(0.,0.,1.));
#2321=DIRECTION('ref_axis',(0.457827632423448,0.88904097711497,0.));
#2322=DIRECTION('',(0.,0.,-1.));
#2323=DIRECTION('center_axis',(0.,0.,1.));
#2324=DIRECTION('ref_axis',(0.457827632423448,0.88904097711497,0.));
#2325=DIRECTION('',(0.,0.,-1.));
#2326=DIRECTION('center_axis',(0.,0.,1.));
#2327=DIRECTION('ref_axis',(0.457827632423448,0.88904097711497,0.));
#2328=DIRECTION('',(0.,0.,-1.));
#2329=DIRECTION('center_axis',(0.,0.,1.));
#2330=DIRECTION('ref_axis',(-1.,0.,0.));
#2331=DIRECTION('center_axis',(0.,0.,-1.));
#2332=DIRECTION('ref_axis',(-1.,0.,0.));
#2333=DIRECTION('center_axis',(0.,0.,-1.));
#2334=DIRECTION('ref_axis',(-1.,0.,0.));
#2335=DIRECTION('center_axis',(0.,0.,-1.));
#2336=DIRECTION('ref_axis',(-1.,0.,0.));
#2337=DIRECTION('center_axis',(0.,0.,1.));
#2338=DIRECTION('ref_axis',(0.457827632423448,0.88904097711497,0.));
#2339=DIRECTION('center_axis',(0.,0.,1.));
#2340=DIRECTION('ref_axis',(-1.,-2.19773242311135E-14,0.));
#2341=DIRECTION('center_axis',(0.,0.,1.));
#2342=DIRECTION('ref_axis',(1.,0.,0.));
#2343=DIRECTION('center_axis',(0.,0.,1.));
#2344=DIRECTION('ref_axis',(-1.,0.,0.));
#2345=DIRECTION('center_axis',(0.,0.,1.));
#2346=DIRECTION('ref_axis',(-1.,0.,0.));
#2720=CARTESIAN_POINT('',(0.,0.,0.));
#2721=CARTESIAN_POINT('Origin',(0.,0.,294.689226550727));
#2722=CARTESIAN_POINT('',(-1.47546400239267,-2.86515680899727,297.653713253152));
#2723=CARTESIAN_POINT('',(-1.47546398584926,-2.86515681751659,297.410170442659));
#2724=CARTESIAN_POINT('',(-1.47546400239267,-2.86515680899727,294.689226550727));
#2725=CARTESIAN_POINT('',(1.87151685390576,2.62365055372218,297.000096128141));
#2726=CARTESIAN_POINT('Ctrl Pts',(1.87151685390576,2.62365055372218,297.000096128141));
#2727=CARTESIAN_POINT('Ctrl Pts',(1.79141615285366,2.68078842668167,297.00620095976));
#2728=CARTESIAN_POINT('Ctrl Pts',(1.70855111526434,2.7343581154886,297.012305791378));
#2729=CARTESIAN_POINT('Ctrl Pts',(1.62327730492518,2.78407764866838,297.018410622997));
#2730=CARTESIAN_POINT('Ctrl Pts',(1.53811042861501,2.83373483316243,297.024507799109));
#2731=CARTESIAN_POINT('Ctrl Pts',(1.45054116169697,2.87955123245278,297.030604975221));
#2732=CARTESIAN_POINT('Ctrl Pts',(1.3609557972031,2.9212868535218,297.036702151332));
#2733=CARTESIAN_POINT('Ctrl Pts',(1.27145830627926,2.96298153645274,297.042793346772));
#2734=CARTESIAN_POINT('Ctrl Pts',(1.179949049884,3.00060321142747,297.048884542213));
#2735=CARTESIAN_POINT('Ctrl Pts',(1.08683978303569,3.03395729180734,297.054975737653));
#2736=CARTESIAN_POINT('Ctrl Pts',(0.993779731326844,3.06729374208686,297.061063713446));
#2737=CARTESIAN_POINT('Ctrl Pts',(0.899121766051749,3.096366927626,297.067151689238));
#2738=CARTESIAN_POINT('Ctrl Pts',(0.80329768648275,3.12103034099181,297.073239665031));
#2739=CARTESIAN_POINT('Ctrl Pts',(0.707497314123379,3.14568765254362,297.079326134637));
#2740=CARTESIAN_POINT('Ctrl Pts',(0.610531830865964,3.16593724870124,297.085412604243));
#2741=CARTESIAN_POINT('Ctrl Pts',(0.512847160816357,3.18168278622219,297.09149907385));
#2742=CARTESIAN_POINT('Ctrl Pts',(0.415159192462197,3.19742885538826,297.097585748964));
#2743=CARTESIAN_POINT('Ctrl Pts',(0.316752428147877,3.20867049459657,297.103672424079));
#2744=CARTESIAN_POINT('Ctrl Pts',(0.21808078403911,3.21536286196953,297.109759099194));
#2745=CARTESIAN_POINT('Ctrl Pts',(0.119317279639045,3.2220614597324,297.115851440818));
#2746=CARTESIAN_POINT('Ctrl Pts',(0.0202888472946114,3.22420229773245,297.121943782441));
#2747=CARTESIAN_POINT('Ctrl Pts',(-0.0785480134665766,3.22179263331464,
297.128036124065));
#2748=CARTESIAN_POINT('Ctrl Pts',(-0.177431840313444,3.21938182385332,297.134131360696));
#2749=CARTESIAN_POINT('Ctrl Pts',(-0.276123470897804,3.21241623846137,297.140226597327));
#2750=CARTESIAN_POINT('Ctrl Pts',(-0.374171112763951,3.20095509822818,297.146321833958));
#2751=CARTESIAN_POINT('Ctrl Pts',(-0.472375829059162,3.18947559700207,297.152426835289));
#2752=CARTESIAN_POINT('Ctrl Pts',(-0.569934057389595,3.17348622911528,297.15853183662));
#2753=CARTESIAN_POINT('Ctrl Pts',(-0.66640380079212,3.1530974512041,297.164636837951));
#2754=CARTESIAN_POINT('Ctrl Pts',(-0.743036967641216,3.13690111270037,297.169486499297));
#2755=CARTESIAN_POINT('Ctrl Pts',(-0.818983426118032,3.11792963437914,297.174336160643));
#2756=CARTESIAN_POINT('Ctrl Pts',(-0.89402967360142,3.09626040655823,297.179185821989));
#2757=CARTESIAN_POINT('Ctrl Pts',(-0.989823629542428,3.06860038190994,297.185376248038));
#2758=CARTESIAN_POINT('Ctrl Pts',(-1.08448985773541,3.0364452542115,297.191566674086));
#2759=CARTESIAN_POINT('Ctrl Pts',(-1.17757729863649,2.99990487653125,297.197757100135));
#2760=CARTESIAN_POINT('Ctrl Pts',(-1.27054427470928,2.9634117858994,297.203939515129));
#2761=CARTESIAN_POINT('Ctrl Pts',(-1.36193612688466,2.92254488352808,297.210121930123));
#2762=CARTESIAN_POINT('Ctrl Pts',(-1.45131602364403,2.87746405051637,297.216304345117));
#2763=CARTESIAN_POINT('Ctrl Pts',(-1.5406061879105,2.83242847617775,297.222480553306));
#2764=CARTESIAN_POINT('Ctrl Pts',(-1.62788803009054,2.78318757691115,297.228656761496));
#2765=CARTESIAN_POINT('Ctrl Pts',(-1.71274467983952,2.7299493079875,297.234832969686));
#2766=CARTESIAN_POINT('Ctrl Pts',(-1.79754448300981,2.67674670407599,297.241005040353));
#2767=CARTESIAN_POINT('Ctrl Pts',(-1.87992195979798,2.61955228375788,297.24717711102));
#2768=CARTESIAN_POINT('Ctrl Pts',(-1.95948561107439,2.55861949154079,297.253349181687));
#2769=CARTESIAN_POINT('Ctrl Pts',(-2.03902221220878,2.49770741532473,297.259519153967));
#2770=CARTESIAN_POINT('Ctrl Pts',(-2.11574654703192,2.43305975523258,297.265689126246));
#2771=CARTESIAN_POINT('Ctrl Pts',(-2.18929756661504,2.36497224662648,297.271859098526));
#2772=CARTESIAN_POINT('Ctrl Pts',(-2.26284290673704,2.29688999560021,297.278028594372));
#2773=CARTESIAN_POINT('Ctrl Pts',(-2.33321510254691,2.22536871743231,297.284198090219));
#2774=CARTESIAN_POINT('Ctrl Pts',(-2.4000882941973,2.15074260258104,297.290367586065));
#2775=CARTESIAN_POINT('Ctrl Pts',(-2.46697389341984,2.07610264168952,297.296538226593));
#2776=CARTESIAN_POINT('Ctrl Pts',(-2.5303589108648,1.99835702081822,297.30270886712));
#2777=CARTESIAN_POINT('Ctrl Pts',(-2.58995692026528,1.91787400881027,297.308879507648));
#2778=CARTESIAN_POINT('Ctrl Pts',(-2.64961799436772,1.83730583226049,297.315056677749));
#2779=CARTESIAN_POINT('Ctrl Pts',(-2.70548380233446,1.75399482833522,297.321233847851));
#2780=CARTESIAN_POINT('Ctrl Pts',(-2.75731060812822,1.66833922593806,297.327411017952));
#2781=CARTESIAN_POINT('Ctrl Pts',(-2.80916732135543,1.58263419469439,297.333591752682));
#2782=CARTESIAN_POINT('Ctrl Pts',(-2.8569801844651,1.4945822491352,297.339772487412));
#2783=CARTESIAN_POINT('Ctrl Pts',(-2.90055185139118,1.40460546769945,297.345953222142));
#2784=CARTESIAN_POINT('Ctrl Pts',(-2.94419234272329,1.31448656182883,297.352143719762));
#2785=CARTESIAN_POINT('Ctrl Pts',(-2.98357808941882,1.22243714456876,297.358334217382));
#2786=CARTESIAN_POINT('Ctrl Pts',(-3.01856020756448,1.12889850553906,297.364524715002));
#2787=CARTESIAN_POINT('Ctrl Pts',(-3.03942608990356,1.07310525059589,297.368217178517));
#2788=CARTESIAN_POINT('Ctrl Pts',(-3.0587262063523,1.01678246065064,297.371909642033));
#2789=CARTESIAN_POINT('Ctrl Pts',(-3.07643756647016,0.960025761170579,297.375602105549));
#2790=CARTESIAN_POINT('Ctrl Pts',(-3.10606820094873,0.865073312272688,297.381779498817));
#2791=CARTESIAN_POINT('Ctrl Pts',(-3.13134962751106,0.768584728667232,297.387956892085));
#2792=CARTESIAN_POINT('Ctrl Pts',(-3.15212371614888,0.670994516066822,297.394134285353));
#2793=CARTESIAN_POINT('Ctrl Pts',(-3.17287014539651,0.573534238686073,297.400303453812));
#2794=CARTESIAN_POINT('Ctrl Pts',(-3.18912107616278,0.474975668252509,297.40647262227));
#2795=CARTESIAN_POINT('Ctrl Pts',(-3.2007678817287,0.37576925072976,297.412641790728));
#2796=CARTESIAN_POINT('Ctrl Pts',(-3.21240260373906,0.276665759820667,297.418804558677));
#2797=CARTESIAN_POINT('Ctrl Pts',(-3.21944264763299,0.176916186463936,297.424967326625));
#2798=CARTESIAN_POINT('Ctrl Pts',(-3.22183045528502,0.0769810359627175,
297.431130094574));
#2799=CARTESIAN_POINT('Ctrl Pts',(-3.22421656964183,-0.022883246303877,
297.437288492244));
#2800=CARTESIAN_POINT('Ctrl Pts',(-3.22195699700505,-0.122932411931123,
297.443446889914));
#2801=CARTESIAN_POINT('Ctrl Pts',(-3.21504610200097,-0.222701873607629,
297.449605287583));
#2802=CARTESIAN_POINT('Ctrl Pts',(-3.20813771679354,-0.322435102486507,
297.455761448737));
#2803=CARTESIAN_POINT('Ctrl Pts',(-3.19658139593122,-0.421888397275395,
297.461917609891));
#2804=CARTESIAN_POINT('Ctrl Pts',(-3.18042357849842,-0.520599100874478,
297.468073771045));
#2805=CARTESIAN_POINT('Ctrl Pts',(-3.16426732873914,-0.619300227303995,
297.474229334912));
#2806=CARTESIAN_POINT('Ctrl Pts',(-3.14351054030028,-0.717258478044924,
297.480384898779));
#2807=CARTESIAN_POINT('Ctrl Pts',(-3.1182511545876,-0.814019225456698,297.486540462647));
#2808=CARTESIAN_POINT('Ctrl Pts',(-3.09298749710563,-0.910796336670578,
297.492697067519));
#2809=CARTESIAN_POINT('Ctrl Pts',(-3.06321983936119,-1.0063751228674,297.498853672391));
#2810=CARTESIAN_POINT('Ctrl Pts',(-3.02909632157031,-1.10031497179181,297.505010277263));
#2811=CARTESIAN_POINT('Ctrl Pts',(-2.99493701929128,-1.19435333310969,297.511173338415));
#2812=CARTESIAN_POINT('Ctrl Pts',(-2.95641288494598,-1.28674891743634,297.517336399566));
#2813=CARTESIAN_POINT('Ctrl Pts',(-2.91372061764584,-1.37708014465591,297.523499460717));
#2814=CARTESIAN_POINT('Ctrl Pts',(-2.87100408196638,-1.46746272057691,297.529666025255));
#2815=CARTESIAN_POINT('Ctrl Pts',(-2.82411489797059,-1.55577821966582,297.535832589793));
#2816=CARTESIAN_POINT('Ctrl Pts',(-2.77329526067888,-1.64163057951418,297.54199915433));
#2817=CARTESIAN_POINT('Ctrl Pts',(-2.72239482155023,-1.72761944227266,297.548175523537));
#2818=CARTESIAN_POINT('Ctrl Pts',(-2.66755168691305,-1.81113698255652,297.554351892744));
#2819=CARTESIAN_POINT('Ctrl Pts',(-2.60905081857773,-1.89181695430052,297.560528261951));
#2820=CARTESIAN_POINT('Ctrl Pts',(-2.57277371178145,-1.94184759546128,297.564358304337));
#2821=CARTESIAN_POINT('Ctrl Pts',(-2.53509087092948,-1.99078772839539,297.568188346723));
#2822=CARTESIAN_POINT('Ctrl Pts',(-2.49607753242807,-2.03855696869325,297.572018389109));
#2823=CARTESIAN_POINT('Ctrl Pts',(-2.43309809797871,-2.1156711007721,297.578201246374));
#2824=CARTESIAN_POINT('Ctrl Pts',(-2.36643510744065,-2.18999455866235,297.584384103639));
#2825=CARTESIAN_POINT('Ctrl Pts',(-2.2963650479526,-2.26115570650092,297.590566960904));
#2826=CARTESIAN_POINT('Ctrl Pts',(-2.22640572126366,-2.33220439727657,297.596740047304));
#2827=CARTESIAN_POINT('Ctrl Pts',(-2.15305033958826,-2.40010041536909,297.602913133704));
#2828=CARTESIAN_POINT('Ctrl Pts',(-2.07661568444226,-2.46450499322448,297.609086220104));
#2829=CARTESIAN_POINT('Ctrl Pts',(-2.00025084138479,-2.52885074674054,297.615253668275));
#2830=CARTESIAN_POINT('Ctrl Pts',(-1.92081264186164,-2.58971111871789,297.621421116447));
#2831=CARTESIAN_POINT('Ctrl Pts',(-1.83865445309451,-2.64678434418366,297.627588564618));
#2832=CARTESIAN_POINT('Ctrl Pts',(-1.75655585229805,-2.70381617538629,297.633751539642));
#2833=CARTESIAN_POINT('Ctrl Pts',(-1.67174153991997,-2.75706607659332,297.639914514665));
#2834=CARTESIAN_POINT('Ctrl Pts',(-1.58459681948458,-2.80627341543538,297.646077489689));
#2835=CARTESIAN_POINT('Ctrl Pts',(-1.54860681629195,-2.82659561364978,297.648622744177));
#2836=CARTESIAN_POINT('Ctrl Pts',(-1.51221969163722,-2.84622880610641,297.651167998664));
#2837=CARTESIAN_POINT('Ctrl Pts',(-1.47546400239267,-2.86515680899727,297.653713253152));
#2838=CARTESIAN_POINT('',(-1.87158653173916,2.62360084935048,297.));
#2839=CARTESIAN_POINT('Origin',(0.,0.,297.));
#2840=CARTESIAN_POINT('Ctrl Pts',(-1.87158653173917,2.62360084935048,297.));
#2841=CARTESIAN_POINT('Ctrl Pts',(-1.89151501090213,2.60938455832866,297.001511146392));
#2842=CARTESIAN_POINT('Ctrl Pts',(-1.91128147124222,2.5949412363802,297.00300977116));
#2843=CARTESIAN_POINT('Ctrl Pts',(-1.95983501508414,2.55860742914849,297.006694908871));
#2844=CARTESIAN_POINT('Ctrl Pts',(-1.98842232314421,2.53645463522962,297.008868175637));
#2845=CARTESIAN_POINT('Ctrl Pts',(-2.13255247496678,2.42083104011892,297.01987385646));
#2846=CARTESIAN_POINT('Ctrl Pts',(-2.24191063438775,2.31992370603537,297.028391387703));
#2847=CARTESIAN_POINT('Ctrl Pts',(-2.46530621998206,2.08318620708576,297.047026520952));
#2848=CARTESIAN_POINT('Ctrl Pts',(-2.57589028177142,1.94478371461386,297.057118274445));
#2849=CARTESIAN_POINT('Ctrl Pts',(-2.70940464418189,1.74618011739376,297.071255356244));
#2850=CARTESIAN_POINT('Ctrl Pts',(-2.74273483708399,1.69334683074426,297.074984204102));
#2851=CARTESIAN_POINT('Ctrl Pts',(-2.7950495198796,1.60481962890104,297.081204455471));
#2852=CARTESIAN_POINT('Ctrl Pts',(-2.81493561634823,1.56967676057289,297.083666710306));
#2853=CARTESIAN_POINT('Ctrl Pts',(-2.8532321465274,1.49892952774936,297.088615648114));
#2854=CARTESIAN_POINT('Ctrl Pts',(-2.87164905468074,1.46333690847566,297.091101568197));
#2855=CARTESIAN_POINT('Ctrl Pts',(-2.91608813159483,1.37338236282152,297.097380141935));
#2856=CARTESIAN_POINT('Ctrl Pts',(-2.94125721501756,1.31861835794363,297.101198954259));
#2857=CARTESIAN_POINT('Ctrl Pts',(-3.06310458212016,1.03262491785649,297.121145009664));
#2858=CARTESIAN_POINT('Ctrl Pts',(-3.13409080569824,0.791428840294966,297.13806703326));
#2859=CARTESIAN_POINT('Ctrl Pts',(-3.19560910512955,0.432550735117186,297.162772691734));
#2860=CARTESIAN_POINT('Ctrl Pts',(-3.2088682612389,0.319663245654916,297.170462687525));
#2861=CARTESIAN_POINT('Ctrl Pts',(-3.21914654228964,0.159434016087073,297.181108231019));
#2862=CARTESIAN_POINT('Ctrl Pts',(-3.22112839309526,0.112498732676699,297.184193686169));
#2863=CARTESIAN_POINT('Ctrl Pts',(-3.22283301721058,0.0286891419506858,
297.189627765798));
#2864=CARTESIAN_POINT('Ctrl Pts',(-3.22295039765794,-0.00816845506468047,
297.191991529349));
#2865=CARTESIAN_POINT('Ctrl Pts',(-3.22213315783248,-0.0666625260269022,
297.195693911339));
#2866=CARTESIAN_POINT('Ctrl Pts',(-3.22161280522507,-0.0883004785492859,
297.197052839046));
#2867=CARTESIAN_POINT('Ctrl Pts',(-3.22016204112837,-0.130806011876565,
297.199699403599));
#2868=CARTESIAN_POINT('Ctrl Pts',(-3.2192466890242,-0.15167255601355,297.200987579638));
#2869=CARTESIAN_POINT('Ctrl Pts',(-3.21629995036034,-0.206637096286946,
297.20435494168));
#2870=CARTESIAN_POINT('Ctrl Pts',(-3.21392914815483,-0.240715394021917,
297.206416577875));
#2871=CARTESIAN_POINT('Ctrl Pts',(-3.19355424788907,-0.47883694661062,297.220679927958));
#2872=CARTESIAN_POINT('Ctrl Pts',(-3.15667236462029,-0.68081800582869,297.232069265853));
#2873=CARTESIAN_POINT('Ctrl Pts',(-3.05209968839318,-1.05016165625582,297.253659071756));
#2874=CARTESIAN_POINT('Ctrl Pts',(-2.9890851907885,-1.2179954617432,297.263791240634));
#2875=CARTESIAN_POINT('Ctrl Pts',(-2.89116624536072,-1.42469347743832,297.277321614191));
#2876=CARTESIAN_POINT('Ctrl Pts',(-2.86882461384046,-1.46916258475178,297.280296856216));
#2877=CARTESIAN_POINT('Ctrl Pts',(-2.82908961162629,-1.5438865742787,297.285417905799));
#2878=CARTESIAN_POINT('Ctrl Pts',(-2.81221773925494,-1.5744094204346,297.287545228085));
#2879=CARTESIAN_POINT('Ctrl Pts',(-2.77679274541169,-1.6361098551466,297.291921949513));
#2880=CARTESIAN_POINT('Ctrl Pts',(-2.75820190641163,-1.66725987159154,297.294172499382));
#2881=CARTESIAN_POINT('Ctrl Pts',(-2.70887846405452,-1.74682070859336,297.300030720848));
#2882=CARTESIAN_POINT('Ctrl Pts',(-2.67737365654439,-1.7947352844465,297.303666606203));
#2883=CARTESIAN_POINT('Ctrl Pts',(-2.51535548869813,-2.02737671830831,297.321873988285));
#2884=CARTESIAN_POINT('Ctrl Pts',(-2.36694320299785,-2.19882201149093,297.33713143598));
#2885=CARTESIAN_POINT('Ctrl Pts',(-2.07642187633599,-2.47064582761142,297.364161641344));
#2886=CARTESIAN_POINT('Ctrl Pts',(-1.94180921729375,-2.57779094123865,297.375828218173));
#2887=CARTESIAN_POINT('Ctrl Pts',(-1.77165654763903,-2.69229638299389,297.389088817439));
#2888=CARTESIAN_POINT('Ctrl Pts',(-1.74373830172358,-2.71046189452414,297.391219825866));
#2889=CARTESIAN_POINT('Ctrl Pts',(-1.69839475250396,-2.73897483142018,297.394603283233));
#2890=CARTESIAN_POINT('Ctrl Pts',(-1.68114546687041,-2.74959594696396,297.395872611772));
#2891=CARTESIAN_POINT('Ctrl Pts',(-1.64565612078635,-2.77098937504568,297.39844683352));
#2892=CARTESIAN_POINT('Ctrl Pts',(-1.62740842460557,-2.7817455063204,297.399750915196));
#2893=CARTESIAN_POINT('Ctrl Pts',(-1.57842496984379,-2.80997187616802,297.403203392058));
#2894=CARTESIAN_POINT('Ctrl Pts',(-1.54750474949298,-2.82711807487197,297.405332765564));
#2895=CARTESIAN_POINT('Ctrl Pts',(-1.50274205757047,-2.85098582998335,297.408353435895));
#2896=CARTESIAN_POINT('Ctrl Pts',(-1.48912726939844,-2.85812066414376,297.409264091));
#2897=CARTESIAN_POINT('Ctrl Pts',(-1.47546398584926,-2.86515681751659,297.410170442659));
#2898=CARTESIAN_POINT('Origin',(0.,0.,294.689226550727));
#2899=CARTESIAN_POINT('',(-1.47546409036591,-2.86515676369386,298.903152516993));
#2900=CARTESIAN_POINT('',(-1.47546399981363,-2.86515681032539,298.654589343883));
#2901=CARTESIAN_POINT('',(-1.47546400239267,-2.86515680899727,294.689226550727));
#2902=CARTESIAN_POINT('',(3.22274999369119,-0.000201651753011577,298.060773449234));
#2903=CARTESIAN_POINT('Ctrl Pts',(-1.47546409036594,-2.86515676369385,298.903152516993));
#2904=CARTESIAN_POINT('Ctrl Pts',(-1.6591960385397,-2.77054068710826,298.891552718834));
#2905=CARTESIAN_POINT('Ctrl Pts',(-1.83345625504359,-2.65844361410806,298.879965681433));
#2906=CARTESIAN_POINT('Ctrl Pts',(-2.03848911916688,-2.49672422759705,298.864567628018));
#2907=CARTESIAN_POINT('Ctrl Pts',(-2.08029032183093,-2.46200354033995,298.861327433074));
#2908=CARTESIAN_POINT('Ctrl Pts',(-2.14590885635884,-2.404635232992,298.856062741298));
#2909=CARTESIAN_POINT('Ctrl Pts',(-2.17029311842409,-2.3826504324519,298.854064920298));
#2910=CARTESIAN_POINT('Ctrl Pts',(-2.22076152090531,-2.33573064346003,298.849839082774));
#2911=CARTESIAN_POINT('Ctrl Pts',(-2.24677114267321,-2.31072253620592,298.847608164488));
#2912=CARTESIAN_POINT('Ctrl Pts',(-2.30930897980404,-2.24853851159302,298.842109267261));
#2913=CARTESIAN_POINT('Ctrl Pts',(-2.3453648036758,-2.21090407871771,298.83882178845));
#2914=CARTESIAN_POINT('Ctrl Pts',(-2.51658583690561,-2.02328323331635,298.822616507258));
#2915=CARTESIAN_POINT('Ctrl Pts',(-2.6383466108852,-1.86171539963794,298.809175177368));
#2916=CARTESIAN_POINT('Ctrl Pts',(-2.84071143788486,-1.53309064159345,298.783168906886));
#2917=CARTESIAN_POINT('Ctrl Pts',(-2.92363824819888,-1.36834082840619,298.7706881872));
#2918=CARTESIAN_POINT('Ctrl Pts',(-3.00578395655033,-1.16307666829401,298.756382966809));
#2919=CARTESIAN_POINT('Ctrl Pts',(-3.0189299383629,-1.12851531661196,298.75401545357));
#2920=CARTESIAN_POINT('Ctrl Pts',(-3.03879817190377,-1.07344695303929,298.750316131406));
#2921=CARTESIAN_POINT('Ctrl Pts',(-3.04591391774224,-1.05308649083907,298.748963961046));
#2922=CARTESIAN_POINT('Ctrl Pts',(-3.0595761224216,-1.012697105867,298.746314456983));
#2923=CARTESIAN_POINT('Ctrl Pts',(-3.06613155932879,-0.992672544564584,
298.745016737267));
#2924=CARTESIAN_POINT('Ctrl Pts',(-3.08291771229299,-0.939643440628762,
298.741618383366));
#2925=CARTESIAN_POINT('Ctrl Pts',(-3.09281515472522,-0.906535188865807,
298.739535501352));
#2926=CARTESIAN_POINT('Ctrl Pts',(-3.11392929785717,-0.831530161019412,
298.734890812584));
#2927=CARTESIAN_POINT('Ctrl Pts',(-3.12483674935978,-0.789552846483335,
298.732342774009));
#2928=CARTESIAN_POINT('Ctrl Pts',(-3.15828145695989,-0.649266082201744,
298.723959497458));
#2929=CARTESIAN_POINT('Ctrl Pts',(-3.17705246238441,-0.550116424821424,
298.718247236005));
#2930=CARTESIAN_POINT('Ctrl Pts',(-3.22499356732628,-0.210330398377229,
298.698932430009));
#2931=CARTESIAN_POINT('Ctrl Pts',(-3.23167902450801,0.0326145108600474,
298.685497356927));
#2932=CARTESIAN_POINT('Ctrl Pts',(-3.20649373452886,0.327758383857938,298.668024653567));
#2933=CARTESIAN_POINT('Ctrl Pts',(-3.2005585338958,0.381381969750893,298.664806732028));
#2934=CARTESIAN_POINT('Ctrl Pts',(-3.18885961360891,0.46729601691632,298.659568379224));
#2935=CARTESIAN_POINT('Ctrl Pts',(-3.1839438446911,0.499692582311363,298.657574098447));
#2936=CARTESIAN_POINT('Ctrl Pts',(-3.17256922501014,0.567651427338976,298.653347858176));
#2937=CARTESIAN_POINT('Ctrl Pts',(-3.1660044147582,0.603191106258999,298.651112875841));
#2938=CARTESIAN_POINT('Ctrl Pts',(-3.14844664871458,0.69003923113951,298.645587125001));
#2939=CARTESIAN_POINT('Ctrl Pts',(-3.13679592483552,0.741202577938277,298.642276401362));
#2940=CARTESIAN_POINT('Ctrl Pts',(-3.07527219724289,0.983854585014435,298.626300206029));
#2941=CARTESIAN_POINT('Ctrl Pts',(-3.00908909751798,1.17073940105393,298.613135594628));
#2942=CARTESIAN_POINT('Ctrl Pts',(-2.8476123523373,1.5206586346405,298.587172357915));
#2943=CARTESIAN_POINT('Ctrl Pts',(-2.75429821604088,1.68379009583437,298.574447194288));
#2944=CARTESIAN_POINT('Ctrl Pts',(-2.62630800401366,1.86814911927084,298.559927696015));
#2945=CARTESIAN_POINT('Ctrl Pts',(-2.60477938358137,1.89805149743848,298.557568832788));
#2946=CARTESIAN_POINT('Ctrl Pts',(-2.56985873263698,1.94484127813371,298.553879806655));
#2947=CARTESIAN_POINT('Ctrl Pts',(-2.55680258421338,1.96197403370382,298.552529460067));
#2948=CARTESIAN_POINT('Ctrl Pts',(-2.53062283313602,1.99562284741262,298.549880372227));
#2949=CARTESIAN_POINT('Ctrl Pts',(-2.51750700065251,2.01214338918097,298.54858129126));
#2950=CARTESIAN_POINT('Ctrl Pts',(-2.48240929964527,2.05547156835581,298.545174797424));
#2951=CARTESIAN_POINT('Ctrl Pts',(-2.46015481709589,2.08205614496051,298.543085291257));
#2952=CARTESIAN_POINT('Ctrl Pts',(-2.40898051929473,2.14122105581336,298.538423026225));
#2953=CARTESIAN_POINT('Ctrl Pts',(-2.37982011345836,2.17358489831474,298.535864193234));
#2954=CARTESIAN_POINT('Ctrl Pts',(-2.28046718034941,2.27945499922921,298.527426252839));
#2955=CARTESIAN_POINT('Ctrl Pts',(-2.20745263262055,2.35023419787734,298.521671815143));
#2956=CARTESIAN_POINT('Ctrl Pts',(-1.9507171707951,2.57657108956049,298.502410249197));
#2957=CARTESIAN_POINT('Ctrl Pts',(-1.75298689405621,2.71496659631791,298.489062451772));
#2958=CARTESIAN_POINT('Ctrl Pts',(-1.49412873871142,2.85598174572173,298.471678239932));
#2959=CARTESIAN_POINT('Ctrl Pts',(-1.44591171104451,2.88069284127834,298.468447183325));
#2960=CARTESIAN_POINT('Ctrl Pts',(-1.36753443702595,2.91839738624888,298.463193249873));
#2961=CARTESIAN_POINT('Ctrl Pts',(-1.33775757184079,2.93216614456803,298.461196831334));
#2962=CARTESIAN_POINT('Ctrl Pts',(-1.27477687403119,2.96012924239569,298.456970696247));
#2963=CARTESIAN_POINT('Ctrl Pts',(-1.24153443779829,2.97422482085654,298.454738027793));
#2964=CARTESIAN_POINT('Ctrl Pts',(-1.1596124682817,3.00734895671664,298.449227872593));
#2965=CARTESIAN_POINT('Ctrl Pts',(-1.11069473316829,3.02575701848861,298.445930698259));
#2966=CARTESIAN_POINT('Ctrl Pts',(-1.00373266373073,3.06306420681997,298.438702423404));
#2967=CARTESIAN_POINT('Ctrl Pts',(-0.94555598457028,3.08151987491369,298.434759158993));
#2968=CARTESIAN_POINT('Ctrl Pts',(-0.764296860510881,3.13340538089995,298.422440913458));
#2969=CARTESIAN_POINT('Ctrl Pts',(-0.639734933850608,3.1611886328633,298.413925238229));
#2970=CARTESIAN_POINT('Ctrl Pts',(-0.317205756116933,3.21328203832322,298.391933079726));
#2971=CARTESIAN_POINT('Ctrl Pts',(-0.118015487143215,3.22674490844994,298.378388921139));
#2972=CARTESIAN_POINT('Ctrl Pts',(0.116922403576108,3.22082707674956,298.363201765964));
#2973=CARTESIAN_POINT('Ctrl Pts',(0.152677183535147,3.21933033795137,298.360912942984));
#2974=CARTESIAN_POINT('Ctrl Pts',(0.209686893482735,3.21599185352485,298.357306970387));
#2975=CARTESIAN_POINT('Ctrl Pts',(0.230960350489543,3.21453411412291,298.355971068119));
#2976=CARTESIAN_POINT('Ctrl Pts',(0.27345431084657,3.2111982254573,298.353324035055));
#2977=CARTESIAN_POINT('Ctrl Pts',(0.294673798092116,3.20932060006801,298.35201294946));
#2978=CARTESIAN_POINT('Ctrl Pts',(0.351372827070678,3.20373642872578,298.348534700757));
#2979=CARTESIAN_POINT('Ctrl Pts',(0.386813015016976,3.19965090167405,298.3463868294));
#2980=CARTESIAN_POINT('Ctrl Pts',(0.467055241463996,3.18904781164447,298.341568726853));
#2981=CARTESIAN_POINT('Ctrl Pts',(0.511802945558486,3.18217294500449,298.338913868008));
#2982=CARTESIAN_POINT('Ctrl Pts',(0.663536742366492,3.15557745095116,298.329976816981));
#2983=CARTESIAN_POINT('Ctrl Pts',(0.769667143674456,3.13138389696102,298.323835245966));
#2984=CARTESIAN_POINT('Ctrl Pts',(1.09182626101457,3.04057149360314,298.305021351661));
#2985=CARTESIAN_POINT('Ctrl Pts',(1.30220933664901,2.95658604124506,298.292444842921));
#2986=CARTESIAN_POINT('Ctrl Pts',(1.55160365214098,2.82520396911323,298.275847268083));
#2987=CARTESIAN_POINT('Ctrl Pts',(1.60044111024342,2.79782756224527,298.27251290614));
#2988=CARTESIAN_POINT('Ctrl Pts',(1.68013606286744,2.75038407921992,298.266915308918));
#2989=CARTESIAN_POINT('Ctrl Pts',(1.7114079881714,2.73103502392164,298.264677522831));
#2990=CARTESIAN_POINT('Ctrl Pts',(1.77301028584244,2.69144592487489,298.260182490146));
#2991=CARTESIAN_POINT('Ctrl Pts',(1.80334184377295,2.67121782427452,298.257925906087));
#2992=CARTESIAN_POINT('Ctrl Pts',(1.87793243713751,2.61962391437302,298.252264443833));
#2993=CARTESIAN_POINT('Ctrl Pts',(1.92175370357352,2.58764793539101,298.248837315161));
#2994=CARTESIAN_POINT('Ctrl Pts',(2.11960578197402,2.43547869585365,298.232881974063));
#2995=CARTESIAN_POINT('Ctrl Pts',(2.2632940852352,2.30255621012592,298.21987474582));
#2996=CARTESIAN_POINT('Ctrl Pts',(2.51863696368645,2.01921315438659,298.194175827212));
#2997=CARTESIAN_POINT('Ctrl Pts',(2.63102481851755,1.87042006772774,298.181553379709));
#2998=CARTESIAN_POINT('Ctrl Pts',(2.7495606857906,1.6814861753241,298.167123046619));
#2999=CARTESIAN_POINT('Ctrl Pts',(2.76863783192965,1.64988622025523,298.164759837543));
#3000=CARTESIAN_POINT('Ctrl Pts',(2.79798973231079,1.59932347695914,298.161065601027));
#3001=CARTESIAN_POINT('Ctrl Pts',(2.80862375159028,1.58057420227658,298.159714301926));
#3002=CARTESIAN_POINT('Ctrl Pts',(2.82927960006955,1.54328819588219,298.157065651632));
#3003=CARTESIAN_POINT('Ctrl Pts',(2.83930923909406,1.52475722600699,298.155767930978));
#3004=CARTESIAN_POINT('Ctrl Pts',(2.86532023960482,1.47555199424044,298.152367591886));
#3005=CARTESIAN_POINT('Ctrl Pts',(2.88099128038311,1.4447156190346,298.150282785567));
#3006=CARTESIAN_POINT('Ctrl Pts',(2.91521223602377,1.3746057788721,298.145632733273));
#3007=CARTESIAN_POINT('Ctrl Pts',(2.93347100913079,1.3351972120616,298.143081316996));
#3008=CARTESIAN_POINT('Ctrl Pts',(2.99157234195457,1.2028451150518,298.134680033881));
#3009=CARTESIAN_POINT('Ctrl Pts',(3.02783877354474,1.10839345233708,298.128953805258));
#3010=CARTESIAN_POINT('Ctrl Pts',(3.13288996364184,0.790911305705543,298.110133298698));
#3011=CARTESIAN_POINT('Ctrl Pts',(3.1819049131835,0.562150509798829,298.097193790661));
#3012=CARTESIAN_POINT('Ctrl Pts',(3.21164346314507,0.273348893061976,298.080131172405));
#3013=CARTESIAN_POINT('Ctrl Pts',(3.21597939596838,0.216447001981912,298.07673857764));
#3014=CARTESIAN_POINT('Ctrl Pts',(3.22027761091772,0.129686066079792,298.071503986356));
#3015=CARTESIAN_POINT('Ctrl Pts',(3.22133946752476,0.0998915044040692,298.06969537231));
#3016=CARTESIAN_POINT('Ctrl Pts',(3.22249863186971,0.0466034311486563,298.066439097593));
#3017=CARTESIAN_POINT('Ctrl Pts',(3.22275269597726,0.0231153400034857,298.064996338945));
#3018=CARTESIAN_POINT('Ctrl Pts',(3.22274997842995,-0.000372866926442411,
298.063545698078));
#3019=CARTESIAN_POINT('Ctrl Pts',(-1.47546400239267,-2.86515680899727,297.653713253152));
#3020=CARTESIAN_POINT('Ctrl Pts',(-1.3864988722017,-2.91097100201203,297.659873902062));
#3021=CARTESIAN_POINT('Ctrl Pts',(-1.295372951794,-2.9526505390965,297.666034550972));
#3022=CARTESIAN_POINT('Ctrl Pts',(-1.20250825355637,-2.98999857234562,297.672195199882));
#3023=CARTESIAN_POINT('Ctrl Pts',(-1.10964207451035,-3.02734720114161,297.678355947028));
#3024=CARTESIAN_POINT('Ctrl Pts',(-1.01503746431377,-3.06036402808895,297.684516694175));
#3025=CARTESIAN_POINT('Ctrl Pts',(-0.919135749817075,-3.0889006192994,297.690677441322));
#3026=CARTESIAN_POINT('Ctrl Pts',(-0.818267954305444,-3.11891492156627,
297.697157210601));
#3027=CARTESIAN_POINT('Ctrl Pts',(-0.715965614330064,-3.14397235708149,
297.70363697988));
#3028=CARTESIAN_POINT('Ctrl Pts',(-0.612757774231671,-3.16396040945816,
297.710116749159));
#3029=CARTESIAN_POINT('Ctrl Pts',(-0.514492453227045,-3.18299125421935,
297.71628620884));
#3030=CARTESIAN_POINT('Ctrl Pts',(-0.415406804278566,-3.19742702253057,
297.722455668521));
#3031=CARTESIAN_POINT('Ctrl Pts',(-0.315964162543643,-3.2072237543533,297.728625128201));
#3032=CARTESIAN_POINT('Ctrl Pts',(-0.216454009223977,-3.21702713717484,
297.734798776327));
#3033=CARTESIAN_POINT('Ctrl Pts',(-0.116586811851768,-3.22218519139546,
297.740972424452));
#3034=CARTESIAN_POINT('Ctrl Pts',(-0.0168268071893892,-3.22270607115508,
297.747146072578));
#3035=CARTESIAN_POINT('Ctrl Pts',(0.0830782578465212,-3.22322770832257,
297.753328697765));
#3036=CARTESIAN_POINT('Ctrl Pts',(0.182875388517365,-3.2190987360934,297.759511322952));
#3037=CARTESIAN_POINT('Ctrl Pts',(0.282104855435379,-3.21037916966825,297.765693948139));
#3038=CARTESIAN_POINT('Ctrl Pts',(0.296767485300708,-3.20909072401748,297.766607522983));
#3039=CARTESIAN_POINT('Ctrl Pts',(0.311417738880869,-3.20770213618914,297.767521097826));
#3040=CARTESIAN_POINT('Ctrl Pts',(0.326054153801449,-3.20621369395255,297.76843467267));
#3041=CARTESIAN_POINT('Ctrl Pts',(0.425105640416448,-3.19614070701722,297.77461726225));
#3042=CARTESIAN_POINT('Ctrl Pts',(0.523857142175329,-3.18145634053772,297.780799851831));
#3043=CARTESIAN_POINT('Ctrl Pts',(0.621846278658205,-3.16218670672985,297.786982441412));
#3044=CARTESIAN_POINT('Ctrl Pts',(0.71970621202586,-3.14294248080704,297.793156878968));
#3045=CARTESIAN_POINT('Ctrl Pts',(0.816805357319707,-3.11912508864679,297.799331316524));
#3046=CARTESIAN_POINT('Ctrl Pts',(0.912686224488411,-3.09081242040488,297.80550575408));
#3047=CARTESIAN_POINT('Ctrl Pts',(1.00846870967552,-3.06252880338548,297.811673856135));
#3048=CARTESIAN_POINT('Ctrl Pts',(1.1030349894859,-3.0297592034546,297.817841958189));
#3049=CARTESIAN_POINT('Ctrl Pts',(1.19593847430688,-2.99263240779293,297.824010060244));
#3050=CARTESIAN_POINT('Ctrl Pts',(1.28877726195373,-2.955531466907,297.830173866886));
#3051=CARTESIAN_POINT('Ctrl Pts',(1.37995515640695,-2.91407952363585,297.836337673528));
#3052=CARTESIAN_POINT('Ctrl Pts',(1.46904228340674,-2.86845469409281,297.84250148017));
#3053=CARTESIAN_POINT('Ctrl Pts',(1.55809772307698,-2.82284609280921,297.848663094413));
#3054=CARTESIAN_POINT('Ctrl Pts',(1.64506348851173,-2.77306775193101,297.854824708656));
#3055=CARTESIAN_POINT('Ctrl Pts',(1.72953200026501,-2.71934488849048,297.860986322898));
#3056=CARTESIAN_POINT('Ctrl Pts',(1.81399283656353,-2.66562690672005,297.86714737725));
#3057=CARTESIAN_POINT('Ctrl Pts',(1.89595650546268,-2.60796534743763,297.873308431601));
#3058=CARTESIAN_POINT('Ctrl Pts',(1.97504309248858,-2.54662960504922,297.879469485952));
#3059=CARTESIAN_POINT('Ctrl Pts',(2.05414343654389,-2.48528319337233,297.885631612012));
#3060=CARTESIAN_POINT('Ctrl Pts',(2.13036536272108,-2.42026159413796,297.891793738073));
#3061=CARTESIAN_POINT('Ctrl Pts',(2.20336160092606,-2.35187483044157,297.897955864133));
#3062=CARTESIAN_POINT('Ctrl Pts',(2.27643448021811,-2.28341626529294,297.904124460007));
#3063=CARTESIAN_POINT('Ctrl Pts',(2.34627459326325,-2.21158577753458,297.91029305588));
#3064=CARTESIAN_POINT('Ctrl Pts',(2.41257127322473,-2.13673054316889,297.916461651754));
#3065=CARTESIAN_POINT('Ctrl Pts',(2.47890577301725,-2.06183260662991,297.922633766586));
#3066=CARTESIAN_POINT('Ctrl Pts',(2.54169254259044,-1.98390682376247,297.928805881418));
#3067=CARTESIAN_POINT('Ctrl Pts',(2.60066226735119,-1.90333216588061,297.93497799625));
#3068=CARTESIAN_POINT('Ctrl Pts',(2.65972538334018,-1.82262990071729,297.941159885952));
#3069=CARTESIAN_POINT('Ctrl Pts',(2.71495914327061,-1.73927074331159,297.947341775654));
#3070=CARTESIAN_POINT('Ctrl Pts',(2.76613846154025,-1.65366126340546,297.953523665355));
#3071=CARTESIAN_POINT('Ctrl Pts',(2.79739767475446,-1.60137285715033,297.95729942898));
#3072=CARTESIAN_POINT('Ctrl Pts',(2.82714528212604,-1.5482454479238,297.961075192605));
#3073=CARTESIAN_POINT('Ctrl Pts',(2.8553387868184,-1.49437544646265,297.964850956229));
#3074=CARTESIAN_POINT('Ctrl Pts',(2.90406371299427,-1.40127556856774,297.971376352979));
#3075=CARTESIAN_POINT('Ctrl Pts',(2.94829409842913,-1.3056709537505,297.977901749728));
#3076=CARTESIAN_POINT('Ctrl Pts',(2.98778066801885,-1.20800837841169,297.984427146477));
#3077=CARTESIAN_POINT('Ctrl Pts',(3.02715878541849,-1.11061403909069,297.99093462084));
#3078=CARTESIAN_POINT('Ctrl Pts',(3.06181892203709,-1.01117333837293,297.997442095202));
#3079=CARTESIAN_POINT('Ctrl Pts',(3.09155861547018,-0.910155420580508,298.003949569565));
#3080=CARTESIAN_POINT('Ctrl Pts',(3.12124947881499,-0.809303365756907,298.010446359199));
#3081=CARTESIAN_POINT('Ctrl Pts',(3.14603588209779,-0.706879593528002,298.016943148833));
#3082=CARTESIAN_POINT('Ctrl Pts',(3.16576366259527,-0.603372186209608,298.023439938467));
#3083=CARTESIAN_POINT('Ctrl Pts',(3.18544680753346,-0.500098972039173,298.029922028635));
#3084=CARTESIAN_POINT('Ctrl Pts',(3.20009407460375,-0.39574736234028,298.036404118803));
#3085=CARTESIAN_POINT('Ctrl Pts',(3.20960157544718,-0.290818309923867,298.042886208972));
#3086=CARTESIAN_POINT('Ctrl Pts',(3.21834684883231,-0.194301542317404,298.048848622392));
#3087=CARTESIAN_POINT('Ctrl Pts',(3.22274391833166,-0.0972965918580311,
298.054811035813));
#3088=CARTESIAN_POINT('Ctrl Pts',(3.22274999369119,-0.000201651753011577,
298.060773449234));
#3089=CARTESIAN_POINT('Ctrl Pts',(-1.47546398584926,-2.86515681751659,297.410170442659));
#3090=CARTESIAN_POINT('Ctrl Pts',(-1.30851984510788,-2.95112770253292,297.421244654684));
#3091=CARTESIAN_POINT('Ctrl Pts',(-1.13433665046958,-3.02236604353812,297.431692562582));
#3092=CARTESIAN_POINT('Ctrl Pts',(-0.780905386326587,-3.13201051280962,
297.452458858485));
#3093=CARTESIAN_POINT('Ctrl Pts',(-0.602670515941956,-3.17113270153365,
297.462737748404));
#3094=CARTESIAN_POINT('Ctrl Pts',(-0.36765776902151,-3.20218057114698,297.476709960238));
#3095=CARTESIAN_POINT('Ctrl Pts',(-0.31304862087637,-3.20797953396451,297.479983403163));
#3096=CARTESIAN_POINT('Ctrl Pts',(-0.221646792429247,-3.21532951632577,
297.485520749532));
#3097=CARTESIAN_POINT('Ctrl Pts',(-0.184926767625853,-3.21765024839751,
297.487760958484));
#3098=CARTESIAN_POINT('Ctrl Pts',(-0.111162063892194,-3.22104540549316,
297.492296085474));
#3099=CARTESIAN_POINT('Ctrl Pts',(-0.0741225918464192,-3.22211051532846,
297.494590934589));
#3100=CARTESIAN_POINT('Ctrl Pts',(0.0193168099386926,-3.22318550257323,
297.50042767845));
#3101=CARTESIAN_POINT('Ctrl Pts',(0.0757121308366272,-3.22235395020963,
297.503994249201));
#3102=CARTESIAN_POINT('Ctrl Pts',(0.346136926652778,-3.21126382775852,297.521314803023));
#3103=CARTESIAN_POINT('Ctrl Pts',(0.558782943186501,-3.18115757680039,297.535642348083));
#3104=CARTESIAN_POINT('Ctrl Pts',(0.918787944819762,-3.09296315630843,297.56056829093));
#3105=CARTESIAN_POINT('Ctrl Pts',(1.06783819627523,-3.04472021935663,297.571082711752));
#3106=CARTESIAN_POINT('Ctrl Pts',(1.24620321896529,-2.9722709672623,297.583511944796));
#3107=CARTESIAN_POINT('Ctrl Pts',(1.27937469373764,-2.95814431683222,297.585816121074));
#3108=CARTESIAN_POINT('Ctrl Pts',(1.33202709175196,-2.93466995236105,297.589453917096));
#3109=CARTESIAN_POINT('Ctrl Pts',(1.35166232454172,-2.92567819884748,297.590806101317));
#3110=CARTESIAN_POINT('Ctrl Pts',(1.39077385678603,-2.90728965997207,297.593488464489));
#3111=CARTESIAN_POINT('Ctrl Pts',(1.41024883954537,-2.89789291529142,297.594818478245));
#3112=CARTESIAN_POINT('Ctrl Pts',(1.4625308623315,-2.8720147713772,297.598377589641));
#3113=CARTESIAN_POINT('Ctrl Pts',(1.49515427636117,-2.85516712469556,297.600586196206));
#3114=CARTESIAN_POINT('Ctrl Pts',(1.69584493983292,-2.74714133098956,297.614139594867));
#3115=CARTESIAN_POINT('Ctrl Pts',(1.85582581255376,-2.64170438231457,297.62481233139));
#3116=CARTESIAN_POINT('Ctrl Pts',(2.15696372202097,-2.40230149826316,297.646421192671));
#3117=CARTESIAN_POINT('Ctrl Pts',(2.29723812346219,-2.26853085700959,297.65732451832));
#3118=CARTESIAN_POINT('Ctrl Pts',(2.45954444485929,-2.08316157114292,297.671878148233));
#3119=CARTESIAN_POINT('Ctrl Pts',(2.49343526508803,-2.04247426454587,297.675040329777));
#3120=CARTESIAN_POINT('Ctrl Pts',(2.54890260773457,-1.97244453475001,297.680442309161));
#3121=CARTESIAN_POINT('Ctrl Pts',(2.57101250848631,-1.94353710118818,297.682660967959));
#3122=CARTESIAN_POINT('Ctrl Pts',(2.6122055521326,-1.88774630595666,297.68692520292));
#3123=CARTESIAN_POINT('Ctrl Pts',(2.6313750820318,-1.86093229718561,297.688967122066));
#3124=CARTESIAN_POINT('Ctrl Pts',(2.68097906322758,-1.78924790466129,297.694408671795));
#3125=CARTESIAN_POINT('Ctrl Pts',(2.71069724957047,-1.74389697792683,297.697833884215));
#3126=CARTESIAN_POINT('Ctrl Pts',(2.86656767873251,-1.49241625739937,297.716744568368));
#3127=CARTESIAN_POINT('Ctrl Pts',(2.97035410420162,-1.27337263094209,297.733001632057));
#3128=CARTESIAN_POINT('Ctrl Pts',(3.08147992048965,-0.949123700666557,297.756100300445));
#3129=CARTESIAN_POINT('Ctrl Pts',(3.10975813891146,-0.851915762275134,297.762897851485));
#3130=CARTESIAN_POINT('Ctrl Pts',(3.14358972444243,-0.711234154586975,297.772434921197));
#3131=CARTESIAN_POINT('Ctrl Pts',(3.15290514404828,-0.668730040466414,297.775277652372));
#3132=CARTESIAN_POINT('Ctrl Pts',(3.16809292173972,-0.592036316220455,297.7803234418));
#3133=CARTESIAN_POINT('Ctrl Pts',(3.17427939679768,-0.557916025582743,297.782538830892));
#3134=CARTESIAN_POINT('Ctrl Pts',(3.18335362306144,-0.502817295223105,297.786062140488));
#3135=CARTESIAN_POINT('Ctrl Pts',(3.18658727506148,-0.48189949120656,297.787387232875));
#3136=CARTESIAN_POINT('Ctrl Pts',(3.19269590812945,-0.439629922251756,297.790037676898));
#3137=CARTESIAN_POINT('Ctrl Pts',(3.1955633461254,-0.418278127082079,297.791362554702));
#3138=CARTESIAN_POINT('Ctrl Pts',(3.20277304752365,-0.360182199098518,297.794933427222));
#3139=CARTESIAN_POINT('Ctrl Pts',(3.20669714814887,-0.323388417396749,297.797158137567));
#3140=CARTESIAN_POINT('Ctrl Pts',(3.22623374077421,-0.104523251231982,297.810216194395));
#3141=CARTESIAN_POINT('Ctrl Pts',(3.22697258870022,0.078559510277362,297.820433044072));
#3142=CARTESIAN_POINT('Ctrl Pts',(3.19622541191419,0.457358281996847,297.841755255838));
#3143=CARTESIAN_POINT('Ctrl Pts',(3.16224788712159,0.652083027481734,297.852834716233));
#3144=CARTESIAN_POINT('Ctrl Pts',(3.09637610721237,0.895303617317299,297.867683841644));
#3145=CARTESIAN_POINT('Ctrl Pts',(3.08072445277333,0.947760463793996,297.870946278825));
#3146=CARTESIAN_POINT('Ctrl Pts',(3.05243690877041,1.03444439421292,297.876451838098));
#3147=CARTESIAN_POINT('Ctrl Pts',(3.04054179325477,1.06890211178701,297.878671016752));
#3148=CARTESIAN_POINT('Ctrl Pts',(3.01557161674428,1.13744342272423,297.883150610087));
#3149=CARTESIAN_POINT('Ctrl Pts',(3.00249683922268,1.17152135048366,297.885410743925));
#3150=CARTESIAN_POINT('Ctrl Pts',(2.96827952385552,1.25636700367486,297.891124136968));
#3151=CARTESIAN_POINT('Ctrl Pts',(2.94641169902695,1.30682779937892,297.894600848131));
#3152=CARTESIAN_POINT('Ctrl Pts',(2.82425710998779,1.57003236260474,297.913165277664));
#3153=CARTESIAN_POINT('Ctrl Pts',(2.70220846244861,1.77185395369853,297.928982119722));
#3154=CARTESIAN_POINT('Ctrl Pts',(2.4657745824985,2.08080916702227,297.955228105775));
#3155=CARTESIAN_POINT('Ctrl Pts',(2.36358216146528,2.19620096274597,297.965577804624));
#3156=CARTESIAN_POINT('Ctrl Pts',(2.23012892924665,2.32673883719612,297.977603991894));
#3157=CARTESIAN_POINT('Ctrl Pts',(2.20638459163562,2.34926709446119,297.979691748334));
#3158=CARTESIAN_POINT('Ctrl Pts',(2.16709529565289,2.38542292109452,297.983056780651));
#3159=CARTESIAN_POINT('Ctrl Pts',(2.15175551412132,2.39926922782389,297.984348995116));
#3160=CARTESIAN_POINT('Ctrl Pts',(2.11979539061685,2.42756461584974,297.986995296334));
#3161=CARTESIAN_POINT('Ctrl Pts',(2.10315832487625,2.44199254430847,297.98834801666));
#3162=CARTESIAN_POINT('Ctrl Pts',(2.05654892637634,2.4815832505092,297.992073599697));
#3163=CARTESIAN_POINT('Ctrl Pts',(2.02626329001173,2.5063731355181,297.994422131999));
#3164=CARTESIAN_POINT('Ctrl Pts',(1.83379911489679,2.65814247207678,298.008954389232));
#3165=CARTESIAN_POINT('Ctrl Pts',(1.66019443503162,2.76989411810704,298.020374493635));
#3166=CARTESIAN_POINT('Ctrl Pts',(1.33065379777891,2.93983428897944,298.041208192669));
#3167=CARTESIAN_POINT('Ctrl Pts',(1.17865120946816,3.00400392837138,298.050532628656));
#3168=CARTESIAN_POINT('Ctrl Pts',(0.967786311960895,3.07454480412374,298.063607085734));
#3169=CARTESIAN_POINT('Ctrl Pts',(0.912677883444726,3.09135157972572,298.067034476848));
#3170=CARTESIAN_POINT('Ctrl Pts',(0.821363761800754,3.11654574058412,298.072747166308));
#3171=CARTESIAN_POINT('Ctrl Pts',(0.785409786273584,3.12580022976907,298.075004817545));
#3172=CARTESIAN_POINT('Ctrl Pts',(0.714000112733848,3.14287115107033,298.079509081158));
#3173=CARTESIAN_POINT('Ctrl Pts',(0.678556272267247,3.15071364154695,298.081754497305));
#3174=CARTESIAN_POINT('Ctrl Pts',(0.590991197760881,3.1685426912215,298.087328865796));
#3175=CARTESIAN_POINT('Ctrl Pts',(0.538742812073637,3.17784345797606,298.090678454025));
#3176=CARTESIAN_POINT('Ctrl Pts',(0.424724139071017,3.19524737004199,298.098042776611));
#3177=CARTESIAN_POINT('Ctrl Pts',(0.362901179433595,3.20285783442598,298.102070491835));
#3178=CARTESIAN_POINT('Ctrl Pts',(0.169073936717036,3.22103436448897,298.114801315828));
#3179=CARTESIAN_POINT('Ctrl Pts',(0.0366216376400551,3.22526003050917,298.123655730661));
#3180=CARTESIAN_POINT('Ctrl Pts',(-0.284359912647403,3.21572371645284,298.145280995186));
#3181=CARTESIAN_POINT('Ctrl Pts',(-0.4721687516899,3.1935568241037,298.158085124294));
#3182=CARTESIAN_POINT('Ctrl Pts',(-0.69295846235032,3.14758283540607,298.172672001631));
#3183=CARTESIAN_POINT('Ctrl Pts',(-0.728821117846843,3.13947275392857,298.175025421685));
#3184=CARTESIAN_POINT('Ctrl Pts',(-0.785484913247391,3.12563528227853,298.178710394452));
#3185=CARTESIAN_POINT('Ctrl Pts',(-0.806379864384549,3.1203099272178,298.180061946459));
#3186=CARTESIAN_POINT('Ctrl Pts',(-0.847686556701125,3.10933971580286,298.182717178185));
#3187=CARTESIAN_POINT('Ctrl Pts',(-0.868099084774921,3.10370262601329,298.184021132953));
#3188=CARTESIAN_POINT('Ctrl Pts',(-0.922053377912032,3.08822875217649,298.187449562523));
#3189=CARTESIAN_POINT('Ctrl Pts',(-0.955494211869299,3.07804650530772,298.189555776803));
#3190=CARTESIAN_POINT('Ctrl Pts',(-1.14270937817302,3.01769689838389,298.20127542487));
#3191=CARTESIAN_POINT('Ctrl Pts',(-1.29271726027755,2.95654738589552,298.210398728571));
#3192=CARTESIAN_POINT('Ctrl Pts',(-1.63260663900358,2.78715428852557,298.231733711671));
#3193=CARTESIAN_POINT('Ctrl Pts',(-1.81731648951552,2.67039040889286,298.243891905099));
#3194=CARTESIAN_POINT('Ctrl Pts',(-2.03352108400273,2.50082714888708,298.260059563738));
#3195=CARTESIAN_POINT('Ctrl Pts',(-2.07728277742612,2.46459735513104,298.263441222975));
#3196=CARTESIAN_POINT('Ctrl Pts',(-2.14789787377132,2.40291868700456,298.269097808159));
#3197=CARTESIAN_POINT('Ctrl Pts',(-2.1753121492951,2.37812959574368,298.271346184632));
#3198=CARTESIAN_POINT('Ctrl Pts',(-2.22885849330394,2.32801017324282,298.275847074358));
#3199=CARTESIAN_POINT('Ctrl Pts',(-2.2549998534883,2.30269777472373,298.278098656237));
#3200=CARTESIAN_POINT('Ctrl Pts',(-2.31861487115342,2.2389777842165,298.283717402327));
#3201=CARTESIAN_POINT('Ctrl Pts',(-2.35556742763593,2.20006772484594,298.287106007648));
#3202=CARTESIAN_POINT('Ctrl Pts',(-2.52214717193582,2.01565412337334,298.302983058208));
#3203=CARTESIAN_POINT('Ctrl Pts',(-2.63936266769136,1.85952485963476,298.315949635673));
#3204=CARTESIAN_POINT('Ctrl Pts',(-2.84065140844619,1.53369778463225,298.341751046986));
#3205=CARTESIAN_POINT('Ctrl Pts',(-2.92534777304943,1.36523943220443,298.354519439996));
#3206=CARTESIAN_POINT('Ctrl Pts',(-3.00846715461208,1.15611405673199,298.369077942086));
#3207=CARTESIAN_POINT('Ctrl Pts',(-3.02148498959266,1.12165192923532,298.371436309191));
#3208=CARTESIAN_POINT('Ctrl Pts',(-3.04117983742346,1.06668054304194,298.375125835033));
#3209=CARTESIAN_POINT('Ctrl Pts',(-3.04824643673452,1.04631539520742,298.376477149375));
#3210=CARTESIAN_POINT('Ctrl Pts',(-3.06183137034291,1.00585897168002,298.379128831305));
#3211=CARTESIAN_POINT('Ctrl Pts',(-3.06835753176477,0.985771633100665,298.380429523657));
#3212=CARTESIAN_POINT('Ctrl Pts',(-3.08509886150542,0.932464666899898,298.38384281159));
#3213=CARTESIAN_POINT('Ctrl Pts',(-3.0949752756659,0.899140478698359,298.385937383));
#3214=CARTESIAN_POINT('Ctrl Pts',(-3.116048569681,0.823570460619718,298.390612683482));
#3215=CARTESIAN_POINT('Ctrl Pts',(-3.12692924982858,0.781243106843752,298.393179369342));
#3216=CARTESIAN_POINT('Ctrl Pts',(-3.16036602137312,0.63925240449213,298.401655807293));
#3217=CARTESIAN_POINT('Ctrl Pts',(-3.17904434828389,0.538735869891413,298.407439656722));
#3218=CARTESIAN_POINT('Ctrl Pts',(-3.22541621195218,0.200307297151154,298.426660769588));
#3219=CARTESIAN_POINT('Ctrl Pts',(-3.23138419072083,-0.0397437242021221,
298.439944322083));
#3220=CARTESIAN_POINT('Ctrl Pts',(-3.20602491621992,-0.332378027677306,
298.457263953187));
#3221=CARTESIAN_POINT('Ctrl Pts',(-3.19996455386814,-0.386390046878018,
298.460504720139));
#3222=CARTESIAN_POINT('Ctrl Pts',(-3.18805517551508,-0.472758488642186,
298.465770884098));
#3223=CARTESIAN_POINT('Ctrl Pts',(-3.18307151732941,-0.505224688292369,
298.467769591033));
#3224=CARTESIAN_POINT('Ctrl Pts',(-3.17156988229157,-0.573206376989585,
298.471997781393));
#3225=CARTESIAN_POINT('Ctrl Pts',(-3.16494954199224,-0.608699680032584,
298.474230177923));
#3226=CARTESIAN_POINT('Ctrl Pts',(-3.14730928595423,-0.69518557451247,298.479733833854));
#3227=CARTESIAN_POINT('Ctrl Pts',(-3.13564511615684,-0.746034807224774,
298.483024652436));
#3228=CARTESIAN_POINT('Ctrl Pts',(-3.10770952174123,-0.855548413743614,
298.490235642101));
#3229=CARTESIAN_POINT('Ctrl Pts',(-3.09099979309789,-0.914079377243734,
298.494167863774));
#3230=CARTESIAN_POINT('Ctrl Pts',(-3.03438304962176,-1.09303544343262,298.506429810837));
#3231=CARTESIAN_POINT('Ctrl Pts',(-2.98901868785504,-1.21159799003507,298.514898806429));
#3232=CARTESIAN_POINT('Ctrl Pts',(-2.85413239354378,-1.51007713582641,298.536946003867));
#3233=CARTESIAN_POINT('Ctrl Pts',(-2.75456388262891,-1.68487149835763,298.550597419637));
#3234=CARTESIAN_POINT('Ctrl Pts',(-2.61893242225138,-1.87845142726865,298.565869911451));
#3235=CARTESIAN_POINT('Ctrl Pts',(-2.59800598775317,-1.90728915540127,298.568148494384));
#3236=CARTESIAN_POINT('Ctrl Pts',(-2.56381318681165,-1.95280132526904,298.571742652846));
#3237=CARTESIAN_POINT('Ctrl Pts',(-2.55085278833936,-1.96970078607938,298.573076783023));
#3238=CARTESIAN_POINT('Ctrl Pts',(-2.52456211832076,-2.00328723034336,298.575725304862));
#3239=CARTESIAN_POINT('Ctrl Pts',(-2.51123160167491,-2.01997265281993,298.577039578494));
#3240=CARTESIAN_POINT('Ctrl Pts',(-2.47506274321663,-2.06433265720713,298.580533424514));
#3241=CARTESIAN_POINT('Ctrl Pts',(-2.45192585144059,-2.09176116182084,298.582693419418));
#3242=CARTESIAN_POINT('Ctrl Pts',(-2.32434259954537,-2.23798308577702,298.594242181843));
#3243=CARTESIAN_POINT('Ctrl Pts',(-2.21170583475831,-2.34936255906779,298.603168933322));
#3244=CARTESIAN_POINT('Ctrl Pts',(-1.92370770487942,-2.59499608423301,298.624435806898));
#3245=CARTESIAN_POINT('Ctrl Pts',(-1.74187899374605,-2.72038677972278,298.636716250659));
#3246=CARTESIAN_POINT('Ctrl Pts',(-1.5244468743339,-2.83953225480568,298.65130727442));
#3247=CARTESIAN_POINT('Ctrl Pts',(-1.50003654230719,-2.85250273788423,298.65294329802));
#3248=CARTESIAN_POINT('Ctrl Pts',(-1.47546399981363,-2.86515681032539,298.654589343883));
#3249=CARTESIAN_POINT('Origin',(0.,0.,294.689226550727));
#3250=CARTESIAN_POINT('',(-1.47546414420613,-2.86515673596787,300.152134095017));
#3251=CARTESIAN_POINT('',(-1.47546400147781,-2.86515680946839,299.907672586636));
#3252=CARTESIAN_POINT('',(-1.47546400239267,-2.86515680899727,294.689226550727));
#3253=CARTESIAN_POINT('Ctrl Pts',(-1.47546414420613,-2.86515673596787,300.152134095017));
#3254=CARTESIAN_POINT('Ctrl Pts',(-1.563549486761,-2.81979559989518,300.145496287807));
#3255=CARTESIAN_POINT('Ctrl Pts',(-1.64953114565584,-2.77037847724467,300.138924810279));
#3256=CARTESIAN_POINT('Ctrl Pts',(-1.76162338783503,-2.69887806569273,300.130351539397));
#3257=CARTESIAN_POINT('Ctrl Pts',(-1.78983046673973,-2.68025500284619,300.128193764278));
#3258=CARTESIAN_POINT('Ctrl Pts',(-1.83501423321666,-2.64939199023005,300.12474317954));
#3259=CARTESIAN_POINT('Ctrl Pts',(-1.85217332908825,-2.6374247270353,300.123434192876));
#3260=CARTESIAN_POINT('Ctrl Pts',(-1.88693843929308,-2.61267185608773,300.120786978898));
#3261=CARTESIAN_POINT('Ctrl Pts',(-1.90453376442025,-2.59987347830767,300.119449622142));
#3262=CARTESIAN_POINT('Ctrl Pts',(-1.95241894567294,-2.56429601269393,300.115812788393));
#3263=CARTESIAN_POINT('Ctrl Pts',(-1.98243962186252,-2.54115863340587,300.113535800539));
#3264=CARTESIAN_POINT('Ctrl Pts',(-2.14951247820355,-2.40762977437996,300.100837667517));
#3265=CARTESIAN_POINT('Ctrl Pts',(-2.27776360346689,-2.28667682631798,300.090977860896));
#3266=CARTESIAN_POINT('Ctrl Pts',(-2.53433845332124,-2.00157899001737,300.069450944227));
#3267=CARTESIAN_POINT('Ctrl Pts',(-2.65793109500705,-1.83427957220254,300.057806916586));
#3268=CARTESIAN_POINT('Ctrl Pts',(-2.79154219304184,-1.61126113042641,300.042450629321));
#3269=CARTESIAN_POINT('Ctrl Pts',(-2.81740177257449,-1.56560436968607,300.039317341756));
#3270=CARTESIAN_POINT('Ctrl Pts',(-2.85917251929353,-1.48746636985305,300.033960187568));
#3271=CARTESIAN_POINT('Ctrl Pts',(-2.87567275551391,-1.45531087345991,300.03175709769));
#3272=CARTESIAN_POINT('Ctrl Pts',(-2.90609608074538,-1.39348373611918,300.027520647675));
#3273=CARTESIAN_POINT('Ctrl Pts',(-2.92011419249179,-1.36386375146938,300.025490874761));
#3274=CARTESIAN_POINT('Ctrl Pts',(-2.95601117012331,-1.2849227275657,300.020078405565));
#3275=CARTESIAN_POINT('Ctrl Pts',(-2.9771065537306,-1.23525886905161,300.01667022153));
#3276=CARTESIAN_POINT('Ctrl Pts',(-3.0860306350114,-0.959803749766988,299.997740352056));
#3277=CARTESIAN_POINT('Ctrl Pts',(-3.14941701326185,-0.725220753789514,
299.981438264264));
#3278=CARTESIAN_POINT('Ctrl Pts',(-3.20112953441015,-0.386084907233361,
299.958316330828));
#3279=CARTESIAN_POINT('Ctrl Pts',(-3.21164531612068,-0.285706254992559,
299.951538956968));
#3280=CARTESIAN_POINT('Ctrl Pts',(-3.21992549833164,-0.141697775911958,
299.942031008696));
#3281=CARTESIAN_POINT('Ctrl Pts',(-3.22154088859554,-0.0983519814407669,
299.939197208208));
#3282=CARTESIAN_POINT('Ctrl Pts',(-3.22287046550643,-0.0204348434260564,
299.934167902587));
#3283=CARTESIAN_POINT('Ctrl Pts',(-3.22290433428755,0.0141241285302486,
299.931960074034));
#3284=CARTESIAN_POINT('Ctrl Pts',(-3.2220640859195,0.069746261029314,299.928450272112));
#3285=CARTESIAN_POINT('Ctrl Pts',(-3.22153921348952,0.090811243855519,299.927131146703));
#3286=CARTESIAN_POINT('Ctrl Pts',(-3.22005911864908,0.133423949830002,299.92448510169));
#3287=CARTESIAN_POINT('Ctrl Pts',(-3.21909412676297,0.154970130628407,299.923158720442));
#3288=CARTESIAN_POINT('Ctrl Pts',(-3.21588799795303,0.213421747348317,299.919587880599));
#3289=CARTESIAN_POINT('Ctrl Pts',(-3.21322791576597,0.250301968630703,299.917364562014));
#3290=CARTESIAN_POINT('Ctrl Pts',(-3.19352090477777,0.470614060514461,299.904218151561));
#3291=CARTESIAN_POINT('Ctrl Pts',(-3.1614042244661,0.652373624564809,299.893919936405));
#3292=CARTESIAN_POINT('Ctrl Pts',(-3.06192985806229,1.02538999835319,299.872253119217));
#3293=CARTESIAN_POINT('Ctrl Pts',(-2.99174081178703,1.21503727103232,299.860908909247));
#3294=CARTESIAN_POINT('Ctrl Pts',(-2.88170607968123,1.44381488041093,299.845908540881));
#3295=CARTESIAN_POINT('Ctrl Pts',(-2.85799253603054,1.49020453495757,299.842796556796));
#3296=CARTESIAN_POINT('Ctrl Pts',(-2.81597149556612,1.56771286593709,299.837464637358));
#3297=CARTESIAN_POINT('Ctrl Pts',(-2.79824614955375,1.59913646066605,299.835264998874));
#3298=CARTESIAN_POINT('Ctrl Pts',(-2.76338845158233,1.65857766393129,299.831027717092));
#3299=CARTESIAN_POINT('Ctrl Pts',(-2.74634799214967,1.68664405945773,299.828993535283));
#3300=CARTESIAN_POINT('Ctrl Pts',(-2.69996709038672,1.76046856764238,299.823550877854));
#3301=CARTESIAN_POINT('Ctrl Pts',(-2.66989378311293,1.80575150388964,299.820116373342));
#3302=CARTESIAN_POINT('Ctrl Pts',(-2.50131178302599,2.04617078075428,299.801344330845));
#3303=CARTESIAN_POINT('Ctrl Pts',(-2.34255822436219,2.22615411049026,299.785249657016));
#3304=CARTESIAN_POINT('Ctrl Pts',(-2.08965513658444,2.4555884531845,299.762232128189));
#3305=CARTESIAN_POINT('Ctrl Pts',(-2.010692449144,2.52065289047428,299.755358988234));
#3306=CARTESIAN_POINT('Ctrl Pts',(-1.89374977880329,2.60801453812505,299.745734560329));
#3307=CARTESIAN_POINT('Ctrl Pts',(-1.85820267959273,2.63345992915296,299.742877762231));
#3308=CARTESIAN_POINT('Ctrl Pts',(-1.79348007142165,2.67782650298746,299.737812441977));
#3309=CARTESIAN_POINT('Ctrl Pts',(-1.76449535217294,2.69701351888333,299.735591350453));
#3310=CARTESIAN_POINT('Ctrl Pts',(-1.71741506140514,2.72709529286136,299.732065831359));
#3311=CARTESIAN_POINT('Ctrl Pts',(-1.69951356148575,2.73828722986786,299.730743991563));
#3312=CARTESIAN_POINT('Ctrl Pts',(-1.66314479238028,2.76053075317411,299.728098049811));
#3313=CARTESIAN_POINT('Ctrl Pts',(-1.64467431508814,2.77157484058304,299.726774401516));
#3314=CARTESIAN_POINT('Ctrl Pts',(-1.59437233794269,2.80097203737478,299.723219960756));
#3315=CARTESIAN_POINT('Ctrl Pts',(-1.5623344686675,2.81896767743382,299.721009978234));
#3316=CARTESIAN_POINT('Ctrl Pts',(-1.3634378249976,2.92625488243654,299.707574915214));
#3317=CARTESIAN_POINT('Ctrl Pts',(-1.18927260801748,3.00126251697006,299.697012333321));
#3318=CARTESIAN_POINT('Ctrl Pts',(-0.823891189572074,3.1217824710916,299.675417485551));
#3319=CARTESIAN_POINT('Ctrl Pts',(-0.633101254567623,3.16599042953249,299.664415182304));
#3320=CARTESIAN_POINT('Ctrl Pts',(-0.387113354978648,3.1998525398595,299.649753894847));
#3321=CARTESIAN_POINT('Ctrl Pts',(-0.334568009085671,3.2057724199353,299.646597359688));
#3322=CARTESIAN_POINT('Ctrl Pts',(-0.245830945727075,3.21356436499495,299.641212613135));
#3323=CARTESIAN_POINT('Ctrl Pts',(-0.209709336233353,3.21612353835702,299.639005705586));
#3324=CARTESIAN_POINT('Ctrl Pts',(-0.1365482459055,3.22006917627843,299.634502048397));
#3325=CARTESIAN_POINT('Ctrl Pts',(-0.099512736678044,3.22142638592084,299.632204748356));
#3326=CARTESIAN_POINT('Ctrl Pts',(-0.00492897176134279,3.22325994949287,
299.62628996061));
#3327=CARTESIAN_POINT('Ctrl Pts',(0.0526217259274038,3.22283404611002,299.622645736504));
#3328=CARTESIAN_POINT('Ctrl Pts',(0.268206813217654,3.21546279294993,299.608817630297));
#3329=CARTESIAN_POINT('Ctrl Pts',(0.425654946869618,3.19842818758335,299.598347706023));
#3330=CARTESIAN_POINT('Ctrl Pts',(0.733662774720013,3.14195527748034,299.577317690514));
#3331=CARTESIAN_POINT('Ctrl Pts',(0.883910983267427,3.1030382457499,299.566792395836));
#3332=CARTESIAN_POINT('Ctrl Pts',(1.08234425028818,3.03605184173366,299.552876924668));
#3333=CARTESIAN_POINT('Ctrl Pts',(1.13346555452356,3.01733927063249,299.54929196399));
#3334=CARTESIAN_POINT('Ctrl Pts',(1.22205946120328,2.98234049843804,299.543105859657));
#3335=CARTESIAN_POINT('Ctrl Pts',(1.25974181782351,2.96662014274287,299.540483377253));
#3336=CARTESIAN_POINT('Ctrl Pts',(1.3175742873062,2.94119277749597,299.536482933941));
#3337=CARTESIAN_POINT('Ctrl Pts',(1.33793800893872,2.93198548907836,299.535079080511));
#3338=CARTESIAN_POINT('Ctrl Pts',(1.37661715070186,2.91401012489106,299.532423990696));
#3339=CARTESIAN_POINT('Ctrl Pts',(1.39494812330703,2.90527959748838,299.531170861429));
#3340=CARTESIAN_POINT('Ctrl Pts',(1.44159602572989,2.88251922051468,299.527992508266));
#3341=CARTESIAN_POINT('Ctrl Pts',(1.46979219288063,2.86824462617599,299.526081320729));
#3342=CARTESIAN_POINT('Ctrl Pts',(1.59676684173781,2.80159817281276,299.517499904559));
#3343=CARTESIAN_POINT('Ctrl Pts',(1.69299742679754,2.74451835174352,299.511064880895));
#3344=CARTESIAN_POINT('Ctrl Pts',(1.94642259942879,2.57578463469648,299.493791646811));
#3345=CARTESIAN_POINT('Ctrl Pts',(2.09687462939088,2.45486161550592,299.483148183455));
#3346=CARTESIAN_POINT('Ctrl Pts',(2.28932495904262,2.26950805608279,299.46788553351));
#3347=CARTESIAN_POINT('Ctrl Pts',(2.34120869852717,2.21594594865832,299.4635812));
#3348=CARTESIAN_POINT('Ctrl Pts',(2.43172984129206,2.1157657190864,299.455660706836));
#3349=CARTESIAN_POINT('Ctrl Pts',(2.47100016999023,2.06976619079909,299.452069816462));
#3350=CARTESIAN_POINT('Ctrl Pts',(2.53255683337475,1.99341114157365,299.446162602071));
#3351=CARTESIAN_POINT('Ctrl Pts',(2.55564695804178,1.96372109514022,299.443878140299));
#3352=CARTESIAN_POINT('Ctrl Pts',(2.59948181126903,1.9052739002946,299.439400951123));
#3353=CARTESIAN_POINT('Ctrl Pts',(2.62028202517081,1.87656502013045,299.437210796515));
#3354=CARTESIAN_POINT('Ctrl Pts',(2.66952716259211,1.80618044168319,299.431859886711));
#3355=CARTESIAN_POINT('Ctrl Pts',(2.69747440717476,1.76416961563188,299.428681354976));
#3356=CARTESIAN_POINT('Ctrl Pts',(2.81349638678403,1.5805571182932,299.414846469962));
#3357=CARTESIAN_POINT('Ctrl Pts',(2.89148340255457,1.43291071217499,299.403846177885));
#3358=CARTESIAN_POINT('Ctrl Pts',(3.02127957829406,1.13297075735029,299.381919913077));
#3359=CARTESIAN_POINT('Ctrl Pts',(3.07382850959044,0.981494700323993,299.371041239186));
#3360=CARTESIAN_POINT('Ctrl Pts',(3.12907985012651,0.773324692873389,299.356723720829));
#3361=CARTESIAN_POINT('Ctrl Pts',(3.14188151554877,0.719550503793197,299.353081631265));
#3362=CARTESIAN_POINT('Ctrl Pts',(3.16181781622192,0.625083570764121,299.346809126808));
#3363=CARTESIAN_POINT('Ctrl Pts',(3.16956495888623,0.584533744754777,299.344156608327));
#3364=CARTESIAN_POINT('Ctrl Pts',(3.18031758487748,0.52172890128881,299.340120865111));
#3365=CARTESIAN_POINT('Ctrl Pts',(3.18387295720959,0.499573865566821,299.338711063671));
#3366=CARTESIAN_POINT('Ctrl Pts',(3.19019780197776,0.457346692858114,299.336052601732));
#3367=CARTESIAN_POINT('Ctrl Pts',(3.19300984291246,0.437282716274429,299.334801915709));
#3368=CARTESIAN_POINT('Ctrl Pts',(3.19969069695675,0.386108449562979,299.331641011643));
#3369=CARTESIAN_POINT('Ctrl Pts',(3.20329524089861,0.354964864261157,299.32974450534));
#3370=CARTESIAN_POINT('Ctrl Pts',(3.21722622669429,0.217000837729855,299.321443630263));
#3371=CARTESIAN_POINT('Ctrl Pts',(3.22266871063748,0.109747374945496,299.31525530431));
#3372=CARTESIAN_POINT('Ctrl Pts',(3.22288674166129,-0.181375703593998,299.298715214201));
#3373=CARTESIAN_POINT('Ctrl Pts',(3.20730257840436,-0.364840062766869,299.288552665414));
#3374=CARTESIAN_POINT('Ctrl Pts',(3.15638739802366,-0.66103328564887,299.271451557693));
#3375=CARTESIAN_POINT('Ctrl Pts',(3.13037423414779,-0.774919255549078,299.264707235851));
#3376=CARTESIAN_POINT('Ctrl Pts',(3.08647928354816,-0.928218343966984,299.255240031375));
#3377=CARTESIAN_POINT('Ctrl Pts',(3.07390056120917,-0.969060757186082,299.252679554835));
#3378=CARTESIAN_POINT('Ctrl Pts',(3.04939183864144,-1.04335388392142,299.247944822355));
#3379=CARTESIAN_POINT('Ctrl Pts',(3.03771380356277,-1.0768809623489,299.245778857995));
#3380=CARTESIAN_POINT('Ctrl Pts',(3.01256079215715,-1.14542676452772,299.241286740243));
#3381=CARTESIAN_POINT('Ctrl Pts',(2.99902339712373,-1.18041665407409,299.238958823198));
#3382=CARTESIAN_POINT('Ctrl Pts',(2.96226460620396,-1.27070964415948,299.232856992934));
#3383=CARTESIAN_POINT('Ctrl Pts',(2.93810554754108,-1.32561293042703,299.229052883889));
#3384=CARTESIAN_POINT('Ctrl Pts',(2.88087507068635,-1.44641221240006,299.22046718668));
#3385=CARTESIAN_POINT('Ctrl Pts',(2.84704655955309,-1.51191075251473,299.215663519429));
#3386=CARTESIAN_POINT('Ctrl Pts',(2.71932021150384,-1.73970033067975,299.198440382127));
#3387=CARTESIAN_POINT('Ctrl Pts',(2.61354781484821,-1.89489278614232,299.185718988243));
#3388=CARTESIAN_POINT('Ctrl Pts',(2.42001534349954,-2.13158114860275,299.165179933183));
#3389=CARTESIAN_POINT('Ctrl Pts',(2.34013868835361,-2.21897910523336,299.157306944371));
#3390=CARTESIAN_POINT('Ctrl Pts',(2.23288762038897,-2.32407924762077,299.147646430006));
#3391=CARTESIAN_POINT('Ctrl Pts',(2.2098149912666,-2.34602842138877,299.145617527318));
#3392=CARTESIAN_POINT('Ctrl Pts',(2.17147316854219,-2.38143565090629,299.142331161196));
#3393=CARTESIAN_POINT('Ctrl Pts',(2.15639543694034,-2.39509713471953,299.141059786481));
#3394=CARTESIAN_POINT('Ctrl Pts',(2.12454903300024,-2.42340765088651,299.138419682113));
#3395=CARTESIAN_POINT('Ctrl Pts',(2.10775620636334,-2.43802729191267,299.137052921841));
#3396=CARTESIAN_POINT('Ctrl Pts',(2.06006401347751,-2.47868644423725,299.133237660296));
#3397=CARTESIAN_POINT('Ctrl Pts',(2.02882352182033,-2.50432139946177,299.130815467557));
#3398=CARTESIAN_POINT('Ctrl Pts',(1.95499372939945,-2.56261513874834,299.125245815627));
#3399=CARTESIAN_POINT('Ctrl Pts',(1.91205384335592,-2.59481164683851,299.122121803894));
#3400=CARTESIAN_POINT('Ctrl Pts',(1.74571765018845,-2.71315885429767,299.110369589579));
#3401=CARTESIAN_POINT('Ctrl Pts',(1.61714226009152,-2.791704911298,299.101986996676));
#3402=CARTESIAN_POINT('Ctrl Pts',(1.33778419675828,-2.93656424592635,299.084304194234));
#3403=CARTESIAN_POINT('Ctrl Pts',(1.18647494667525,-3.00089094599694,299.075010857996));
#3404=CARTESIAN_POINT('Ctrl Pts',(0.976417839463468,-3.07181319257301,299.061974038049));
#3405=CARTESIAN_POINT('Ctrl Pts',(0.9214235382365,-3.08875479156811,299.05855074832));
#3406=CARTESIAN_POINT('Ctrl Pts',(0.830313110490968,-3.11417259575874,299.052846266156));
#3407=CARTESIAN_POINT('Ctrl Pts',(0.794450742439805,-3.12351383264113,299.050592694904));
#3408=CARTESIAN_POINT('Ctrl Pts',(0.723241526182453,-3.14075636737339,299.046097978202));
#3409=CARTESIAN_POINT('Ctrl Pts',(0.687906730818511,-3.14868433279057,299.043858047684));
#3410=CARTESIAN_POINT('Ctrl Pts',(0.600663306123015,-3.16672027545137,299.038300921395));
#3411=CARTESIAN_POINT('Ctrl Pts',(0.548626613046161,-3.17614893122665,299.034963245026));
#3412=CARTESIAN_POINT('Ctrl Pts',(0.303097695713372,-3.21442323295909,299.019098206603));
#3413=CARTESIAN_POINT('Ctrl Pts',(0.107496798203785,-3.22688845579623,299.006085787622));
#3414=CARTESIAN_POINT('Ctrl Pts',(-0.276994704810866,-3.21638578880807,
298.980175479974));
#3415=CARTESIAN_POINT('Ctrl Pts',(-0.465180787409814,-3.19460161136501,
298.967344848395));
#3416=CARTESIAN_POINT('Ctrl Pts',(-0.686377900808624,-3.14902425866946,
298.952735368959));
#3417=CARTESIAN_POINT('Ctrl Pts',(-0.722247728320832,-3.14099138520554,
298.950382314337));
#3418=CARTESIAN_POINT('Ctrl Pts',(-0.778892041586941,-3.12728443526204,
298.946700139958));
#3419=CARTESIAN_POINT('Ctrl Pts',(-0.799759603834225,-3.12201303458973,
298.945350957575));
#3420=CARTESIAN_POINT('Ctrl Pts',(-0.840987293683504,-3.11115791119713,
298.94270204384));
#3421=CARTESIAN_POINT('Ctrl Pts',(-0.861348332266915,-3.10558243687959,
298.941402004251));
#3422=CARTESIAN_POINT('Ctrl Pts',(-0.915074949881425,-3.09030139989273,
298.937989748997));
#3423=CARTESIAN_POINT('Ctrl Pts',(-0.948341854935828,-3.08025532207555,
298.93589555004));
#3424=CARTESIAN_POINT('Ctrl Pts',(-1.02305920641151,-3.05636655722115,298.931220797139));
#3425=CARTESIAN_POINT('Ctrl Pts',(-1.06440411298453,-3.0422147999709,298.928654282202));
#3426=CARTESIAN_POINT('Ctrl Pts',(-1.20143690815107,-2.99217462264578,298.920177123254));
#3427=CARTESIAN_POINT('Ctrl Pts',(-1.29570768167465,-2.95257573994885,298.914392369835));
#3428=CARTESIAN_POINT('Ctrl Pts',(-1.4173446430655,-2.8945315868833,298.90680829297));
#3429=CARTESIAN_POINT('Ctrl Pts',(-1.44652186378979,-2.88006108465439,298.904979765819));
#3430=CARTESIAN_POINT('Ctrl Pts',(-1.47546409036594,-2.86515676369385,298.903152516993));
#3431=CARTESIAN_POINT('',(3.22274998327137,0.000328366225831933,299.061455114234));
#3432=CARTESIAN_POINT('Ctrl Pts',(-1.47546399981363,-2.86515681032539,298.654589343883));
#3433=CARTESIAN_POINT('Ctrl Pts',(-1.44972727176912,-2.8784104010419,298.656313375279));
#3434=CARTESIAN_POINT('Ctrl Pts',(-1.42381259905786,-2.89131688948619,298.6580484028));
#3435=CARTESIAN_POINT('Ctrl Pts',(-1.36446682477198,-2.91988191139373,298.662022252458));
#3436=CARTESIAN_POINT('Ctrl Pts',(-1.33093520187307,-2.93531794016742,298.66426797716));
#3437=CARTESIAN_POINT('Ctrl Pts',(-1.26382007437086,-2.96482744453382,298.668767485804));
#3438=CARTESIAN_POINT('Ctrl Pts',(-1.23024850074144,-2.97891446896464,298.671020406907));
#3439=CARTESIAN_POINT('Ctrl Pts',(-1.14648503000512,-3.01240515599955,298.676650214486));
#3440=CARTESIAN_POINT('Ctrl Pts',(-1.09603361673257,-3.03112561855672,298.68004875204));
#3441=CARTESIAN_POINT('Ctrl Pts',(-0.868060424748604,-3.1092814454528,298.695447848269));
#3442=CARTESIAN_POINT('Ctrl Pts',(-0.686052861443158,-3.15443713918839,
298.707884473109));
#3443=CARTESIAN_POINT('Ctrl Pts',(-0.306875813562086,-3.21413052489826,
298.733726884096));
#3444=CARTESIAN_POINT('Ctrl Pts',(-0.110167435728297,-3.22686848774799,
298.747094095232));
#3445=CARTESIAN_POINT('Ctrl Pts',(0.122538922243097,-3.22062147587102,298.762141870928));
#3446=CARTESIAN_POINT('Ctrl Pts',(0.158577091441751,-3.21904831123245,298.764449564213));
#3447=CARTESIAN_POINT('Ctrl Pts',(0.215940807579819,-3.21557847975082,298.768078926574));
#3448=CARTESIAN_POINT('Ctrl Pts',(0.237286024440114,-3.2140738625771,298.769419713178));
#3449=CARTESIAN_POINT('Ctrl Pts',(0.279820894036702,-3.21064953226938,298.772070045707));
#3450=CARTESIAN_POINT('Ctrl Pts',(0.301009642550687,-3.20873236670442,298.773379635183));
#3451=CARTESIAN_POINT('Ctrl Pts',(0.357483491662,-3.20305824830348,298.776845210373));
#3452=CARTESIAN_POINT('Ctrl Pts',(0.392729130563988,-3.19892804677135,298.778982175235));
#3453=CARTESIAN_POINT('Ctrl Pts',(0.472436474736355,-3.18825035829915,298.783770401538));
#3454=CARTESIAN_POINT('Ctrl Pts',(0.516844370135017,-3.18135330070173,298.786406583031));
#3455=CARTESIAN_POINT('Ctrl Pts',(0.666768876743215,-3.15484592176801,298.795242262176));
#3456=CARTESIAN_POINT('Ctrl Pts',(0.771449192611776,-3.13089478736509,298.801304465707));
#3457=CARTESIAN_POINT('Ctrl Pts',(1.09498089377746,-3.03965396986981,298.820202799356));
#3458=CARTESIAN_POINT('Ctrl Pts',(1.30795679462404,-2.95427131424047,298.832931691854));
#3459=CARTESIAN_POINT('Ctrl Pts',(1.5592801309835,-2.82096852048813,298.849686957103));
#3460=CARTESIAN_POINT('Ctrl Pts',(1.60778327113594,-2.79360883740029,298.85300422155));
#3461=CARTESIAN_POINT('Ctrl Pts',(1.68707394293094,-2.74613346000209,298.858582726813));
#3462=CARTESIAN_POINT('Ctrl Pts',(1.71827040180665,-2.72672223128069,298.860818947206));
#3463=CARTESIAN_POINT('Ctrl Pts',(1.77982571474049,-2.68694508810186,298.865318465518));
#3464=CARTESIAN_POINT('Ctrl Pts',(1.81018345625124,-2.66658755053654,298.867581230052));
#3465=CARTESIAN_POINT('Ctrl Pts',(1.88503625403199,-2.61452488125141,298.873273887736));
#3466=CARTESIAN_POINT('Ctrl Pts',(1.92908232715173,-2.58219728921272,298.876726523632));
#3467=CARTESIAN_POINT('Ctrl Pts',(2.11820279416264,-2.43585235974076,298.892017668719));
#3468=CARTESIAN_POINT('Ctrl Pts',(2.25413637994349,-2.31063021183482,298.904275603743));
#3469=CARTESIAN_POINT('Ctrl Pts',(2.5121798699909,-2.02836534794506,298.930021874429));
#3470=CARTESIAN_POINT('Ctrl Pts',(2.63202143352579,-1.87023694225259,298.943479788305));
#3471=CARTESIAN_POINT('Ctrl Pts',(2.75557590075299,-1.67158913535168,298.95859983779));
#3472=CARTESIAN_POINT('Ctrl Pts',(2.77404353435776,-1.64075942629812,298.960898667214));
#3473=CARTESIAN_POINT('Ctrl Pts',(2.80266401943303,-1.59111548070182,298.964517321434));
#3474=CARTESIAN_POINT('Ctrl Pts',(2.81315154979447,-1.57249880639375,298.96585609137));
#3475=CARTESIAN_POINT('Ctrl Pts',(2.83372093834934,-1.53512107991172,298.968505713402));
#3476=CARTESIAN_POINT('Ctrl Pts',(2.84380351986709,-1.51636165969508,298.969816562622));
#3477=CARTESIAN_POINT('Ctrl Pts',(2.87024022903925,-1.46598284603505,298.973290162266));
#3478=CARTESIAN_POINT('Ctrl Pts',(2.88625814159511,-1.43418926538341,298.975433728949));
#3479=CARTESIAN_POINT('Ctrl Pts',(2.96857206817698,-1.26383897929995,298.986696944379));
#3480=CARTESIAN_POINT('Ctrl Pts',(3.02543233258286,-1.12092726726277,298.995380459747));
#3481=CARTESIAN_POINT('Ctrl Pts',(3.13875471800757,-0.7637017781328,299.016446315585));
#3482=CARTESIAN_POINT('Ctrl Pts',(3.18374527431879,-0.546606845896657,299.028754599677));
#3483=CARTESIAN_POINT('Ctrl Pts',(3.21199439995888,-0.269310680461309,299.045128815724));
#3484=CARTESIAN_POINT('Ctrl Pts',(3.21629489894568,-0.211855621199054,299.048552849423));
#3485=CARTESIAN_POINT('Ctrl Pts',(3.22043839029637,-0.125423264005401,299.053766033411));
#3486=CARTESIAN_POINT('Ctrl Pts',(3.22143444773672,-0.0965113372770463,
299.05552024537));
#3487=CARTESIAN_POINT('Ctrl Pts',(3.22251600548125,-0.0449535281750034,
299.058668704482));
#3488=CARTESIAN_POINT('Ctrl Pts',(3.22275229016343,-0.0223126235551124,
299.060058250793));
#3489=CARTESIAN_POINT('Ctrl Pts',(3.22274998327137,0.000328366225831933,
299.061455114234));
#3490=CARTESIAN_POINT('Ctrl Pts',(3.2227499833101,0.000327985858891378,
299.061455090767));
#3491=CARTESIAN_POINT('Ctrl Pts',(3.22274652943001,0.0342654002378796,299.063548900761));
#3492=CARTESIAN_POINT('Ctrl Pts',(3.22220700613506,0.0681998290130912,299.065658974486));
#3493=CARTESIAN_POINT('Ctrl Pts',(3.21947014498759,0.154528700673276,299.071071128188));
#3494=CARTESIAN_POINT('Ctrl Pts',(3.2165298177619,0.206887808251486,299.074395187485));
#3495=CARTESIAN_POINT('Ctrl Pts',(3.19495845765172,0.474277662394748,299.09159017247));
#3496=CARTESIAN_POINT('Ctrl Pts',(3.15603891383566,0.687089508949695,299.10605626149));
#3497=CARTESIAN_POINT('Ctrl Pts',(3.05030848821211,1.05310533397084,299.131749186655));
#3498=CARTESIAN_POINT('Ctrl Pts',(2.99231729381699,1.2080806206243,299.142887430541));
#3499=CARTESIAN_POINT('Ctrl Pts',(2.90851574812353,1.3884472147167,299.155709639974));
#3500=CARTESIAN_POINT('Ctrl Pts',(2.89386167901502,1.41873687176191,299.157857365973));
#3501=CARTESIAN_POINT('Ctrl Pts',(2.86933862323411,1.46746391293589,299.161296922416));
#3502=CARTESIAN_POINT('Ctrl Pts',(2.85976010165921,1.48604398016733,299.162604724947));
#3503=CARTESIAN_POINT('Ctrl Pts',(2.83980893666348,1.52383706194522,299.165255281266));
#3504=CARTESIAN_POINT('Ctrl Pts',(2.82942059866414,1.54304028667318,299.16659707343));
#3505=CARTESIAN_POINT('Ctrl Pts',(2.80032139422189,1.59554907856148,299.170256305141));
#3506=CARTESIAN_POINT('Ctrl Pts',(2.78121172208303,1.62863083914335,299.172550820575));
#3507=CARTESIAN_POINT('Ctrl Pts',(2.69634853721565,1.76969011750964,299.182321221369));
#3508=CARTESIAN_POINT('Ctrl Pts',(2.62485627100743,1.87409545685446,299.189521128991));
#3509=CARTESIAN_POINT('Ctrl Pts',(2.44154800288276,2.11064665212321,299.206395487783));
#3510=CARTESIAN_POINT('Ctrl Pts',(2.32487318237436,2.23851501047242,299.215991761999));
#3511=CARTESIAN_POINT('Ctrl Pts',(2.14650908015825,2.40492706762266,299.229957032947));
#3512=CARTESIAN_POINT('Ctrl Pts',(2.09291929588547,2.45170621938392,299.234072338396));
#3513=CARTESIAN_POINT('Ctrl Pts',(1.99253876365373,2.5336385803422,299.241685753729));
#3514=CARTESIAN_POINT('Ctrl Pts',(1.94625412153623,2.56936362946208,299.245161809221));
#3515=CARTESIAN_POINT('Ctrl Pts',(1.86892391032431,2.62576256718452,299.250931633346));
#3516=CARTESIAN_POINT('Ctrl Pts',(1.83844487782098,2.64719207796599,299.253196496412));
#3517=CARTESIAN_POINT('Ctrl Pts',(1.77803018218675,2.68812241572455,299.257671803833));
#3518=CARTESIAN_POINT('Ctrl Pts',(1.7481281789436,2.70766341351952,299.259880323221));
#3519=CARTESIAN_POINT('Ctrl Pts',(1.67396666145783,2.75438750086574,299.26534497329));
#3520=CARTESIAN_POINT('Ctrl Pts',(1.62936419624911,2.78100462330133,299.268620719597));
#3521=CARTESIAN_POINT('Ctrl Pts',(1.36070805727037,2.93264695287077,299.288299071401));
#3522=CARTESIAN_POINT('Ctrl Pts',(1.12304640696586,3.03161158339221,299.305600120804));
#3523=CARTESIAN_POINT('Ctrl Pts',(0.785279453879957,3.12704089828685,299.329239937053));
#3524=CARTESIAN_POINT('Ctrl Pts',(0.693244638444545,3.14872389556241,299.335577660602));
#3525=CARTESIAN_POINT('Ctrl Pts',(0.559341962365844,3.17411394233356,299.344548507362));
#3526=CARTESIAN_POINT('Ctrl Pts',(0.518148570284986,3.18109809877438,299.347274453156));
#3527=CARTESIAN_POINT('Ctrl Pts',(0.44358771873394,3.19225268942585,299.352134743905));
#3528=CARTESIAN_POINT('Ctrl Pts',(0.410268840565864,3.19670564467387,299.354280277517));
#3529=CARTESIAN_POINT('Ctrl Pts',(0.35613154876545,3.20308047946914,299.357717304906));
#3530=CARTESIAN_POINT('Ctrl Pts',(0.335353965326037,3.20532245422802,299.359024726494));
#3531=CARTESIAN_POINT('Ctrl Pts',(0.292817714721626,3.20949410429793,299.361675489255));
#3532=CARTESIAN_POINT('Ctrl Pts',(0.271058544082364,3.21140498032574,299.363017853156));
#3533=CARTESIAN_POINT('Ctrl Pts',(0.21114739735927,3.2160530557697,299.366680538027));
#3534=CARTESIAN_POINT('Ctrl Pts',(0.172962378619341,3.21833260831637,299.368977862752));
#3535=CARTESIAN_POINT('Ctrl Pts',(-0.0367391129070247,3.22710795688053,
299.381434179051));
#3536=CARTESIAN_POINT('Ctrl Pts',(-0.208539857577076,3.22057428817795,299.3910627984));
#3537=CARTESIAN_POINT('Ctrl Pts',(-0.520108818447957,3.18367562584064,299.408673204732));
#3538=CARTESIAN_POINT('Ctrl Pts',(-0.659937138630424,3.15765484489247,299.416632983012));
#3539=CARTESIAN_POINT('Ctrl Pts',(-0.860212983691056,3.10649789293809,299.428522095241));
#3540=CARTESIAN_POINT('Ctrl Pts',(-0.922341162682467,3.08862131492622,299.432279418562));
#3541=CARTESIAN_POINT('Ctrl Pts',(-1.03581087776999,3.05224287121845,299.439304573561));
#3542=CARTESIAN_POINT('Ctrl Pts',(-1.08730109076792,3.03428188383167,299.442555827765));
#3543=CARTESIAN_POINT('Ctrl Pts',(-1.17248507537425,3.00212105285813,299.448055174808));
#3544=CARTESIAN_POINT('Ctrl Pts',(-1.20643833823916,2.98863822465511,299.450279805762));
#3545=CARTESIAN_POINT('Ctrl Pts',(-1.27408318216367,2.96043592938583,299.454781494208));
#3546=CARTESIAN_POINT('Ctrl Pts',(-1.30776664591104,2.94571130162186,299.457058456034));
#3547=CARTESIAN_POINT('Ctrl Pts',(-1.39191632125742,2.90719773986043,299.462839738995));
#3548=CARTESIAN_POINT('Ctrl Pts',(-1.44202878292749,2.8826692714849,299.46636835399));
#3549=CARTESIAN_POINT('Ctrl Pts',(-1.69354036726437,2.75136266606126,299.484529315101));
#3550=CARTESIAN_POINT('Ctrl Pts',(-1.88381382441009,2.62474594363358,299.499834162193));
#3551=CARTESIAN_POINT('Ctrl Pts',(-2.14202141941021,2.41028582596662,299.522467306961));
#3552=CARTESIAN_POINT('Ctrl Pts',(-2.22142777066103,2.33730489266956,299.529722523681));
#3553=CARTESIAN_POINT('Ctrl Pts',(-2.32862346381739,2.22837588240021,299.53981012481));
#3554=CARTESIAN_POINT('Ctrl Pts',(-2.35954122060311,2.19561196591743,299.542757171771));
#3555=CARTESIAN_POINT('Ctrl Pts',(-2.41361158563693,2.13585115751491,299.547963874209));
#3556=CARTESIAN_POINT('Ctrl Pts',(-2.43702329695914,2.10909903505091,299.550237075028));
#3557=CARTESIAN_POINT('Ctrl Pts',(-2.47373989080687,2.06571576246227,299.553825279728));
#3558=CARTESIAN_POINT('Ctrl Pts',(-2.48733028638676,2.04933129748226,299.555158715314));
#3559=CARTESIAN_POINT('Ctrl Pts',(-2.51424196133368,2.01622466805292,299.557807836605));
#3560=CARTESIAN_POINT('Ctrl Pts',(-2.52756117562432,1.99950221672883,299.559123370618));
#3561=CARTESIAN_POINT('Ctrl Pts',(-2.5628531317649,1.95427646307167,299.562624899302));
#3562=CARTESIAN_POINT('Ctrl Pts',(-2.58451708114854,1.92553482567744,299.564791164076));
#3563=CARTESIAN_POINT('Ctrl Pts',(-2.72188392441937,1.73679319741942,299.578681682843));
#3564=CARTESIAN_POINT('Ctrl Pts',(-2.82316845962759,1.56679295450636,299.589675973107));
#3565=CARTESIAN_POINT('Ctrl Pts',(-2.96356564030094,1.27274189386293,299.607969050815));
#3566=CARTESIAN_POINT('Ctrl Pts',(-3.01189893099362,1.15371381949891,299.615193673971));
#3567=CARTESIAN_POINT('Ctrl Pts',(-3.07262239223831,0.974095302863697,299.626128825142));
#3568=CARTESIAN_POINT('Ctrl Pts',(-3.09058142087567,0.915519471101641,299.629698847361));
#3569=CARTESIAN_POINT('Ctrl Pts',(-3.12079038022706,0.805935910786828,299.636413511808));
#3570=CARTESIAN_POINT('Ctrl Pts',(-3.13348544947862,0.755072031760421,299.639544146113));
#3571=CARTESIAN_POINT('Ctrl Pts',(-3.15283208023271,0.668636640488964,299.644899835209));
#3572=CARTESIAN_POINT('Ctrl Pts',(-3.16013549121602,0.633220813553157,299.64710420046));
#3573=CARTESIAN_POINT('Ctrl Pts',(-3.17292822332172,0.565439008533792,299.651345267361));
#3574=CARTESIAN_POINT('Ctrl Pts',(-3.17852198387097,0.533097229954114,299.653378409875));
#3575=CARTESIAN_POINT('Ctrl Pts',(-3.19202971807472,0.447206447929462,299.658805451542));
#3576=CARTESIAN_POINT('Ctrl Pts',(-3.19908993931695,0.39353568476881,299.662225051569));
#3577=CARTESIAN_POINT('Ctrl Pts',(-3.23021349317849,0.0999230793525244,
299.681096782862));
#3578=CARTESIAN_POINT('Ctrl Pts',(-3.22863505367647,-0.141930876552373,
299.697320409317));
#3579=CARTESIAN_POINT('Ctrl Pts',(-3.18812008460518,-0.481958291917196,
299.720401367959));
#3580=CARTESIAN_POINT('Ctrl Pts',(-3.17138333488818,-0.581999202259457,
299.72721350014));
#3581=CARTESIAN_POINT('Ctrl Pts',(-3.14076408719736,-0.723609758698783,
299.736764485859));
#3582=CARTESIAN_POINT('Ctrl Pts',(-3.13070964948847,-0.765942270748718,
299.739607364256));
#3583=CARTESIAN_POINT('Ctrl Pts',(-3.11111494654605,-0.841594533335596,
299.74465130694));
#3584=CARTESIAN_POINT('Ctrl Pts',(-3.10188863376593,-0.874988395979888,
299.746864783742));
#3585=CARTESIAN_POINT('Ctrl Pts',(-3.08617850944212,-0.928474576100684,
299.750382134578));
#3586=CARTESIAN_POINT('Ctrl Pts',(-3.08003282585468,-0.948662581466748,
299.751703260386));
#3587=CARTESIAN_POINT('Ctrl Pts',(-3.06720178168864,-0.989371772621045,
299.754352162033));
#3588=CARTESIAN_POINT('Ctrl Pts',(-3.06050773848367,-1.009888962818,299.755679415671));
#3589=CARTESIAN_POINT('Ctrl Pts',(-3.04178754238398,-1.06536991872102,299.759251187829));
#3590=CARTESIAN_POINT('Ctrl Pts',(-3.02936467036833,-1.10019746737571,299.761474577198));
#3591=CARTESIAN_POINT('Ctrl Pts',(-2.95130406516198,-1.30768480066771,299.774650452702));
#3592=CARTESIAN_POINT('Ctrl Pts',(-2.87151386680793,-1.47467219581102,299.784974557556));
#3593=CARTESIAN_POINT('Ctrl Pts',(-2.67594058513953,-1.80716927650832,299.806624503734));
#3594=CARTESIAN_POINT('Ctrl Pts',(-2.55806070616615,-1.97049076739934,299.817925501167));
#3595=CARTESIAN_POINT('Ctrl Pts',(-2.391343347136,-2.16109344518877,299.832886243998));
#3596=CARTESIAN_POINT('Ctrl Pts',(-2.35599196947165,-2.19957933981397,299.836007359242));
#3597=CARTESIAN_POINT('Ctrl Pts',(-2.29464016256247,-2.26319454798497,299.841351784131));
#3598=CARTESIAN_POINT('Ctrl Pts',(-2.26912351267697,-2.28877726322254,299.843554619228));
#3599=CARTESIAN_POINT('Ctrl Pts',(-2.21959650962692,-2.33679011411177,299.847796089334));
#3600=CARTESIAN_POINT('Ctrl Pts',(-2.19566259756052,-2.35929276184724,299.849831221558));
#3601=CARTESIAN_POINT('Ctrl Pts',(-2.13125957688887,-2.41801560520044,299.855271832299));
#3602=CARTESIAN_POINT('Ctrl Pts',(-2.09021316436199,-2.45358415793376,299.858703254716));
#3603=CARTESIAN_POINT('Ctrl Pts',(-1.87125441526666,-2.63383874863234,299.876833425788));
#3604=CARTESIAN_POINT('Ctrl Pts',(-1.67921620378575,-2.7602309503553,299.892218230902));
#3605=CARTESIAN_POINT('Ctrl Pts',(-1.47546400147781,-2.86515680946839,299.907672586636));
#3606=CARTESIAN_POINT('Origin',(0.,0.,294.689226550727));
#3607=CARTESIAN_POINT('',(-1.47546400249216,-2.86515680894603,301.40644069294));
#3608=CARTESIAN_POINT('',(-1.47546399521001,-2.86515681269611,301.158594111703));
#3609=CARTESIAN_POINT('',(-1.47546400239267,-2.86515680899727,294.689226550727));
#3610=CARTESIAN_POINT('',(3.22274884483193,-0.00272866899239652,300.5603484081));
#3611=CARTESIAN_POINT('Ctrl Pts',(-1.47546400249216,-2.86515680894603,301.40644069294));
#3612=CARTESIAN_POINT('Ctrl Pts',(-1.48048779144244,-2.86256971851904,301.406095014753));
#3613=CARTESIAN_POINT('Ctrl Pts',(-1.48550478569221,-2.85996941000239,301.405748883669));
#3614=CARTESIAN_POINT('Ctrl Pts',(-1.52255103390791,-2.84064455585854,301.403186139525));
#3615=CARTESIAN_POINT('Ctrl Pts',(-1.55430275391081,-2.82339616904349,301.400951628733));
#3616=CARTESIAN_POINT('Ctrl Pts',(-1.63139331994373,-2.77982399220617,301.395429324958));
#3617=CARTESIAN_POINT('Ctrl Pts',(-1.67639146020706,-2.75292149557001,301.39212163822));
#3618=CARTESIAN_POINT('Ctrl Pts',(-1.7725252509366,-2.69221599731516,301.384865802181));
#3619=CARTESIAN_POINT('Ctrl Pts',(-1.82339246276776,-2.65802782598722,301.380905315219));
#3620=CARTESIAN_POINT('Ctrl Pts',(-1.97781921567345,-2.54771709546525,301.368503391277));
#3621=CARTESIAN_POINT('Ctrl Pts',(-2.07781750929126,-2.46684027798489,301.359919053805));
#3622=CARTESIAN_POINT('Ctrl Pts',(-2.31836096538013,-2.24726693192574,301.337992074979));
#3623=CARTESIAN_POINT('Ctrl Pts',(-2.45150570599166,-2.1012223433221,301.324589002491));
#3624=CARTESIAN_POINT('Ctrl Pts',(-2.59218619337671,-1.91519830870355,301.309513481265));
#3625=CARTESIAN_POINT('Ctrl Pts',(-2.6134213391613,-1.88611849344987,301.307210001328));
#3626=CARTESIAN_POINT('Ctrl Pts',(-2.64647562913427,-1.83922289510277,301.303586672688));
#3627=CARTESIAN_POINT('Ctrl Pts',(-2.6586120071956,-1.82163562989948,301.302247773877));
#3628=CARTESIAN_POINT('Ctrl Pts',(-2.68246785346804,-1.78631894103634,301.299600772632));
#3629=CARTESIAN_POINT('Ctrl Pts',(-2.6941886474835,-1.76859173644498,301.298292630756));
#3630=CARTESIAN_POINT('Ctrl Pts',(-2.72498550734598,-1.72099606118296,301.294831142034));
#3631=CARTESIAN_POINT('Ctrl Pts',(-2.74374623397127,-1.69092586774839,301.292696769458));
#3632=CARTESIAN_POINT('Ctrl Pts',(-2.78512765680131,-1.62209581055673,301.287914749298));
#3633=CARTESIAN_POINT('Ctrl Pts',(-2.80744275713907,-1.58316025860629,301.285282137501));
#3634=CARTESIAN_POINT('Ctrl Pts',(-2.88023795856153,-1.4497639774965,301.276462399039));
#3635=CARTESIAN_POINT('Ctrl Pts',(-2.92682278557449,-1.35325428603195,301.270412113192));
#3636=CARTESIAN_POINT('Ctrl Pts',(-3.05778951249449,-1.04337290603943,301.251498066971));
#3637=CARTESIAN_POINT('Ctrl Pts',(-3.12425490059124,-0.823240909377905,
301.238743451911));
#3638=CARTESIAN_POINT('Ctrl Pts',(-3.17711292787648,-0.543288723888024,
301.221963093766));
#3639=CARTESIAN_POINT('Ctrl Pts',(-3.18601280926782,-0.488396394497893,
301.218650368036));
#3640=CARTESIAN_POINT('Ctrl Pts',(-3.19842228888966,-0.396937366890892,
301.213078985377));
#3641=CARTESIAN_POINT('Ctrl Pts',(-3.20273487571026,-0.360490719708634,
301.210845269089));
#3642=CARTESIAN_POINT('Ctrl Pts',(-3.21009463848992,-0.287651167234611,
301.206350558358));
#3643=CARTESIAN_POINT('Ctrl Pts',(-3.213147498771,-0.25126432768427,301.204090091128));
#3644=CARTESIAN_POINT('Ctrl Pts',(-3.2192196670176,-0.160377892211314,301.198403072046));
#3645=CARTESIAN_POINT('Ctrl Pts',(-3.22147382249619,-0.105840337517778,
301.19495381777));
#3646=CARTESIAN_POINT('Ctrl Pts',(-3.22337208614907,0.013456305133541,301.187324709849));
#3647=CARTESIAN_POINT('Ctrl Pts',(-3.22245133808547,0.0781996587369309,
301.183130064313));
#3648=CARTESIAN_POINT('Ctrl Pts',(-3.2132609586872,0.285307921366612,301.169544638267));
#3649=CARTESIAN_POINT('Ctrl Pts',(-3.19749502732674,0.427160833119939,301.159977973014));
#3650=CARTESIAN_POINT('Ctrl Pts',(-3.14226428957243,0.735911014105936,301.138830886301));
#3651=CARTESIAN_POINT('Ctrl Pts',(-3.09877102466537,0.901674028955715,301.127260008606));
#3652=CARTESIAN_POINT('Ctrl Pts',(-3.02973848380263,1.0992071805318,301.113705382374));
#3653=CARTESIAN_POINT('Ctrl Pts',(-3.01651948328793,1.13498114460499,301.111261102602));
#3654=CARTESIAN_POINT('Ctrl Pts',(-2.99474853941737,1.19082920009342,301.107470861951));
#3655=CARTESIAN_POINT('Ctrl Pts',(-2.98662284026428,1.21106443712615,301.106102926268));
#3656=CARTESIAN_POINT('Ctrl Pts',(-2.97031378161113,1.25051578372242,301.103448672512));
#3657=CARTESIAN_POINT('Ctrl Pts',(-2.96214790108208,1.26973758360641,301.102161573342));
#3658=CARTESIAN_POINT('Ctrl Pts',(-2.94035171587583,1.31968911012023,301.098829552937));
#3659=CARTESIAN_POINT('Ctrl Pts',(-2.92642601848393,1.35028830888471,301.096801114455));
#3660=CARTESIAN_POINT('Ctrl Pts',(-2.84072075294001,1.5310531480985,301.084862002645));
#3661=CARTESIAN_POINT('Ctrl Pts',(-2.75786696914208,1.67570882832922,301.075481696633));
#3662=CARTESIAN_POINT('Ctrl Pts',(-2.54295500602276,1.99146429361558,301.054028608583));
#3663=CARTESIAN_POINT('Ctrl Pts',(-2.4041623443193,2.15697574230061,301.042003189011));
#3664=CARTESIAN_POINT('Ctrl Pts',(-2.2090906640932,2.34718653378429,301.025974837117));
#3665=CARTESIAN_POINT('Ctrl Pts',(-2.1672362262738,2.38588615679911,301.022582423097));
#3666=CARTESIAN_POINT('Ctrl Pts',(-2.09658858650008,2.44781528355479,301.016915174149));
#3667=CARTESIAN_POINT('Ctrl Pts',(-2.06838166952625,2.4716958674441,301.014667202694));
#3668=CARTESIAN_POINT('Ctrl Pts',(-2.0116750446927,2.51805441690071,301.01017292876));
#3669=CARTESIAN_POINT('Ctrl Pts',(-1.9831938859128,2.5405464717554,301.007927654445));
#3670=CARTESIAN_POINT('Ctrl Pts',(-1.91193839791788,2.59488973420661,301.002336430517));
#3671=CARTESIAN_POINT('Ctrl Pts',(-1.86874296911706,2.62616837924515,300.998969422062));
#3672=CARTESIAN_POINT('Ctrl Pts',(-1.65413860550772,2.7735914227825,300.982339853672));
#3673=CARTESIAN_POINT('Ctrl Pts',(-1.47260812854855,2.87408866741503,300.968527613011));
#3674=CARTESIAN_POINT('Ctrl Pts',(-1.12317577973019,3.02569687979525,300.942849370896));
#3675=CARTESIAN_POINT('Ctrl Pts',(-0.958274226056778,3.08189617965034,300.93107942795));
#3676=CARTESIAN_POINT('Ctrl Pts',(-0.752520091850376,3.13389477707587,300.917330126871));
#3677=CARTESIAN_POINT('Ctrl Pts',(-0.715240363419869,3.14261268272783,300.914876100239));
#3678=CARTESIAN_POINT('Ctrl Pts',(-0.656466246644875,3.15525694291316,300.91107433019));
#3679=CARTESIAN_POINT('Ctrl Pts',(-0.635073282425498,3.15963230419091,300.909704403945));
#3680=CARTESIAN_POINT('Ctrl Pts',(-0.593156579751613,3.16776231006098,300.907049445366));
#3681=CARTESIAN_POINT('Ctrl Pts',(-0.57263793945248,3.17153568526683,300.905763583054));
#3682=CARTESIAN_POINT('Ctrl Pts',(-0.519074425484693,3.1808492353663,300.902439396346));
#3683=CARTESIAN_POINT('Ctrl Pts',(-0.485976205180451,3.18607398562912,300.900417406232));
#3684=CARTESIAN_POINT('Ctrl Pts',(-0.411605773256444,3.1966278295378,300.895933891364));
#3685=CARTESIAN_POINT('Ctrl Pts',(-0.370299313783368,3.20167573405516,300.893484717169));
#3686=CARTESIAN_POINT('Ctrl Pts',(-0.235498359699913,3.21550535907748,300.885592504093));
#3687=CARTESIAN_POINT('Ctrl Pts',(-0.141712217226645,3.221001982046,300.88025759648));
#3688=CARTESIAN_POINT('Ctrl Pts',(0.210172167162838,3.22622340342791,300.860415233727));
#3689=CARTESIAN_POINT('Ctrl Pts',(0.467663024958985,3.19905803019254,300.846160749087));
#3690=CARTESIAN_POINT('Ctrl Pts',(0.769549770924178,3.12994940917951,300.827854387569));
#3691=CARTESIAN_POINT('Ctrl Pts',(0.819656191181735,3.11720282385432,300.824765123725));
#3692=CARTESIAN_POINT('Ctrl Pts',(0.903762576384387,3.09363893144115,300.819481683605));
#3693=CARTESIAN_POINT('Ctrl Pts',(0.937929671882019,3.08345202787499,300.817307646901));
#3694=CARTESIAN_POINT('Ctrl Pts',(1.00744792827213,3.06146284911055,300.812823945922));
#3695=CARTESIAN_POINT('Ctrl Pts',(1.04277732018905,3.0496100379103,300.810512938629));
#3696=CARTESIAN_POINT('Ctrl Pts',(1.13315022490661,3.01753644349174,300.804514294769));
#3697=CARTESIAN_POINT('Ctrl Pts',(1.18785977209493,2.99642187992722,300.800798388116));
#3698=CARTESIAN_POINT('Ctrl Pts',(1.3078750771396,2.9462998645552,300.792453432364));
#3699=CARTESIAN_POINT('Ctrl Pts',(1.37285243119301,2.91658964956414,300.787804277415));
#3700=CARTESIAN_POINT('Ctrl Pts',(1.59306701486275,2.80690891557254,300.771603948267));
#3701=CARTESIAN_POINT('Ctrl Pts',(1.74275568726422,2.71650413598036,300.75979036805));
#3702=CARTESIAN_POINT('Ctrl Pts',(1.9939557294236,2.53544955282293,300.738942127581));
#3703=CARTESIAN_POINT('Ctrl Pts',(2.09847356513752,2.449648755529,300.729909877036));
#3704=CARTESIAN_POINT('Ctrl Pts',(2.22094805248526,2.3354982089623,300.719132689149));
#3705=CARTESIAN_POINT('Ctrl Pts',(2.24425918410452,2.31310679234612,300.717072293906));
#3706=CARTESIAN_POINT('Ctrl Pts',(2.28045044231943,2.27728113395602,300.713864425716));
#3707=CARTESIAN_POINT('Ctrl Pts',(2.29355727659156,2.26408008880387,300.712700756559));
#3708=CARTESIAN_POINT('Ctrl Pts',(2.32154037620654,2.23540344763261,300.710213618923));
#3709=CARTESIAN_POINT('Ctrl Pts',(2.33637787553941,2.21989116272948,300.708893124301));
#3710=CARTESIAN_POINT('Ctrl Pts',(2.37600815126554,2.17762103131011,300.705357596258));
#3711=CARTESIAN_POINT('Ctrl Pts',(2.4005041380894,2.1505878780608,300.703162994628));
#3712=CARTESIAN_POINT('Ctrl Pts',(2.45527387975482,2.08804322715453,300.698218993814));
#3713=CARTESIAN_POINT('Ctrl Pts',(2.48524634108066,2.05227809008357,300.695486201604));
#3714=CARTESIAN_POINT('Ctrl Pts',(2.58629395556978,1.9262396823475,300.686127443769));
#3715=CARTESIAN_POINT('Ctrl Pts',(2.65331476419022,1.83282277765959,300.679656324057));
#3716=CARTESIAN_POINT('Ctrl Pts',(2.83180430068046,1.55365811498024,300.661046339581));
#3717=CARTESIAN_POINT('Ctrl Pts',(2.92972362144358,1.36002908993869,300.648964795727));
#3718=CARTESIAN_POINT('Ctrl Pts',(3.02770628031384,1.10556583450756,300.632913304538));
#3719=CARTESIAN_POINT('Ctrl Pts',(3.04653891883523,1.05255935604962,300.629563810806));
#3720=CARTESIAN_POINT('Ctrl Pts',(3.0753880828721,0.964085702392131,300.623948239376));
#3721=CARTESIAN_POINT('Ctrl Pts',(3.08620092283184,0.928890088242497,300.621707983677));
#3722=CARTESIAN_POINT('Ctrl Pts',(3.10650185738157,0.858538985392412,300.6172137711));
#3723=CARTESIAN_POINT('Ctrl Pts',(3.11600183482399,0.823392601023137,300.614960576127));
#3724=CARTESIAN_POINT('Ctrl Pts',(3.13810474941508,0.735751411190933,300.60931922431));
#3725=CARTESIAN_POINT('Ctrl Pts',(3.14998755182577,0.683088158279952,300.605909152221));
#3726=CARTESIAN_POINT('Ctrl Pts',(3.20209880960479,0.421723666838208,300.588876913646));
#3727=CARTESIAN_POINT('Ctrl Pts',(3.22292873155932,0.209730132176812,300.574674566188));
#3728=CARTESIAN_POINT('Ctrl Pts',(3.22274884483193,-0.00272866899239652,
300.5603484081));
#3729=CARTESIAN_POINT('Ctrl Pts',(3.22274884385928,-0.00272981751187232,
300.560348330655));
#3730=CARTESIAN_POINT('Ctrl Pts',(3.22263402356394,-0.138283557810964,300.551207902855));
#3731=CARTESIAN_POINT('Ctrl Pts',(3.21396693228134,-0.273703941416887,300.54205285242));
#3732=CARTESIAN_POINT('Ctrl Pts',(3.19035975633614,-0.458589497413305,300.529792771035));
#3733=CARTESIAN_POINT('Ctrl Pts',(3.18273208395242,-0.508838635045151,300.526486096843));
#3734=CARTESIAN_POINT('Ctrl Pts',(3.17007469760743,-0.580719665148035,300.521811256994));
#3735=CARTESIAN_POINT('Ctrl Pts',(3.16600533064313,-0.602510766804593,300.520401429198));
#3736=CARTESIAN_POINT('Ctrl Pts',(3.15763570940016,-0.644900760220875,300.517675528554));
#3737=CARTESIAN_POINT('Ctrl Pts',(3.15335787500929,-0.665503154493343,300.51635838811));
#3738=CARTESIAN_POINT('Ctrl Pts',(3.14427972183635,-0.707169880936442,300.513712214637));
#3739=CARTESIAN_POINT('Ctrl Pts',(3.13946880615948,-0.728230654001299,300.512383782968));
#3740=CARTESIAN_POINT('Ctrl Pts',(3.12581084655722,-0.785368579262997,300.508800632964));
#3741=CARTESIAN_POINT('Ctrl Pts',(3.11655103135972,-0.82134474032904,300.50656730374));
#3742=CARTESIAN_POINT('Ctrl Pts',(3.05664870658941,-1.03845475247073,300.493184028216));
#3743=CARTESIAN_POINT('Ctrl Pts',(2.99084633230843,-1.2150486230341,300.482684704198));
#3744=CARTESIAN_POINT('Ctrl Pts',(2.82517085049119,-1.56317040140482,300.461045708711));
#3745=CARTESIAN_POINT('Ctrl Pts',(2.72414303459175,-1.73324163970284,300.449933952863));
#3746=CARTESIAN_POINT('Ctrl Pts',(2.5775446613667,-1.93522719381413,300.435188088566));
#3747=CARTESIAN_POINT('Ctrl Pts',(2.54587245025847,-1.97670781637585,300.432070924453));
#3748=CARTESIAN_POINT('Ctrl Pts',(2.49061515624663,-2.0455454899615,300.42673287346));
#3749=CARTESIAN_POINT('Ctrl Pts',(2.46755143369191,-2.07330894209824,300.424532399853));
#3750=CARTESIAN_POINT('Ctrl Pts',(2.42263563218952,-2.12556607624192,300.420295341215));
#3751=CARTESIAN_POINT('Ctrl Pts',(2.40086601484393,-2.15012483484957,300.418262248426));
#3752=CARTESIAN_POINT('Ctrl Pts',(2.34212085698658,-2.21439179561324,300.412827036108));
#3753=CARTESIAN_POINT('Ctrl Pts',(2.30451240997127,-2.25350463246978,300.409399021457));
#3754=CARTESIAN_POINT('Ctrl Pts',(2.09525675002074,-2.46041252029592,300.390587583881));
#3755=CARTESIAN_POINT('Ctrl Pts',(1.90628076146895,-2.60955735949895,300.374441273762));
#3756=CARTESIAN_POINT('Ctrl Pts',(1.6160190181811,-2.79015857136675,300.351397885107));
#3757=CARTESIAN_POINT('Ctrl Pts',(1.52698572853849,-2.83986245727343,300.344548760881));
#3758=CARTESIAN_POINT('Ctrl Pts',(1.39668735227513,-2.9047005154241,300.33495352086));
#3759=CARTESIAN_POINT('Ctrl Pts',(1.35723895516576,-2.92334113684662,300.332102468478));
#3760=CARTESIAN_POINT('Ctrl Pts',(1.28574892773296,-2.9553632193987,300.327046142321));
#3761=CARTESIAN_POINT('Ctrl Pts',(1.25384669183796,-2.96903869264591,300.324828360815));
#3762=CARTESIAN_POINT('Ctrl Pts',(1.20220267910952,-2.99019589975931,300.321306764935));
#3763=CARTESIAN_POINT('Ctrl Pts',(1.18259816006196,-2.99800341266394,300.319985603349));
#3764=CARTESIAN_POINT('Ctrl Pts',(1.14283730650054,-3.01338746836862,300.317339642542));
#3765=CARTESIAN_POINT('Ctrl Pts',(1.12267900572573,-3.02095565241521,300.316015318002));
#3766=CARTESIAN_POINT('Ctrl Pts',(1.06786733268022,-3.04090957565896,300.312456821993));
#3767=CARTESIAN_POINT('Ctrl Pts',(1.03307424835159,-3.05290509813842,300.310243541878));
#3768=CARTESIAN_POINT('Ctrl Pts',(0.818982685910732,-3.12263740205925,300.296858473464));
#3769=CARTESIAN_POINT('Ctrl Pts',(0.635093942554579,-3.16516479363169,300.286342352417));
#3770=CARTESIAN_POINT('Ctrl Pts',(0.255463558805834,-3.21851914376431,300.264825495707));
#3771=CARTESIAN_POINT('Ctrl Pts',(0.0603560283042357,-3.22807598171627,
300.253854329408));
#3772=CARTESIAN_POINT('Ctrl Pts',(-0.187820234823062,-3.21771638988053,
300.239195990994));
#3773=CARTESIAN_POINT('Ctrl Pts',(-0.241164486279621,-3.21415843061964,
300.236005987414));
#3774=CARTESIAN_POINT('Ctrl Pts',(-0.330554862086876,-3.20595846777733,
300.230581421172));
#3775=CARTESIAN_POINT('Ctrl Pts',(-0.366656446533083,-3.2020304653081,300.228368927455));
#3776=CARTESIAN_POINT('Ctrl Pts',(-0.439321513808164,-3.19287924149815,
300.223868241477));
#3777=CARTESIAN_POINT('Ctrl Pts',(-0.475876891971064,-3.18763584025664,
300.221579742092));
#3778=CARTESIAN_POINT('Ctrl Pts',(-0.568452387376828,-3.17272918695839,
300.215718983643));
#3779=CARTESIAN_POINT('Ctrl Pts',(-0.624319929774472,-3.16221008112863,
300.212120962107));
#3780=CARTESIAN_POINT('Ctrl Pts',(-0.892317525167407,-3.10437109075683,
300.194555764433));
#3781=CARTESIAN_POINT('Ctrl Pts',(-1.0995463289475,-3.03715696783775,300.179989180362));
#3782=CARTESIAN_POINT('Ctrl Pts',(-1.35828667077545,-2.92326112942877,300.160924389405));
#3783=CARTESIAN_POINT('Ctrl Pts',(-1.41733349196844,-2.8950921639252,300.156514620214));
#3784=CARTESIAN_POINT('Ctrl Pts',(-1.47546414420613,-2.86515673596787,300.152134095017));
#3785=CARTESIAN_POINT('Ctrl Pts',(-1.47546400147781,-2.86515680946839,299.907672586636));
#3786=CARTESIAN_POINT('Ctrl Pts',(-1.46614549632343,-2.86995554120183,299.908379383872));
#3787=CARTESIAN_POINT('Ctrl Pts',(-1.45680248144607,-2.87470937826137,299.909086182415));
#3788=CARTESIAN_POINT('Ctrl Pts',(-1.35630692718034,-2.92522681046287,299.916667929943));
#3789=CARTESIAN_POINT('Ctrl Pts',(-1.2630510708519,-2.96668573293135,299.923523196095));
#3790=CARTESIAN_POINT('Ctrl Pts',(-1.12729366034639,-3.01947552888274,299.933126642353));
#3791=CARTESIAN_POINT('Ctrl Pts',(-1.0862858066101,-3.03446979761809,299.935979874891));
#3792=CARTESIAN_POINT('Ctrl Pts',(-1.01212912733449,-3.05988863794045,299.941040034042));
#3793=CARTESIAN_POINT('Ctrl Pts',(-0.979092601259422,-3.07061911459943,
299.943259483826));
#3794=CARTESIAN_POINT('Ctrl Pts',(-0.92569797176187,-3.08701261292958,299.946783918306));
#3795=CARTESIAN_POINT('Ctrl Pts',(-0.905447115323019,-3.09301296457067,
299.948106271847));
#3796=CARTESIAN_POINT('Ctrl Pts',(-0.864407938164433,-3.10473529840201,
299.950755134605));
#3797=CARTESIAN_POINT('Ctrl Pts',(-0.84361837254559,-3.11044859442196,299.952081159809));
#3798=CARTESIAN_POINT('Ctrl Pts',(-0.787125172449847,-3.1253657141003,299.955645560967));
#3799=CARTESIAN_POINT('Ctrl Pts',(-0.751317393496701,-3.13416644625843,
299.957862956354));
#3800=CARTESIAN_POINT('Ctrl Pts',(-0.532671359600873,-3.18394181369133,
299.971192280551));
#3801=CARTESIAN_POINT('Ctrl Pts',(-0.346678237634265,-3.20952546969058,
299.98165617031));
#3802=CARTESIAN_POINT('Ctrl Pts',(0.0372148264363069,-3.22854829431113,
300.003228977299));
#3803=CARTESIAN_POINT('Ctrl Pts',(0.234388536033836,-3.22024239596763,300.014310004518));
#3804=CARTESIAN_POINT('Ctrl Pts',(0.482051794969479,-3.18693405805876,300.029063880486));
#3805=CARTESIAN_POINT('Ctrl Pts',(0.534357668223951,-3.178582079839,300.03222565744));
#3806=CARTESIAN_POINT('Ctrl Pts',(0.622080479900717,-3.16234845936203,300.037618309369));
#3807=CARTESIAN_POINT('Ctrl Pts',(0.657614014048308,-3.15515063787719,300.039827788519));
#3808=CARTESIAN_POINT('Ctrl Pts',(0.729240404471182,-3.13937919173193,300.044335982624));
#3809=CARTESIAN_POINT('Ctrl Pts',(0.765321674172179,-3.13077879013615,300.046635236049));
#3810=CARTESIAN_POINT('Ctrl Pts',(0.857011999069836,-3.10724360394996,300.052553853443));
#3811=CARTESIAN_POINT('Ctrl Pts',(0.912382047605976,-3.09143829261983,300.056199967282));
#3812=CARTESIAN_POINT('Ctrl Pts',(1.12495959550549,-3.02454992160777,300.070486066516));
#3813=CARTESIAN_POINT('Ctrl Pts',(1.27855345736226,-2.96289134481449,300.081443362004));
#3814=CARTESIAN_POINT('Ctrl Pts',(1.56088046982927,-2.82350041126875,300.10260935198));
#3815=CARTESIAN_POINT('Ctrl Pts',(1.69026189260278,-2.74800263035757,300.112761577617));
#3816=CARTESIAN_POINT('Ctrl Pts',(1.85816883150405,-2.63366485023254,300.126251269833));
#3817=CARTESIAN_POINT('Ctrl Pts',(1.90165112551842,-2.60244221840407,300.129774428926));
#3818=CARTESIAN_POINT('Ctrl Pts',(1.97650701846783,-2.54581317211189,300.135867306005));
#3819=CARTESIAN_POINT('Ctrl Pts',(2.00821843609142,-2.52087360788797,300.138457536914));
#3820=CARTESIAN_POINT('Ctrl Pts',(2.0566934255627,-2.48125480178025,300.142420890205));
#3821=CARTESIAN_POINT('Ctrl Pts',(2.07378616993264,-2.46698687183886,300.143819166602));
#3822=CARTESIAN_POINT('Ctrl Pts',(2.10624022151505,-2.43932061628085,300.146473293157));
#3823=CARTESIAN_POINT('Ctrl Pts',(2.12162452493683,-2.42595184109241,300.147730879588));
#3824=CARTESIAN_POINT('Ctrl Pts',(2.16080206350537,-2.39124928900228,300.150934838974));
#3825=CARTESIAN_POINT('Ctrl Pts',(2.18440742048186,-2.36970528001336,300.152866728992));
#3826=CARTESIAN_POINT('Ctrl Pts',(2.2953856884683,-2.26535047645006,300.161978356271));
#3827=CARTESIAN_POINT('Ctrl Pts',(2.3784016363506,-2.17803109228465,300.168883675901));
#3828=CARTESIAN_POINT('Ctrl Pts',(2.57658716420537,-1.94468965340345,300.186211081492));
#3829=CARTESIAN_POINT('Ctrl Pts',(2.68436472026635,-1.79298789611831,300.196490910727));
#3830=CARTESIAN_POINT('Ctrl Pts',(2.81567899391501,-1.5695416581134,300.211305940885));
#3831=CARTESIAN_POINT('Ctrl Pts',(2.85070593620296,-1.50498636033014,300.215548419476));
#3832=CARTESIAN_POINT('Ctrl Pts',(2.91021508841622,-1.38576510259615,300.223369105823));
#3833=CARTESIAN_POINT('Ctrl Pts',(2.9354368293058,-1.33150544375763,300.226923130811));
#3834=CARTESIAN_POINT('Ctrl Pts',(2.97399257814137,-1.24213243752777,300.23278725562));
#3835=CARTESIAN_POINT('Ctrl Pts',(2.98824927242489,-1.20743155264031,300.235066471179));
#3836=CARTESIAN_POINT('Ctrl Pts',(3.01483452526991,-1.13936604599897,300.239545649583));
#3837=CARTESIAN_POINT('Ctrl Pts',(3.02722290768759,-1.10603051998512,300.241743253915));
#3838=CARTESIAN_POINT('Ctrl Pts',(3.05332859888578,-1.03205677830358,300.246631119012));
#3839=CARTESIAN_POINT('Ctrl Pts',(3.06679122154376,-0.991336498470313,300.249329131737));
#3840=CARTESIAN_POINT('Ctrl Pts',(3.11432475099745,-0.837314530139717,300.259566150404));
#3841=CARTESIAN_POINT('Ctrl Pts',(3.14295773488408,-0.72244431135342,300.267269751636));
#3842=CARTESIAN_POINT('Ctrl Pts',(3.20360838933636,-0.405800018996798,300.288640190842));
#3843=CARTESIAN_POINT('Ctrl Pts',(3.2228735108854,-0.202137207769175,300.302557468846));
#3844=CARTESIAN_POINT('Ctrl Pts',(3.22269570388895,0.0902716330811216,300.322059925417));
#3845=CARTESIAN_POINT('Ctrl Pts',(3.21901202739808,0.178551479280643,300.327878945683));
#3846=CARTESIAN_POINT('Ctrl Pts',(3.20923678664985,0.296324004970847,300.335462112288));
#3847=CARTESIAN_POINT('Ctrl Pts',(3.2063542597418,0.32603861213874,300.337359886027));
#3848=CARTESIAN_POINT('Ctrl Pts',(3.20082595493413,0.375819287096127,300.340508502232));
#3849=CARTESIAN_POINT('Ctrl Pts',(3.19840336453674,0.395907735287083,300.341770578645));
#3850=CARTESIAN_POINT('Ctrl Pts',(3.19279943956598,0.438960905865326,300.344455882313));
#3851=CARTESIAN_POINT('Ctrl Pts',(3.18955928743408,0.46191618620156,300.34587604657));
#3852=CARTESIAN_POINT('Ctrl Pts',(3.17929516344003,0.529366381325593,300.350019999086));
#3853=CARTESIAN_POINT('Ctrl Pts',(3.1715854860556,0.573752946201102,300.352709795304));
#3854=CARTESIAN_POINT('Ctrl Pts',(3.15097474687815,0.67924536015374,300.359044346623));
#3855=CARTESIAN_POINT('Ctrl Pts',(3.13722314816176,0.740167428901892,300.362655603398));
#3856=CARTESIAN_POINT('Ctrl Pts',(3.0686037815018,1.00771075404882,300.378452907558));
#3857=CARTESIAN_POINT('Ctrl Pts',(2.99502943570183,1.20897248037131,300.390206930343));
#3858=CARTESIAN_POINT('Ctrl Pts',(2.85441133976939,1.50015420372206,300.408655573263));
#3859=CARTESIAN_POINT('Ctrl Pts',(2.80175723048675,1.59633328673677,300.415004294568));
#3860=CARTESIAN_POINT('Ctrl Pts',(2.72020783428982,1.7287858037857,300.424249294867));
#3861=CARTESIAN_POINT('Ctrl Pts',(2.69527131926595,1.76741144565827,300.427008958671));
#3862=CARTESIAN_POINT('Ctrl Pts',(2.64973620397425,1.83473769581279,300.431941230587));
#3863=CARTESIAN_POINT('Ctrl Pts',(2.62947563826553,1.86365825170514,300.43410121707));
#3864=CARTESIAN_POINT('Ctrl Pts',(2.58573447791983,1.9239622097851,300.438696381022));
#3865=CARTESIAN_POINT('Ctrl Pts',(2.56214849305656,1.95526168648685,300.441135325997));
#3866=CARTESIAN_POINT('Ctrl Pts',(2.4956523392103,2.04023487135188,300.447910828199));
#3867=CARTESIAN_POINT('Ctrl Pts',(2.45158922512294,2.09297589327371,300.452291211085));
#3868=CARTESIAN_POINT('Ctrl Pts',(2.34647346527397,2.21091630712071,300.462503191567));
#3869=CARTESIAN_POINT('Ctrl Pts',(2.28433028802861,2.27506522200026,300.468372768338));
#3870=CARTESIAN_POINT('Ctrl Pts',(2.11060106485386,2.44009963479235,300.484313929542));
#3871=CARTESIAN_POINT('Ctrl Pts',(1.99448371141188,2.53589325896144,300.494501474038));
#3872=CARTESIAN_POINT('Ctrl Pts',(1.77172163757331,2.69487121418497,300.512901042201));
#3873=CARTESIAN_POINT('Ctrl Pts',(1.66729341278445,2.76070035370338,300.521121186726));
#3874=CARTESIAN_POINT('Ctrl Pts',(1.53127019096326,2.8359051379479,300.531123197489));
#3875=CARTESIAN_POINT('Ctrl Pts',(1.50296868845176,2.85100537518207,300.533167404367));
#3876=CARTESIAN_POINT('Ctrl Pts',(1.4579294875811,2.8741788658863,300.536357412042));
#3877=CARTESIAN_POINT('Ctrl Pts',(1.44133996765233,2.88253390110471,300.537519093158));
#3878=CARTESIAN_POINT('Ctrl Pts',(1.40533108078542,2.90028056584591,300.540010501111));
#3879=CARTESIAN_POINT('Ctrl Pts',(1.38588775254039,2.90962162574655,300.541337129728));
#3880=CARTESIAN_POINT('Ctrl Pts',(1.33291411002999,2.93441997828049,300.544905154062));
#3881=CARTESIAN_POINT('Ctrl Pts',(1.29920865155803,2.94949788421,300.547125496191));
#3882=CARTESIAN_POINT('Ctrl Pts',(1.22164211681965,2.98260896973022,300.552138436531));
#3883=CARTESIAN_POINT('Ctrl Pts',(1.17762673374779,3.00026022397891,300.554913747891));
#3884=CARTESIAN_POINT('Ctrl Pts',(1.02251021525017,3.05852586258049,300.564506150169));
#3885=CARTESIAN_POINT('Ctrl Pts',(0.909572631945766,3.09399227562682,300.571160358045));
#3886=CARTESIAN_POINT('Ctrl Pts',(0.592380749544747,3.17472662156811,300.589537762823));
#3887=CARTESIAN_POINT('Ctrl Pts',(0.385309314099095,3.20645157455163,300.601221245527));
#3888=CARTESIAN_POINT('Ctrl Pts',(0.11924498999209,3.22105594355245,300.616890936495));
#3889=CARTESIAN_POINT('Ctrl Pts',(0.0617867178307858,3.2226701001455,300.620310627769));
#3890=CARTESIAN_POINT('Ctrl Pts',(-0.0327533424388702,3.22279678224083,
300.626012371631));
#3891=CARTESIAN_POINT('Ctrl Pts',(-0.0698219772959573,3.22220679031655,
300.628266918268));
#3892=CARTESIAN_POINT('Ctrl Pts',(-0.143119248527061,3.2197748090424,300.632766185502));
#3893=CARTESIAN_POINT('Ctrl Pts',(-0.179343338382857,3.21796033846117,300.635009732994));
#3894=CARTESIAN_POINT('Ctrl Pts',(-0.26845426016443,3.21198749200961,300.640581159139));
#3895=CARTESIAN_POINT('Ctrl Pts',(-0.321282255254522,3.20713400559933,300.643929705222));
#3896=CARTESIAN_POINT('Ctrl Pts',(-0.571595807127612,3.17789036856934,300.660021811296));
#3897=CARTESIAN_POINT('Ctrl Pts',(-0.76663673476866,3.13655159098987,300.673268880885));
#3898=CARTESIAN_POINT('Ctrl Pts',(-1.13327903897695,3.02258661890292,300.699139630684));
#3899=CARTESIAN_POINT('Ctrl Pts',(-1.30491707642323,2.95255000672305,300.711685762921));
#3900=CARTESIAN_POINT('Ctrl Pts',(-1.50249764822595,2.85131274701742,300.726049926427));
#3901=CARTESIAN_POINT('Ctrl Pts',(-1.53509989300249,2.83389346046958,300.728416553639));
#3902=CARTESIAN_POINT('Ctrl Pts',(-1.58625053171304,2.80542196644905,300.732115667487));
#3903=CARTESIAN_POINT('Ctrl Pts',(-1.60499904813429,2.79473814081267,300.733468486261));
#3904=CARTESIAN_POINT('Ctrl Pts',(-1.64186948007166,2.77323413248643,300.736120744368));
#3905=CARTESIAN_POINT('Ctrl Pts',(-1.65999507255093,2.7624227312071,300.737420548346));
#3906=CARTESIAN_POINT('Ctrl Pts',(-1.70759825673703,2.73339103474394,300.740826968178));
#3907=CARTESIAN_POINT('Ctrl Pts',(-1.73689131474505,2.71487147602817,300.742915708644));
#3908=CARTESIAN_POINT('Ctrl Pts',(-1.80228878018694,2.67203423445684,300.747575270932));
#3909=CARTESIAN_POINT('Ctrl Pts',(-1.83821108902838,2.64745011647853,300.75013220325));
#3910=CARTESIAN_POINT('Ctrl Pts',(-1.95616650442604,2.56316632108192,300.758558001915));
#3911=CARTESIAN_POINT('Ctrl Pts',(-2.03588097144029,2.50031995960859,300.764302624803));
#3912=CARTESIAN_POINT('Ctrl Pts',(-2.29446550456624,2.27587385211834,300.783573153777));
#3913=CARTESIAN_POINT('Ctrl Pts',(-2.45812780828279,2.09804004724571,300.796938039432));
#3914=CARTESIAN_POINT('Ctrl Pts',(-2.63242613205356,1.85994147683927,300.814340667441));
#3915=CARTESIAN_POINT('Ctrl Pts',(-2.66330325905612,1.81545170442136,300.817570297326));
#3916=CARTESIAN_POINT('Ctrl Pts',(-2.71107379633234,1.74277763556684,300.822823996123));
#3917=CARTESIAN_POINT('Ctrl Pts',(-2.72868319503614,1.71507519279603,300.824821661315));
#3918=CARTESIAN_POINT('Ctrl Pts',(-2.76479379020732,1.65630315677302,300.829052232402));
#3919=CARTESIAN_POINT('Ctrl Pts',(-2.78320127632047,1.62518163270348,300.831288123116));
#3920=CARTESIAN_POINT('Ctrl Pts',(-2.82699392869198,1.54821464223496,300.836810342943));
#3921=CARTESIAN_POINT('Ctrl Pts',(-2.85179127982464,1.50204834970549,300.840116509032));
#3922=CARTESIAN_POINT('Ctrl Pts',(-2.9667859886612,1.27483633875973,300.856367389074));
#3923=CARTESIAN_POINT('Ctrl Pts',(-3.04091631812592,1.08620092052891,300.869836813035));
#3924=CARTESIAN_POINT('Ctrl Pts',(-3.1475341004324,0.715997393708384,300.895798573365));
#3925=CARTESIAN_POINT('Ctrl Pts',(-3.18311719071375,0.536094142515357,300.908205531704));
#3926=CARTESIAN_POINT('Ctrl Pts',(-3.20730253177424,0.317331048487601,300.922447022555));
#3927=CARTESIAN_POINT('Ctrl Pts',(-3.2107368651734,0.280459571292043,300.924818082341));
#3928=CARTESIAN_POINT('Ctrl Pts',(-3.21516675256344,0.222005647222841,300.928522451926));
#3929=CARTESIAN_POINT('Ctrl Pts',(-3.21658201609482,0.20045934514703,300.929876185759));
#3930=CARTESIAN_POINT('Ctrl Pts',(-3.2189515384922,0.157839926864977,300.932528664378));
#3931=CARTESIAN_POINT('Ctrl Pts',(-3.21991565688435,0.136768618924221,300.93382779728));
#3932=CARTESIAN_POINT('Ctrl Pts',(-3.22191471378086,0.0811166838642623,
300.937230097217));
#3933=CARTESIAN_POINT('Ctrl Pts',(-3.2225998757072,0.0465252055962028,300.939315468292));
#3934=CARTESIAN_POINT('Ctrl Pts',(-3.22288864827989,-0.0314966424706036,
300.94396607129));
#3935=CARTESIAN_POINT('Ctrl Pts',(-3.2221716767474,-0.0749219005992654,
300.946517494866));
#3936=CARTESIAN_POINT('Ctrl Pts',(-3.21686730992213,-0.219301100887406,
300.954915308994));
#3937=CARTESIAN_POINT('Ctrl Pts',(-3.20840994987354,-0.320056380476534,
300.960638327528));
#3938=CARTESIAN_POINT('Ctrl Pts',(-3.16369942792079,-0.659995996979792,
300.97993641725));
#3939=CARTESIAN_POINT('Ctrl Pts',(-3.10528972744827,-0.895407799953573,
300.993346292929));
#3940=CARTESIAN_POINT('Ctrl Pts',(-3.00229341645686,-1.17271960752348,301.010794604542));
#3941=CARTESIAN_POINT('Ctrl Pts',(-2.98221100881263,-1.22288758315954,301.014017570457));
#3942=CARTESIAN_POINT('Ctrl Pts',(-2.94792424387216,-1.30266512827609,301.01926341952));
#3943=CARTESIAN_POINT('Ctrl Pts',(-2.93451156287154,-1.33260479933907,301.021260057045));
#3944=CARTESIAN_POINT('Ctrl Pts',(-2.9053524022045,-1.39511778270642,301.025490853516));
#3945=CARTESIAN_POINT('Ctrl Pts',(-2.88950986822036,-1.42764097870992,301.027728034196));
#3946=CARTESIAN_POINT('Ctrl Pts',(-2.84933753465936,-1.50670180877295,301.033258582655));
#3947=CARTESIAN_POINT('Ctrl Pts',(-2.82441200657364,-1.55292338453925,301.036571927484));
#3948=CARTESIAN_POINT('Ctrl Pts',(-2.6984941959091,-1.77335604916429,301.052773858881));
#3949=CARTESIAN_POINT('Ctrl Pts',(-2.58246675679837,-1.93842875697878,301.066181520913));
#3950=CARTESIAN_POINT('Ctrl Pts',(-2.33256375633524,-2.23137379503876,301.092129107037));
#3951=CARTESIAN_POINT('Ctrl Pts',(-2.20156222920794,-2.3607234626445,301.104585821404));
#3952=CARTESIAN_POINT('Ctrl Pts',(-2.0317909080027,-2.50186175628897,301.118870968421));
#3953=CARTESIAN_POINT('Ctrl Pts',(-2.00293249205562,-2.52502440325386,301.121240256945));
#3954=CARTESIAN_POINT('Ctrl Pts',(-1.95661584113431,-2.56090569265645,301.12494252647));
#3955=CARTESIAN_POINT('Ctrl Pts',(-1.93941849782901,-2.57395405316969,301.126295894764));
#3956=CARTESIAN_POINT('Ctrl Pts',(-1.9051566948386,-2.59941159004449,301.128948284674));
#3957=CARTESIAN_POINT('Ctrl Pts',(-1.88809905231737,-2.61182783853808,301.130247685034));
#3958=CARTESIAN_POINT('Ctrl Pts',(-1.842733441423,-2.64417272576674,301.133651627648));
#3959=CARTESIAN_POINT('Ctrl Pts',(-1.81422333950115,-2.66381490141667,301.135738342283));
#3960=CARTESIAN_POINT('Ctrl Pts',(-1.74921659064302,-2.707073695116,301.140392517317));
#3961=CARTESIAN_POINT('Ctrl Pts',(-1.71254714705836,-2.73041924794202,301.142946137042));
#3962=CARTESIAN_POINT('Ctrl Pts',(-1.61011183487701,-2.79275874012439,301.149915900342));
#3963=CARTESIAN_POINT('Ctrl Pts',(-1.54341903546483,-2.83016214338351,301.154272772181));
#3964=CARTESIAN_POINT('Ctrl Pts',(-1.47546399521001,-2.86515681269611,301.158594111703));
#3965=CARTESIAN_POINT('Origin',(0.,0.,294.689226550727));
#3966=CARTESIAN_POINT('',(-1.47546411936631,-2.86515674875958,302.651619072379));
#3967=CARTESIAN_POINT('',(-1.47546400229876,-2.86515680904563,302.404343180173));
#3968=CARTESIAN_POINT('',(-1.47546400239267,-2.86515680899727,294.689226550727));
#3969=CARTESIAN_POINT('Ctrl Pts',(-1.47546411936631,-2.86515674875959,302.651619072379));
#3970=CARTESIAN_POINT('Ctrl Pts',(-1.56656438462051,-2.81824302485756,302.64575923233));
#3971=CARTESIAN_POINT('Ctrl Pts',(-1.65541897282013,-2.76698859902053,302.640007807061));
#3972=CARTESIAN_POINT('Ctrl Pts',(-1.91531531524237,-2.60004896160934,302.622671394209));
#3973=CARTESIAN_POINT('Ctrl Pts',(-2.07778607985001,-2.47214113131752,302.611090056498));
#3974=CARTESIAN_POINT('Ctrl Pts',(-2.26472861339141,-2.29343823920053,302.595812134333));
#3975=CARTESIAN_POINT('Ctrl Pts',(-2.30165889047301,-2.25637331781722,302.592687368049));
#3976=CARTESIAN_POINT('Ctrl Pts',(-2.36252943902848,-2.19223094090484,302.587340313719));
#3977=CARTESIAN_POINT('Ctrl Pts',(-2.38694675230375,-2.16561928537802,302.585138610119));
#3978=CARTESIAN_POINT('Ctrl Pts',(-2.43267313848977,-2.11407058303965,302.580901855647));
#3979=CARTESIAN_POINT('Ctrl Pts',(-2.4540589104674,-2.08920744993729,302.578870341943));
#3980=CARTESIAN_POINT('Ctrl Pts',(-2.50971667940753,-2.02246576596436,302.573445936145));
#3981=CARTESIAN_POINT('Ctrl Pts',(-2.54331852224081,-1.98004442556283,302.570027342711));
#3982=CARTESIAN_POINT('Ctrl Pts',(-2.72072706728567,-1.74410094828758,302.551159292584));
#3983=CARTESIAN_POINT('Ctrl Pts',(-2.84351759392912,-1.53577877699471,302.534938617956));
#3984=CARTESIAN_POINT('Ctrl Pts',(-2.98332211902242,-1.22318859500695,302.511857830567));
#3985=CARTESIAN_POINT('Ctrl Pts',(-3.02033385479007,-1.12871009162387,302.505043086966));
#3986=CARTESIAN_POINT('Ctrl Pts',(-3.06676937987678,-0.991431085146797,
302.495489658053));
#3987=CARTESIAN_POINT('Ctrl Pts',(-3.07987334170464,-0.949942399395154,
302.492646856339));
#3988=CARTESIAN_POINT('Ctrl Pts',(-3.10189393394382,-0.874969193126422,
302.487603449932));
#3989=CARTESIAN_POINT('Ctrl Pts',(-3.11111821030993,-0.841582300140183,
302.485390425793));
#3990=CARTESIAN_POINT('Ctrl Pts',(-3.12508986566979,-0.787639204586613,
302.481874467981));
#3991=CARTESIAN_POINT('Ctrl Pts',(-3.13017660022288,-0.767174495895574,
302.480554280439));
#3992=CARTESIAN_POINT('Ctrl Pts',(-3.14005460400588,-0.725698943893595,
302.477908284888));
#3993=CARTESIAN_POINT('Ctrl Pts',(-3.14483671463996,-0.70468714461658,302.476582981906));
#3994=CARTESIAN_POINT('Ctrl Pts',(-3.15723122900629,-0.647586843247663,
302.473018615286));
#3995=CARTESIAN_POINT('Ctrl Pts',(-3.16443569996564,-0.611412061202154,
302.470800561102));
#3996=CARTESIAN_POINT('Ctrl Pts',(-3.20435211868759,-0.391326344860414,
302.457505079968));
#3997=CARTESIAN_POINT('Ctrl Pts',(-3.22164780622963,-0.204961933966709,
302.447071438326));
#3998=CARTESIAN_POINT('Ctrl Pts',(-3.22379022441715,0.175815524642427,302.425699773419));
#3999=CARTESIAN_POINT('Ctrl Pts',(-3.20737182576775,0.369447017497268,302.414790748178));
#4000=CARTESIAN_POINT('Ctrl Pts',(-3.16415676457459,0.61417357292202,302.400140325852));
#4001=CARTESIAN_POINT('Ctrl Pts',(-3.15330078481984,0.667675715121783,302.396885718481));
#4002=CARTESIAN_POINT('Ctrl Pts',(-3.13292411498144,0.756463732439752,302.391384007003));
#4003=CARTESIAN_POINT('Ctrl Pts',(-3.12415238958639,0.79191070801318,302.389160470346));
#4004=CARTESIAN_POINT('Ctrl Pts',(-3.10536110910862,0.862668348410636,302.384663819488));
#4005=CARTESIAN_POINT('Ctrl Pts',(-3.09533685573578,0.897972089385883,302.382390847854));
#4006=CARTESIAN_POINT('Ctrl Pts',(-3.06861588434326,0.986308681147351,302.376625948904));
#4007=CARTESIAN_POINT('Ctrl Pts',(-3.05114613632413,1.03909331470047,302.373109960628));
#4008=CARTESIAN_POINT('Ctrl Pts',(-2.95462849305133,1.30725639273526,302.354869912481));
#4009=CARTESIAN_POINT('Ctrl Pts',(-2.8541196202872,1.51417295134879,302.339462691277));
#4010=CARTESIAN_POINT('Ctrl Pts',(-2.67576667315583,1.79940280879597,302.316779962849));
#4011=CARTESIAN_POINT('Ctrl Pts',(-2.61451986611871,1.88729054299005,302.309574931153));
#4012=CARTESIAN_POINT('Ctrl Pts',(-2.52156037207488,2.00745194194057,302.299548616362));
#4013=CARTESIAN_POINT('Ctrl Pts',(-2.49337163801645,2.0423585012062,302.296613850176));
#4014=CARTESIAN_POINT('Ctrl Pts',(-2.4416299200101,2.10376243584213,302.291426720655));
#4015=CARTESIAN_POINT('Ctrl Pts',(-2.4183513724015,2.13048114905897,302.289160939516));
#4016=CARTESIAN_POINT('Ctrl Pts',(-2.38041491842719,2.17260072413725,302.285582393459));
#4017=CARTESIAN_POINT('Ctrl Pts',(-2.36603768715614,2.18824925812226,302.284251333726));
#4018=CARTESIAN_POINT('Ctrl Pts',(-2.33689435565397,2.21934651106358,302.281605160707));
#4019=CARTESIAN_POINT('Ctrl Pts',(-2.32212729530856,2.23479284252099,302.280290225134));
#4020=CARTESIAN_POINT('Ctrl Pts',(-2.28206572295433,2.27587132439407,302.276788004346));
#4021=CARTESIAN_POINT('Ctrl Pts',(-2.25649275148975,2.30122900869434,302.274620491556));
#4022=CARTESIAN_POINT('Ctrl Pts',(-2.0882200306413,2.46258210535103,302.260748662559));
#4023=CARTESIAN_POINT('Ctrl Pts',(-1.93370768469685,2.58568475220007,302.249771553372));
#4024=CARTESIAN_POINT('Ctrl Pts',(-1.66145228858582,2.76445584120435,302.231486883426));
#4025=CARTESIAN_POINT('Ctrl Pts',(-1.54988579555216,2.82851398050596,302.224252481611));
#4026=CARTESIAN_POINT('Ctrl Pts',(-1.37991781639501,2.91302260255444,302.213305399926));
#4027=CARTESIAN_POINT('Ctrl Pts',(-1.32427353579774,2.93873660972428,302.209733657307));
#4028=CARTESIAN_POINT('Ctrl Pts',(-1.21973264267542,2.98347423135796,302.203016785893));
#4029=CARTESIAN_POINT('Ctrl Pts',(-1.17103919381826,3.00292073834523,302.199885701727));
#4030=CARTESIAN_POINT('Ctrl Pts',(-1.08802130321314,3.03374897795421,302.194531160167));
#4031=CARTESIAN_POINT('Ctrl Pts',(-1.05393953784335,3.0457568036242,302.19232842976));
#4032=CARTESIAN_POINT('Ctrl Pts',(-0.988572549668914,3.06755865422687,302.188091905358));
#4033=CARTESIAN_POINT('Ctrl Pts',(-0.957325554598902,3.07745340207265,302.186061685676));
#4034=CARTESIAN_POINT('Ctrl Pts',(-0.874217056372091,3.10238253447798,302.180646149307));
#4035=CARTESIAN_POINT('Ctrl Pts',(-0.822121093078396,3.11659256418156,302.17723529002));
#4036=CARTESIAN_POINT('Ctrl Pts',(-0.534734637313234,3.18727506797976,302.158321240372));
#4037=CARTESIAN_POINT('Ctrl Pts',(-0.294046051273407,3.21841030503454,302.142040006514));
#4038=CARTESIAN_POINT('Ctrl Pts',(0.0488040166192698,3.22396307333619,302.118928632269));
#4039=CARTESIAN_POINT('Ctrl Pts',(0.149822360850706,3.22085001862124,302.112141712529));
#4040=CARTESIAN_POINT('Ctrl Pts',(0.293803765892632,3.20962315128552,302.102622143149));
#4041=CARTESIAN_POINT('Ctrl Pts',(0.337005318291248,3.20537504464777,302.099786040111));
#4042=CARTESIAN_POINT('Ctrl Pts',(0.414443646400678,3.19617732247638,302.094753126921));
#4043=CARTESIAN_POINT('Ctrl Pts',(0.448711350365809,3.19154685941951,302.092543968812));
#4044=CARTESIAN_POINT('Ctrl Pts',(0.503735729571337,3.18320781614914,302.089032591804));
#4045=CARTESIAN_POINT('Ctrl Pts',(0.524541397496784,3.17984560624032,302.087713194817));
#4046=CARTESIAN_POINT('Ctrl Pts',(0.566564256985201,3.17263099243986,302.085067163379));
#4047=CARTESIAN_POINT('Ctrl Pts',(0.587778634801142,3.16876928921676,302.08374105874));
#4048=CARTESIAN_POINT('Ctrl Pts',(0.645235979904885,3.15771329676716,302.080171880853));
#4049=CARTESIAN_POINT('Ctrl Pts',(0.681397589133606,3.15010798481078,302.077949914051));
#4050=CARTESIAN_POINT('Ctrl Pts',(0.897744417873805,3.1007070259585,302.064760139779));
#4051=CARTESIAN_POINT('Ctrl Pts',(1.07420751899143,3.04407984601912,302.054422639236));
#4052=CARTESIAN_POINT('Ctrl Pts',(1.43026140794561,2.89497410757814,302.032757840055));
#4053=CARTESIAN_POINT('Ctrl Pts',(1.60798110297047,2.80016234396717,302.021455452306));
#4054=CARTESIAN_POINT('Ctrl Pts',(1.81920805949189,2.66069861594447,302.006499871361));
#4055=CARTESIAN_POINT('Ctrl Pts',(1.86200579665291,2.63092551290022,302.003385827147));
#4056=CARTESIAN_POINT('Ctrl Pts',(1.93317278980825,2.57881028805522,301.998051469096));
#4057=CARTESIAN_POINT('Ctrl Pts',(1.96192358729006,2.5570051259342,301.995851498389));
#4058=CARTESIAN_POINT('Ctrl Pts',(2.0161201967694,2.514449151445,301.991614305894));
#4059=CARTESIAN_POINT('Ctrl Pts',(2.04162699176136,2.49378312715198,301.989580557835));
#4060=CARTESIAN_POINT('Ctrl Pts',(2.10848674787075,2.43789893586445,301.984140866892));
#4061=CARTESIAN_POINT('Ctrl Pts',(2.14927120629997,2.4020200478917,301.98070894846));
#4062=CARTESIAN_POINT('Ctrl Pts',(2.36495365537342,2.20238765548299,301.961921166423));
#4063=CARTESIAN_POINT('Ctrl Pts',(2.52205919402392,2.02056925855705,301.94580587386));
#4064=CARTESIAN_POINT('Ctrl Pts',(2.71531123660843,1.73885874569804,301.92277803093));
#4065=CARTESIAN_POINT('Ctrl Pts',(2.76904364975881,1.65195157013254,301.915914495822));
#4066=CARTESIAN_POINT('Ctrl Pts',(2.83973796607326,1.52443870867897,301.906301739341));
#4067=CARTESIAN_POINT('Ctrl Pts',(2.86013738222023,1.4858127700909,301.903447237298));
#4068=CARTESIAN_POINT('Ctrl Pts',(2.89534016064232,1.41574344741609,301.898385510776));
#4069=CARTESIAN_POINT('Ctrl Pts',(2.91043202295578,1.38445289422434,301.89616574158));
#4070=CARTESIAN_POINT('Ctrl Pts',(2.93387639192436,1.33376623706746,301.892641789615));
#4071=CARTESIAN_POINT('Ctrl Pts',(2.94254903237091,1.31452208804738,301.891320220605));
#4072=CARTESIAN_POINT('Ctrl Pts',(2.95968256914594,1.27548419470277,301.888674270965));
#4073=CARTESIAN_POINT('Ctrl Pts',(2.96813544250033,1.25568821610776,301.887350352388));
#4074=CARTESIAN_POINT('Ctrl Pts',(2.99048739567302,1.20185452999884,301.883794292138));
#4075=CARTESIAN_POINT('Ctrl Pts',(3.00400379852611,1.16766031279254,301.881582992887));
#4076=CARTESIAN_POINT('Ctrl Pts',(3.08335823294515,0.956401588420554,301.868167115089));
#4077=CARTESIAN_POINT('Ctrl Pts',(3.13411434422543,0.774044499453227,301.857622396741));
#4078=CARTESIAN_POINT('Ctrl Pts',(3.20455820707267,0.394614957239556,301.835962098765));
#4079=CARTESIAN_POINT('Ctrl Pts',(3.22267989304969,0.198086985339928,301.824875396434));
#4080=CARTESIAN_POINT('Ctrl Pts',(3.2227683696409,-0.0511815540635796,301.810149796668));
#4081=CARTESIAN_POINT('Ctrl Pts',(3.22151258882781,-0.103497361171781,301.807024556326));
#4082=CARTESIAN_POINT('Ctrl Pts',(3.21725571438089,-0.191472727016841,301.801698658033));
#4083=CARTESIAN_POINT('Ctrl Pts',(3.21493332152809,-0.227155714872538,301.79951894891));
#4084=CARTESIAN_POINT('Ctrl Pts',(3.2089920367645,-0.299774134902215,301.795039839523));
#4085=CARTESIAN_POINT('Ctrl Pts',(3.20532792537239,-0.336700364262504,301.792739368845));
#4086=CARTESIAN_POINT('Ctrl Pts',(3.19432777379486,-0.430961944822834,301.786805157277));
#4087=CARTESIAN_POINT('Ctrl Pts',(3.18608559544938,-0.488176230768828,301.783144327156));
#4088=CARTESIAN_POINT('Ctrl Pts',(3.14761330287636,-0.712340654620758,301.768561188446));
#4089=CARTESIAN_POINT('Ctrl Pts',(3.10576228328249,-0.876998414390794,301.757302235601));
#4090=CARTESIAN_POINT('Ctrl Pts',(2.9840092915615,-1.23503121957962,301.731865741436));
#4091=CARTESIAN_POINT('Ctrl Pts',(2.89785219803998,-1.4255089947519,301.717661870415));
#4092=CARTESIAN_POINT('Ctrl Pts',(2.77659228961666,-1.63641589213254,301.701958606608));
#4093=CARTESIAN_POINT('Ctrl Pts',(2.75881057115451,-1.66621912379549,301.699741156993));
#4094=CARTESIAN_POINT('Ctrl Pts',(2.72944803908689,-1.71367329428893,301.69621995445));
#4095=CARTESIAN_POINT('Ctrl Pts',(2.71816955541944,-1.73150717457507,301.694898860826));
#4096=CARTESIAN_POINT('Ctrl Pts',(2.69502918049024,-1.76731403851098,301.692252897774));
#4097=CARTESIAN_POINT('Ctrl Pts',(2.68316075152255,-1.7852813884695,301.69092850514));
#4098=CARTESIAN_POINT('Ctrl Pts',(2.65052081746639,-1.83363341619955,301.687369600883));
#4099=CARTESIAN_POINT('Ctrl Pts',(2.62940687895751,-1.8637842759102,301.685155988814));
#4100=CARTESIAN_POINT('Ctrl Pts',(2.58003224384247,-1.93178192756879,301.680160560483));
#4101=CARTESIAN_POINT('Ctrl Pts',(2.55144649945041,-1.96938288788776,301.677395867025));
#4102=CARTESIAN_POINT('Ctrl Pts',(2.44891702201815,-2.0982659926791,301.667860058194));
#4103=CARTESIAN_POINT('Ctrl Pts',(2.37081574605065,-2.18612680372307,301.661249907815));
#4104=CARTESIAN_POINT('Ctrl Pts',(2.13991237667403,-2.41891817201873,301.642838775936));
#4105=CARTESIAN_POINT('Ctrl Pts',(1.97747714127827,-2.55342223537591,301.631081348385));
#4106=CARTESIAN_POINT('Ctrl Pts',(1.75555322046565,-2.70322791916428,301.615334616756));
#4107=CARTESIAN_POINT('Ctrl Pts',(1.70716094770546,-2.73404630690465,301.611921168019));
#4108=CARTESIAN_POINT('Ctrl Pts',(1.62622434022472,-2.78260360629044,301.606228559067));
#4109=CARTESIAN_POINT('Ctrl Pts',(1.59414976631164,-2.80110242310004,301.603976777764));
#4110=CARTESIAN_POINT('Ctrl Pts',(1.53006749377038,-2.83660432526885,301.59948223923));
#4111=CARTESIAN_POINT('Ctrl Pts',(1.4980775519221,-2.8536282370309,301.597240637826));
#4112=CARTESIAN_POINT('Ctrl Pts',(1.4185909733147,-2.89422324797366,301.591672818702));
#4113=CARTESIAN_POINT('Ctrl Pts',(1.3707880605459,-2.91716782707154,301.58832593936));
#4114=CARTESIAN_POINT('Ctrl Pts',(1.14094417933643,-3.02059196120465,301.572232368835));
#4115=CARTESIAN_POINT('Ctrl Pts',(0.952295632917648,-3.08526193892359,301.55898181711));
#4116=CARTESIAN_POINT('Ctrl Pts',(0.579113941289261,-3.17568448021665,301.533108715446));
#4117=CARTESIAN_POINT('Ctrl Pts',(0.395881850157772,-3.20369026392042,301.520563825996));
#4118=CARTESIAN_POINT('Ctrl Pts',(0.17438515354406,-3.21824054881868,301.506201888283));
#4119=CARTESIAN_POINT('Ctrl Pts',(0.137480016494186,-3.22002824818947,301.503836268437));
#4120=CARTESIAN_POINT('Ctrl Pts',(0.079000232393424,-3.22185372047421,301.500139196589));
#4121=CARTESIAN_POINT('Ctrl Pts',(0.0574429559807811,-3.22231016516788,
301.498787422204));
#4122=CARTESIAN_POINT('Ctrl Pts',(0.0148080076377847,-3.22278489118032,
301.496137951778));
#4123=CARTESIAN_POINT('Ctrl Pts',(-0.00626830765275662,-3.22281282164261,
301.494839880365));
#4124=CARTESIAN_POINT('Ctrl Pts',(-0.061921713059651,-3.22234060509785,
301.491439573036));
#4125=CARTESIAN_POINT('Ctrl Pts',(-0.0964941240447321,-3.22149070648021,
301.489355124637));
#4126=CARTESIAN_POINT('Ctrl Pts',(-0.174421625000267,-3.21831929344846,
301.484706299137));
#4127=CARTESIAN_POINT('Ctrl Pts',(-0.217757399199872,-3.21567784775963,
301.482155726233));
#4128=CARTESIAN_POINT('Ctrl Pts',(-0.361726871689196,-3.20397852348821,
301.473759695828));
#4129=CARTESIAN_POINT('Ctrl Pts',(-0.461990600573863,-3.19106434030277,
301.468037600735));
#4130=CARTESIAN_POINT('Ctrl Pts',(-0.799674924297983,-3.13131717494294,
301.448735910623));
#4131=CARTESIAN_POINT('Ctrl Pts',(-1.03234034105093,-3.06249755699573,301.435321826378));
#4132=CARTESIAN_POINT('Ctrl Pts',(-1.30484839411577,-2.9472706346054,301.417870478235));
#4133=CARTESIAN_POINT('Ctrl Pts',(-1.35404585412848,-2.92499450542626,301.414649420727));
#4134=CARTESIAN_POINT('Ctrl Pts',(-1.42707972997024,-2.88968800765593,301.409748711068));
#4135=CARTESIAN_POINT('Ctrl Pts',(-1.45135013935263,-2.87757467623773,301.408099925956));
#4136=CARTESIAN_POINT('Ctrl Pts',(-1.47546400249216,-2.86515680894603,301.40644069294));
#4137=CARTESIAN_POINT('',(3.22274880669402,-0.00279346863476049,301.56427538288));
#4138=CARTESIAN_POINT('Ctrl Pts',(-1.47546399521001,-2.86515681269611,301.158594111703));
#4139=CARTESIAN_POINT('Ctrl Pts',(-1.45345302210279,-2.87649175889358,301.159993814913));
#4140=CARTESIAN_POINT('Ctrl Pts',(-1.43130962004888,-2.88757399582668,301.161389750391));
#4141=CARTESIAN_POINT('Ctrl Pts',(-1.19187476928135,-3.00397362883705,301.176373801413));
#4142=CARTESIAN_POINT('Ctrl Pts',(-0.963554646627904,-3.08479757827593,
301.189765730589));
#4143=CARTESIAN_POINT('Ctrl Pts',(-0.67567640453847,-3.15158745199416,301.207195819349));
#4144=CARTESIAN_POINT('Ctrl Pts',(-0.622700029955293,-3.16248102737201,
301.210421449546));
#4145=CARTESIAN_POINT('Ctrl Pts',(-0.537179844503203,-3.17783449708863,
301.215670436555));
#4146=CARTESIAN_POINT('Ctrl Pts',(-0.504797159632848,-3.18313901417946,
301.217667484575));
#4147=CARTESIAN_POINT('Ctrl Pts',(-0.436562901552625,-3.19324889349919,
301.221898188511));
#4148=CARTESIAN_POINT('Ctrl Pts',(-0.400700296424094,-3.19794696163251,
301.224134851375));
#4149=CARTESIAN_POINT('Ctrl Pts',(-0.312639634462214,-3.20797858158073,
301.229662058633));
#4150=CARTESIAN_POINT('Ctrl Pts',(-0.260377280503483,-3.21264272649583,
301.232972523859));
#4151=CARTESIAN_POINT('Ctrl Pts',(-0.00891327128532342,-3.22890850617758,
301.249054300625));
#4152=CARTESIAN_POINT('Ctrl Pts',(0.190937645520774,-3.22326711999056,301.262334276149));
#4153=CARTESIAN_POINT('Ctrl Pts',(0.573394765673103,-3.17676829414263,301.288293177993));
#4154=CARTESIAN_POINT('Ctrl Pts',(0.755561025127526,-3.13843508525341,301.300893813444));
#4155=CARTESIAN_POINT('Ctrl Pts',(0.968768863344022,-3.07391746421563,301.315306053339));
#4156=CARTESIAN_POINT('Ctrl Pts',(1.00393506550612,-3.06261266465628,301.317671001378));
#4157=CARTESIAN_POINT('Ctrl Pts',(1.05932161465258,-3.04375108223454,301.321368124114));
#4158=CARTESIAN_POINT('Ctrl Pts',(1.0796727843825,-3.03659178579029,301.322720596174));
#4159=CARTESIAN_POINT('Ctrl Pts',(1.11979215424178,-3.02202393484573,301.325372772496));
#4160=CARTESIAN_POINT('Ctrl Pts',(1.13956234063291,-3.01462449521813,301.326672832493));
#4161=CARTESIAN_POINT('Ctrl Pts',(1.1916124558994,-2.99455833836158,301.33008082218));
#4162=CARTESIAN_POINT('Ctrl Pts',(1.2237640766479,-2.9815636145052,301.332170846201));
#4163=CARTESIAN_POINT('Ctrl Pts',(1.29581865757841,-2.95107930363049,301.336833822585));
#4164=CARTESIAN_POINT('Ctrl Pts',(1.33558973665409,-2.93329429745238,301.339392854454));
#4165=CARTESIAN_POINT('Ctrl Pts',(1.46687736253742,-2.87136042617462,301.347829335986));
#4166=CARTESIAN_POINT('Ctrl Pts',(1.55666905542917,-2.82368971380537,301.353582208836));
#4167=CARTESIAN_POINT('Ctrl Pts',(1.85101869968063,-2.64910286229942,301.37284228792));
#4168=CARTESIAN_POINT('Ctrl Pts',(2.04355862119677,-2.50357244306358,301.386190049781));
#4169=CARTESIAN_POINT('Ctrl Pts',(2.25742016995655,-2.30067568172881,301.403575289066));
#4170=CARTESIAN_POINT('Ctrl Pts',(2.29578594176301,-2.26239272176716,301.406807441956));
#4171=CARTESIAN_POINT('Ctrl Pts',(2.35581519136251,-2.1993931589936,301.412064113639));
#4172=CARTESIAN_POINT('Ctrl Pts',(2.37809841184491,-2.17528005250291,301.414062168775));
#4173=CARTESIAN_POINT('Ctrl Pts',(2.4241344834076,-2.1239106258541,301.418292659971));
#4174=CARTESIAN_POINT('Ctrl Pts',(2.44780475724229,-2.09658676068211,301.420528066935));
#4175=CARTESIAN_POINT('Ctrl Pts',(2.50462148480605,-2.02872624173379,301.426047158583));
#4176=CARTESIAN_POINT('Ctrl Pts',(2.53724832293572,-1.98776995455119,301.429350627678));
#4177=CARTESIAN_POINT('Ctrl Pts',(2.68811908316454,-1.78861355191994,301.445294303723));
#4178=CARTESIAN_POINT('Ctrl Pts',(2.79263630709289,-1.62058143652535,301.458431928333));
#4179=CARTESIAN_POINT('Ctrl Pts',(2.96547294622877,-1.27574936145966,301.48441684266));
#4180=CARTESIAN_POINT('Ctrl Pts',(3.03493041119149,-1.10035112917256,301.497192056638));
#4181=CARTESIAN_POINT('Ctrl Pts',(3.09918741784172,-0.884596233552232,301.511755564093));
#4182=CARTESIAN_POINT('Ctrl Pts',(3.10909165297782,-0.849130437892967,301.514112857249));
#4183=CARTESIAN_POINT('Ctrl Pts',(3.12382578344141,-0.792650226447109,301.517800901707));
#4184=CARTESIAN_POINT('Ctrl Pts',(3.12905610741522,-0.771744675550877,301.519151792119));
#4185=CARTESIAN_POINT('Ctrl Pts',(3.13899883674654,-0.730239893023231,301.521803605958));
#4186=CARTESIAN_POINT('Ctrl Pts',(3.14371909013409,-0.709643802145879,301.523104844375));
#4187=CARTESIAN_POINT('Ctrl Pts',(3.15567145248582,-0.655030244662248,301.526520049407));
#4188=CARTESIAN_POINT('Ctrl Pts',(3.16255631306451,-0.620938581176801,301.528615971018));
#4189=CARTESIAN_POINT('Ctrl Pts',(3.2045479384828,-0.394148823274494,301.542360648955));
#4190=CARTESIAN_POINT('Ctrl Pts',(3.22257899414355,-0.198690636089394,301.553279316752));
#4191=CARTESIAN_POINT('Ctrl Pts',(3.22274878942769,-0.00279333892986146,
301.564275417346));
#4192=CARTESIAN_POINT('Ctrl Pts',(3.22274878931396,-0.00279347014087786,
301.564275409981));
#4193=CARTESIAN_POINT('Ctrl Pts',(3.22287158591405,0.138873551275113,301.572227458523));
#4194=CARTESIAN_POINT('Ctrl Pts',(3.21365306475287,0.280392099962546,301.580196534937));
#4195=CARTESIAN_POINT('Ctrl Pts',(3.18615340785927,0.48917779355849,301.59238269485));
#4196=CARTESIAN_POINT('Ctrl Pts',(3.17496313149674,0.557204328551994,301.596420487291));
#4197=CARTESIAN_POINT('Ctrl Pts',(3.15461619497305,0.660160745287787,301.602666014397));
#4198=CARTESIAN_POINT('Ctrl Pts',(3.14703931863876,0.695384011309783,301.604826884526));
#4199=CARTESIAN_POINT('Ctrl Pts',(3.13070004798135,0.765594666178743,301.609187089066));
#4200=CARTESIAN_POINT('Ctrl Pts',(3.12193767200957,0.8005766640351,301.611386142309));
#4201=CARTESIAN_POINT('Ctrl Pts',(3.10405568489855,0.867202336719626,301.615628739179));
#4202=CARTESIAN_POINT('Ctrl Pts',(3.09503442337277,0.898867832612129,301.617668921201));
#4203=CARTESIAN_POINT('Ctrl Pts',(3.06971960605143,0.982821590140605,301.623143998793));
#4204=CARTESIAN_POINT('Ctrl Pts',(3.05257624269807,1.03484030065757,301.626605459846));
#4205=CARTESIAN_POINT('Ctrl Pts',(2.95360986286981,1.31123668505557,301.64538058451));
#4206=CARTESIAN_POINT('Ctrl Pts',(2.84837063316787,1.52640217195652,301.661446270562));
#4207=CARTESIAN_POINT('Ctrl Pts',(2.6656750606014,1.8140277932332,301.684414546406));
#4208=CARTESIAN_POINT('Ctrl Pts',(2.60693032213581,1.89748162865093,301.691269811311));
#4209=CARTESIAN_POINT('Ctrl Pts',(2.51752931484781,2.01247847508349,301.700873254601));
#4210=CARTESIAN_POINT('Ctrl Pts',(2.49003558251926,2.04639844646671,301.703726485868));
#4211=CARTESIAN_POINT('Ctrl Pts',(2.43944647981816,2.10628220260853,301.708786642058));
#4212=CARTESIAN_POINT('Ctrl Pts',(2.41660452503261,2.13245085202524,301.711006090195));
#4213=CARTESIAN_POINT('Ctrl Pts',(2.37919927561547,2.17393063652948,301.714530520455));
#4214=CARTESIAN_POINT('Ctrl Pts',(2.36490119351079,2.1894761978161,301.71585287147));
#4215=CARTESIAN_POINT('Ctrl Pts',(2.33570088624363,2.22060436033124,301.71850172955));
#4216=CARTESIAN_POINT('Ctrl Pts',(2.32079313343711,2.2361801464205,301.719827752613));
#4217=CARTESIAN_POINT('Ctrl Pts',(2.27997095098759,2.27798361178716,301.723392142715));
#4218=CARTESIAN_POINT('Ctrl Pts',(2.25376021386129,2.30391884101336,301.725609529387));
#4219=CARTESIAN_POINT('Ctrl Pts',(2.09167769295594,2.45888384330308,301.738939017457));
#4220=CARTESIAN_POINT('Ctrl Pts',(1.94519681351087,2.57632489684497,301.749403057776));
#4221=CARTESIAN_POINT('Ctrl Pts',(1.62430013811067,2.79054410764109,301.771058122628));
#4222=CARTESIAN_POINT('Ctrl Pts',(1.44947065991038,2.8852230324201,301.782222005566));
#4223=CARTESIAN_POINT('Ctrl Pts',(1.21896518470082,2.98378566006795,301.797032378625));
#4224=CARTESIAN_POINT('Ctrl Pts',(1.17038442105278,3.00317379486243,301.800156288271));
#4225=CARTESIAN_POINT('Ctrl Pts',(1.0874739329138,3.03394529973871,301.805504018538));
#4226=CARTESIAN_POINT('Ctrl Pts',(1.05338452070672,3.04594887133107,301.807707301554));
#4227=CARTESIAN_POINT('Ctrl Pts',(0.987945107899092,3.06776149632866,301.811948647647));
#4228=CARTESIAN_POINT('Ctrl Pts',(0.956632753284695,3.0776695380587,301.813983191352));
#4229=CARTESIAN_POINT('Ctrl Pts',(0.873204846717059,3.10267213418293,301.819419792711));
#4230=CARTESIAN_POINT('Ctrl Pts',(0.820851999292563,3.11693158649496,301.822847722402));
#4231=CARTESIAN_POINT('Ctrl Pts',(0.534896372227233,3.18711408463789,301.841669465062));
#4232=CARTESIAN_POINT('Ctrl Pts',(0.295989141550298,3.21809975154081,301.857827407001));
#4233=CARTESIAN_POINT('Ctrl Pts',(-0.0458887649501769,3.22403113455179,
301.88087526916));
#4234=CARTESIAN_POINT('Ctrl Pts',(-0.147713212640572,3.22097271185103,301.887717702485));
#4235=CARTESIAN_POINT('Ctrl Pts',(-0.29270660207025,3.20972621046373,301.897305546022));
#4236=CARTESIAN_POINT('Ctrl Pts',(-0.336116277435697,3.20547121158965,301.900155702934));
#4237=CARTESIAN_POINT('Ctrl Pts',(-0.413891417913324,3.19625028357872,301.905211045777));
#4238=CARTESIAN_POINT('Ctrl Pts',(-0.448288151853629,3.19160773519085,301.907428721981));
#4239=CARTESIAN_POINT('Ctrl Pts',(-0.503480920506684,3.18324839413136,301.910951052349));
#4240=CARTESIAN_POINT('Ctrl Pts',(-0.524326378966687,3.17988133347345,301.9122730406));
#4241=CARTESIAN_POINT('Ctrl Pts',(-0.566392654434734,3.17266165670944,301.914921911329));
#4242=CARTESIAN_POINT('Ctrl Pts',(-0.587610786301522,3.16880044356729,301.916248298498));
#4243=CARTESIAN_POINT('Ctrl Pts',(-0.645024363515573,3.15775596017347,301.919814873786));
#4244=CARTESIAN_POINT('Ctrl Pts',(-0.68113880854343,3.15016337865994,301.922034037524));
#4245=CARTESIAN_POINT('Ctrl Pts',(-0.899161140598576,3.10040213866061,301.935326554268));
#4246=CARTESIAN_POINT('Ctrl Pts',(-1.07727074207155,3.04310484274677,301.94575668842));
#4247=CARTESIAN_POINT('Ctrl Pts',(-1.37294364717353,2.91874929396772,301.963759474257));
#4248=CARTESIAN_POINT('Ctrl Pts',(-1.49309270256789,2.85915080832196,301.971286435153));
#4249=CARTESIAN_POINT('Ctrl Pts',(-1.66348919025692,2.76095102586271,301.98261563099));
#4250=CARTESIAN_POINT('Ctrl Pts',(-1.71687264610595,2.72807524303073,301.986264769632));
#4251=CARTESIAN_POINT('Ctrl Pts',(-1.81382218260612,2.66439654580075,301.993110807778));
#4252=CARTESIAN_POINT('Ctrl Pts',(-1.85764772834944,2.63402815181,301.996292638502));
#4253=CARTESIAN_POINT('Ctrl Pts',(-1.93002503518077,2.58117022136455,302.001709139965));
#4254=CARTESIAN_POINT('Ctrl Pts',(-1.95898685052975,2.55925901464714,302.003921956551));
#4255=CARTESIAN_POINT('Ctrl Pts',(-2.01670583488942,2.51403758709401,302.008428313554));
#4256=CARTESIAN_POINT('Ctrl Pts',(-2.04544393430232,2.49071201613595,302.010722245879));
#4257=CARTESIAN_POINT('Ctrl Pts',(-2.11751906205271,2.43012276927658,302.01660820448));
#4258=CARTESIAN_POINT('Ctrl Pts',(-2.16027679763536,2.39219296059984,302.020226390257));
#4259=CARTESIAN_POINT('Ctrl Pts',(-2.35814107897976,2.20703784112354,302.037591905868));
#4260=CARTESIAN_POINT('Ctrl Pts',(-2.49932970715633,2.04576922141202,302.051915804817));
#4261=CARTESIAN_POINT('Ctrl Pts',(-2.72046649699764,1.73581633850882,302.077593112331));
#4262=CARTESIAN_POINT('Ctrl Pts',(-2.80673861025839,1.59255253214516,302.088856554702));
#4263=CARTESIAN_POINT('Ctrl Pts',(-2.89677624054073,1.41278622824015,302.101824726863));
#4264=CARTESIAN_POINT('Ctrl Pts',(-2.91154542266173,1.38209296957009,302.103999723996));
#4265=CARTESIAN_POINT('Ctrl Pts',(-2.9346238901664,1.33211881524392,302.107471533848));
#4266=CARTESIAN_POINT('Ctrl Pts',(-2.94323596838296,1.31298134997625,302.108784846463));
#4267=CARTESIAN_POINT('Ctrl Pts',(-2.96038181534689,1.27386380531314,302.111434481281));
#4268=CARTESIAN_POINT('Ctrl Pts',(-2.96890164483975,1.25387901008216,302.11277002841));
#4269=CARTESIAN_POINT('Ctrl Pts',(-2.99164140203908,1.199007275036,302.116391653468));
#4270=CARTESIAN_POINT('Ctrl Pts',(-3.0054531616125,1.16395373070989,302.118655586132));
#4271=CARTESIAN_POINT('Ctrl Pts',(-3.09930031094924,0.912956643547117,302.134569412469));
#4272=CARTESIAN_POINT('Ctrl Pts',(-3.15660877708911,0.689200884248465,302.147244531102));
#4273=CARTESIAN_POINT('Ctrl Pts',(-3.21161788323767,0.30878948818202,302.168896293925));
#4274=CARTESIAN_POINT('Ctrl Pts',(-3.22270289320938,0.154983159663994,302.17767059053));
#4275=CARTESIAN_POINT('Ctrl Pts',(-3.22276580278082,-0.0513356018517207,
302.189859200967));
#4276=CARTESIAN_POINT('Ctrl Pts',(-3.22150775251864,-0.10364416094275,302.192984082902));
#4277=CARTESIAN_POINT('Ctrl Pts',(-3.21722876997443,-0.191997104707538,
302.198332964639));
#4278=CARTESIAN_POINT('Ctrl Pts',(-3.21487331077823,-0.228064203310865,
302.200536404917));
#4279=CARTESIAN_POINT('Ctrl Pts',(-3.20922094147811,-0.296811200111426,
302.204777712067));
#4280=CARTESIAN_POINT('Ctrl Pts',(-3.20603003806182,-0.329495387503727,
302.206812053817));
#4281=CARTESIAN_POINT('Ctrl Pts',(-3.19624613172568,-0.416016527269546,
302.212247272874));
#4282=CARTESIAN_POINT('Ctrl Pts',(-3.1887927799652,-0.469743691384225,302.215673997404));
#4283=CARTESIAN_POINT('Ctrl Pts',(-3.14096708145004,-0.760395850071991,
302.234503004226));
#4284=CARTESIAN_POINT('Ctrl Pts',(-3.07554765739168,-0.992395016090034,
302.250670481751));
#4285=CARTESIAN_POINT('Ctrl Pts',(-2.94661817863001,-1.30916417782987,302.273723134994));
#4286=CARTESIAN_POINT('Ctrl Pts',(-2.90381901916496,-1.40153719398589,302.280561153221));
#4287=CARTESIAN_POINT('Ctrl Pts',(-2.83654024802534,-1.53037824036094,302.290143628212));
#4288=CARTESIAN_POINT('Ctrl Pts',(-2.81557790831675,-1.56861069688823,302.292992726357));
#4289=CARTESIAN_POINT('Ctrl Pts',(-2.77655110855963,-1.63648564947723,302.298046411385));
#4290=CARTESIAN_POINT('Ctrl Pts',(-2.75877143845277,-1.66628380263649,302.300263477205));
#4291=CARTESIAN_POINT('Ctrl Pts',(-2.72940399550728,-1.71374359994853,302.303785084261));
#4292=CARTESIAN_POINT('Ctrl Pts',(-2.71811818269049,-1.73158797427979,302.305106947595));
#4293=CARTESIAN_POINT('Ctrl Pts',(-2.69495043300568,-1.76743454884903,302.307755823025));
#4294=CARTESIAN_POINT('Ctrl Pts',(-2.68306157868412,-1.78543085730189,302.309082335909));
#4295=CARTESIAN_POINT('Ctrl Pts',(-2.65033935025029,-1.83389782787387,302.312649665728));
#4296=CARTESIAN_POINT('Ctrl Pts',(-2.62916114697263,-1.86413299773039,302.314869443073));
#4297=CARTESIAN_POINT('Ctrl Pts',(-2.4978730182205,-2.04487727651015,302.328147853828));
#4298=CARTESIAN_POINT('Ctrl Pts',(-2.375377668476,-2.18597546425527,302.338565095895));
#4299=CARTESIAN_POINT('Ctrl Pts',(-2.09779979157631,-2.45464190113278,302.360246544473));
#4300=CARTESIAN_POINT('Ctrl Pts',(-1.94165263881097,-2.57992354549356,302.371484735465));
#4301=CARTESIAN_POINT('Ctrl Pts',(-1.73147175570793,-2.71860863098421,302.386364689123));
#4302=CARTESIAN_POINT('Ctrl Pts',(-1.68733624352936,-2.74621981728922,302.38947452305));
#4303=CARTESIAN_POINT('Ctrl Pts',(-1.61149581100998,-2.79114705121563,302.394805595799));
#4304=CARTESIAN_POINT('Ctrl Pts',(-1.58013257040606,-2.80902145052584,302.39700661366));
#4305=CARTESIAN_POINT('Ctrl Pts',(-1.5243051829562,-2.83960752620019,302.400921189997));
#4306=CARTESIAN_POINT('Ctrl Pts',(-1.49996563704107,-2.85253925179863,302.402626772245));
#4307=CARTESIAN_POINT('Ctrl Pts',(-1.47546400229876,-2.86515680904563,302.404343180173));
#4308=CARTESIAN_POINT('Origin',(0.,0.,294.689226550727));
#4309=CARTESIAN_POINT('',(-1.47546400670695,-2.86515680677555,303.903774856397));
#4310=CARTESIAN_POINT('',(-1.47546383039573,-2.86515689757018,303.659226720281));
#4311=CARTESIAN_POINT('',(-1.47546400239267,-2.86515680899727,294.689226550727));
#4312=CARTESIAN_POINT('',(3.22274978263189,0.00118365792144974,303.057982460212));
#4313=CARTESIAN_POINT('Ctrl Pts',(-1.47546400670695,-2.86515680677555,303.903774856397));
#4314=CARTESIAN_POINT('Ctrl Pts',(-1.64703992383269,-2.7768007037036,303.890776726147));
#4315=CARTESIAN_POINT('Ctrl Pts',(-1.81035156217509,-2.67320167904195,303.877671639076));
#4316=CARTESIAN_POINT('Ctrl Pts',(-1.99185243055068,-2.53375739307966,303.862879504612));
#4317=CARTESIAN_POINT('Ctrl Pts',(-2.01991429026229,-2.51144363538858,303.860586313955));
#4318=CARTESIAN_POINT('Ctrl Pts',(-2.06407442531159,-2.47510999874109,303.856975206977));
#4319=CARTESIAN_POINT('Ctrl Pts',(-2.08041512192467,-2.46139101297975,303.855638448391));
#4320=CARTESIAN_POINT('Ctrl Pts',(-2.11278122990651,-2.43366512642933,303.852991729229));
#4321=CARTESIAN_POINT('Ctrl Pts',(-2.12880653300698,-2.419659743581,303.851681786262));
#4322=CARTESIAN_POINT('Ctrl Pts',(-2.17125751362461,-2.38181129630646,303.848209470128));
#4323=CARTESIAN_POINT('Ctrl Pts',(-2.19742966188655,-2.35768686517194,303.846066283176));
#4324=CARTESIAN_POINT('Ctrl Pts',(-2.25586995852725,-2.30200021413352,303.841260646555));
#4325=CARTESIAN_POINT('Ctrl Pts',(-2.28788587475091,-2.2701834376632,303.838613456726));
#4326=CARTESIAN_POINT('Ctrl Pts',(-2.394351410733,-2.15983929400474,303.829716810863));
#4327=CARTESIAN_POINT('Ctrl Pts',(-2.46551386365164,-2.07823684474175,303.82360670651));
#4328=CARTESIAN_POINT('Ctrl Pts',(-2.67292206994574,-1.81471718757523,303.804756006067));
#4329=CARTESIAN_POINT('Ctrl Pts',(-2.79412955370635,-1.62189440690968,303.792115830217));
#4330=CARTESIAN_POINT('Ctrl Pts',(-2.91863148260553,-1.36778190217344,303.775452500689));
#4331=CARTESIAN_POINT('Ctrl Pts',(-2.94189616456491,-1.31699790374123,303.772125479833));
#4332=CARTESIAN_POINT('Ctrl Pts',(-2.97825921934005,-1.23184406484862,303.766536927087));
#4333=CARTESIAN_POINT('Ctrl Pts',(-2.99211032432934,-1.19780775416496,303.764300677367));
#4334=CARTESIAN_POINT('Ctrl Pts',(-3.01854345939051,-1.12953223310251,303.759806225724));
#4335=CARTESIAN_POINT('Ctrl Pts',(-3.031132167772,-1.09530146220508,303.757548643026));
#4336=CARTESIAN_POINT('Ctrl Pts',(-3.06102519918106,-1.00955205574303,303.751879697221));
#4337=CARTESIAN_POINT('Ctrl Pts',(-3.07761189331703,-0.957797002403391,
303.748445944007));
#4338=CARTESIAN_POINT('Ctrl Pts',(-3.1109669885766,-0.843886120364744,303.740857926401));
#4339=CARTESIAN_POINT('Ctrl Pts',(-3.12719730379387,-0.781598080957308,
303.736689150671));
#4340=CARTESIAN_POINT('Ctrl Pts',(-3.17299354537236,-0.58146253220149,303.723239028106));
#4341=CARTESIAN_POINT('Ctrl Pts',(-3.19538468486823,-0.442151313892892,
303.713785752114));
#4342=CARTESIAN_POINT('Ctrl Pts',(-3.22480127742499,-0.129443062851917,
303.692611258972));
#4343=CARTESIAN_POINT('Ctrl Pts',(-3.22709965554132,0.0439846905240419,
303.680894853082));
#4344=CARTESIAN_POINT('Ctrl Pts',(-3.21286988157641,0.255064913389759,303.66718715784));
#4345=CARTESIAN_POINT('Ctrl Pts',(-3.20960387595817,0.293315932480469,303.664726205883));
#4346=CARTESIAN_POINT('Ctrl Pts',(-3.20340692144339,0.353241186111654,303.660916246447));
#4347=CARTESIAN_POINT('Ctrl Pts',(-3.20093759968591,0.374958378955537,303.659544907881));
#4348=CARTESIAN_POINT('Ctrl Pts',(-3.19568167654034,0.417337718593409,303.656889435075));
#4349=CARTESIAN_POINT('Ctrl Pts',(-3.19291518748996,0.438000896554211,303.655604436301));
#4350=CARTESIAN_POINT('Ctrl Pts',(-3.18519130253673,0.491722767386906,303.652285738227));
#4351=CARTESIAN_POINT('Ctrl Pts',(-3.17991957596055,0.524734789674906,303.650268269316));
#4352=CARTESIAN_POINT('Ctrl Pts',(-3.16695752725866,0.59851321161376,303.64579666514));
#4353=CARTESIAN_POINT('Ctrl Pts',(-3.15899176796981,0.639225583198342,303.643354778871));
#4354=CARTESIAN_POINT('Ctrl Pts',(-3.13054138666105,0.771071636469618,303.635497985669));
#4355=CARTESIAN_POINT('Ctrl Pts',(-3.10688019852166,0.86147442372401,303.630190172295));
#4356=CARTESIAN_POINT('Ctrl Pts',(-3.00286087530714,1.198384530277,303.610306744584));
#4357=CARTESIAN_POINT('Ctrl Pts',(-2.89680882073736,1.43589304542686,303.595991172968));
#4358=CARTESIAN_POINT('Ctrl Pts',(-2.73695103401422,1.70231349000082,303.577622383332));
#4359=CARTESIAN_POINT('Ctrl Pts',(-2.70938750585779,1.7458496759023,303.574543090492));
#4360=CARTESIAN_POINT('Ctrl Pts',(-2.66102150797335,1.81833745998218,303.569271389652));
#4361=CARTESIAN_POINT('Ctrl Pts',(-2.64076035919025,1.84763934655529,303.567098898376));
#4362=CARTESIAN_POINT('Ctrl Pts',(-2.59829348237041,1.90692959583001,303.56261376611));
#4363=CARTESIAN_POINT('Ctrl Pts',(-2.57604440063986,1.93688011177592,303.560299704713));
#4364=CARTESIAN_POINT('Ctrl Pts',(-2.51735578698527,2.01308318969035,303.554282414172));
#4365=CARTESIAN_POINT('Ctrl Pts',(-2.48016092469924,2.05873387465501,303.550550570188));
#4366=CARTESIAN_POINT('Ctrl Pts',(-2.39485184176819,2.15776810772177,303.542162267115));
#4367=CARTESIAN_POINT('Ctrl Pts',(-2.3461611812047,2.21061193287783,303.537485353967));
#4368=CARTESIAN_POINT('Ctrl Pts',(-2.17165758768544,2.3877361262764,303.521107428813));
#4369=CARTESIAN_POINT('Ctrl Pts',(-2.03741862728109,2.50325740162402,303.509137394115));
#4370=CARTESIAN_POINT('Ctrl Pts',(-1.78757615510471,2.68479498467136,303.488350790574));
#4371=CARTESIAN_POINT('Ctrl Pts',(-1.6760762210895,2.75578070158462,303.479528749445));
#4372=CARTESIAN_POINT('Ctrl Pts',(-1.53227791175949,2.83536317818561,303.468949705946));
#4373=CARTESIAN_POINT('Ctrl Pts',(-1.50379480462413,2.85057210371432,303.466891539695));
#4374=CARTESIAN_POINT('Ctrl Pts',(-1.45855309369064,2.87386259992281,303.463686244889));
#4375=CARTESIAN_POINT('Ctrl Pts',(-1.44194552686641,2.88223116956595,303.462522962458));
#4376=CARTESIAN_POINT('Ctrl Pts',(-1.40600598591886,2.89995273510034,303.46003565169));
#4377=CARTESIAN_POINT('Ctrl Pts',(-1.38665101833263,2.90925724392156,303.45871461091));
#4378=CARTESIAN_POINT('Ctrl Pts',(-1.33413101749682,2.93386193774287,303.455175808777));
#4379=CARTESIAN_POINT('Ctrl Pts',(-1.30079562116827,2.94879338742762,303.45297854448));
#4380=CARTESIAN_POINT('Ctrl Pts',(-1.22424109596349,2.98153241039079,303.448027349343));
#4381=CARTESIAN_POINT('Ctrl Pts',(-1.18087347722927,2.99897315751643,303.445290097142));
#4382=CARTESIAN_POINT('Ctrl Pts',(-1.02931135345218,3.05612763916361,303.435906749962));
#4383=CARTESIAN_POINT('Ctrl Pts',(-0.919373295761669,3.09097939198203,303.42941634474));
#4384=CARTESIAN_POINT('Ctrl Pts',(-0.600456048695917,3.17355376570913,303.410914511226));
#4385=CARTESIAN_POINT('Ctrl Pts',(-0.388296340070686,3.20643223628765,303.39895783596));
#4386=CARTESIAN_POINT('Ctrl Pts',(-0.117435068217946,3.2211157927311,303.383001384459));
#4387=CARTESIAN_POINT('Ctrl Pts',(-0.0603496933341818,3.2226906901211,303.379603082123));
#4388=CARTESIAN_POINT('Ctrl Pts',(0.0337208880234273,3.22278570215275,303.373928736213));
#4389=CARTESIAN_POINT('Ctrl Pts',(0.0706934557232164,3.22218668669088,303.371679700065));
#4390=CARTESIAN_POINT('Ctrl Pts',(0.143900989283213,3.21974004080657,303.367185367169));
#4391=CARTESIAN_POINT('Ctrl Pts',(0.180131311604691,3.21791640168691,303.364941134504));
#4392=CARTESIAN_POINT('Ctrl Pts',(0.269440640683299,3.21190810299397,303.359356537013));
#4393=CARTESIAN_POINT('Ctrl Pts',(0.322459902247589,3.2070190217009,303.355995225971));
#4394=CARTESIAN_POINT('Ctrl Pts',(0.437488160306886,3.19353068860341,303.348598520563));
#4395=CARTESIAN_POINT('Ctrl Pts',(0.499416054034859,3.18443353923819,303.344549887132));
#4396=CARTESIAN_POINT('Ctrl Pts',(0.69264604506215,3.15027321482627,303.331712896561));
#4397=CARTESIAN_POINT('Ctrl Pts',(0.822670594343443,3.11884399761831,303.322769933577));
#4398=CARTESIAN_POINT('Ctrl Pts',(1.12941154473084,3.02417928932736,303.301142764094));
#4399=CARTESIAN_POINT('Ctrl Pts',(1.30331426887408,2.95340679198056,303.28843040933));
#4400=CARTESIAN_POINT('Ctrl Pts',(1.50288317194297,2.85110816200811,303.273921908207));
#4401=CARTESIAN_POINT('Ctrl Pts',(1.53538791899156,2.83373601075532,303.271562408484));
#4402=CARTESIAN_POINT('Ctrl Pts',(1.58641073614623,2.80533110137519,303.267872594399));
#4403=CARTESIAN_POINT('Ctrl Pts',(1.60512752506377,2.79466407661601,303.26652208425));
#4404=CARTESIAN_POINT('Ctrl Pts',(1.64195544782887,2.77318313942054,303.263872912534));
#4405=CARTESIAN_POINT('Ctrl Pts',(1.6600700306086,2.76237759095298,303.262573908045));
#4406=CARTESIAN_POINT('Ctrl Pts',(1.70766798804779,2.73334756135107,303.259167879495));
#4407=CARTESIAN_POINT('Ctrl Pts',(1.73696657071128,2.71482341897815,303.257078753184));
#4408=CARTESIAN_POINT('Ctrl Pts',(1.80238803500374,2.67196766076223,303.252417487722));
#4409=CARTESIAN_POINT('Ctrl Pts',(1.83832841668652,2.64736902820155,303.249859265508));
#4410=CARTESIAN_POINT('Ctrl Pts',(1.95641024736844,2.56298573211447,303.241424360068));
#4411=CARTESIAN_POINT('Ctrl Pts',(2.03622569171254,2.50004482069593,303.235672250693));
#4412=CARTESIAN_POINT('Ctrl Pts',(2.29468205859889,2.27562862774268,303.216408777792));
#4413=CARTESIAN_POINT('Ctrl Pts',(2.45815980934174,2.09797339487428,303.20305713722));
#4414=CARTESIAN_POINT('Ctrl Pts',(2.63232887658665,1.86007948301842,303.185669195881));
#4415=CARTESIAN_POINT('Ctrl Pts',(2.66321540827956,1.81558095090272,303.182438896499));
#4416=CARTESIAN_POINT('Ctrl Pts',(2.71098388656152,1.74291707379026,303.177185895728));
#4417=CARTESIAN_POINT('Ctrl Pts',(2.72858289538505,1.71523433448492,303.175189635818));
#4418=CARTESIAN_POINT('Ctrl Pts',(2.76465978944355,1.65652573818348,303.170963599017));
#4419=CARTESIAN_POINT('Ctrl Pts',(2.78304481718737,1.62544844677601,303.168730866642));
#4420=CARTESIAN_POINT('Ctrl Pts',(2.82675793581253,1.54864113352191,303.163220054273));
#4421=CARTESIAN_POINT('Ctrl Pts',(2.85150228505659,1.50259242887546,303.159922273455));
#4422=CARTESIAN_POINT('Ctrl Pts',(2.90269117303861,1.40150895993529,303.152692392094));
#4423=CARTESIAN_POINT('Ctrl Pts',(2.9287133903155,1.34628397887262,303.148748116728));
#4424=CARTESIAN_POINT('Ctrl Pts',(3.00423160533578,1.17345054718622,303.136424941579));
#4425=CARTESIAN_POINT('Ctrl Pts',(3.04832181703954,1.05362384471593,303.127905208829));
#4426=CARTESIAN_POINT('Ctrl Pts',(3.10129921026084,0.87816069803812,303.115567252037));
#4427=CARTESIAN_POINT('Ctrl Pts',(3.11602001096471,0.824404178271397,303.111806264146));
#4428=CARTESIAN_POINT('Ctrl Pts',(3.12974010974781,0.768665868225409,303.107937075732));
#4429=CARTESIAN_POINT('Ctrl Pts',(3.13013943786739,0.767038115772963,303.107824108745));
#4430=CARTESIAN_POINT('Ctrl Pts',(3.14965191724887,0.687231810421434,303.102286831792));
#4431=CARTESIAN_POINT('Ctrl Pts',(3.16583175498072,0.608362453887039,303.096876159802));
#4432=CARTESIAN_POINT('Ctrl Pts',(3.19152114932299,0.453971854317972,303.086484531808));
#4433=CARTESIAN_POINT('Ctrl Pts',(3.20134314521489,0.37855183052115,303.081499602661));
#4434=CARTESIAN_POINT('Ctrl Pts',(3.2111672238192,0.274472358776477,303.074803934069));
#4435=CARTESIAN_POINT('Ctrl Pts',(3.21346928796665,0.246059504636998,303.072994818867));
#4436=CARTESIAN_POINT('Ctrl Pts',(3.21672359690848,0.197975935185697,303.069968997583));
#4437=CARTESIAN_POINT('Ctrl Pts',(3.21787304032332,0.178320897428194,303.068742345663));
#4438=CARTESIAN_POINT('Ctrl Pts',(3.21976697660709,0.139896146143514,303.066365017933));
#4439=CARTESIAN_POINT('Ctrl Pts',(3.22052761665186,0.12112895931221,303.065213288147));
#4440=CARTESIAN_POINT('Ctrl Pts',(3.22219541480293,0.068643499314685,303.062015894739));
#4441=CARTESIAN_POINT('Ctrl Pts',(3.22273739359673,0.0349153296029804,303.059988401622));
#4442=CARTESIAN_POINT('Ctrl Pts',(3.22274978263189,0.00118365792144974,
303.057982460212));
#4443=CARTESIAN_POINT('Ctrl Pts',(3.22274978135357,0.0011871333156251,303.057982666885));
#4444=CARTESIAN_POINT('Ctrl Pts',(3.22282215967534,-0.195300672711181,303.046298000788));
#4445=CARTESIAN_POINT('Ctrl Pts',(3.20492489689649,-0.39141482917079,303.035355889149));
#4446=CARTESIAN_POINT('Ctrl Pts',(3.14597524532254,-0.710940044934372,303.017115073304));
#4447=CARTESIAN_POINT('Ctrl Pts',(3.11516470245604,-0.835668823371542,303.009889828884));
#4448=CARTESIAN_POINT('Ctrl Pts',(3.05878981325368,-1.01669727728896,302.998954718108));
#4449=CARTESIAN_POINT('Ctrl Pts',(3.03891752920731,-1.07463860111911,302.995385414962));
#4450=CARTESIAN_POINT('Ctrl Pts',(2.99900211799949,-1.18103751210788,302.988672598943));
#4451=CARTESIAN_POINT('Ctrl Pts',(2.97940391253876,-1.22964026481056,302.985543098519));
#4452=CARTESIAN_POINT('Ctrl Pts',(2.94430605617543,-1.31090988304529,302.9801904342));
#4453=CARTESIAN_POINT('Ctrl Pts',(2.92942547827781,-1.34383372481131,302.977987961534));
#4454=CARTESIAN_POINT('Ctrl Pts',(2.89999399256367,-1.40613901762976,302.973751381266));
#4455=CARTESIAN_POINT('Ctrl Pts',(2.88554201781415,-1.43556234051875,302.971720838681));
#4456=CARTESIAN_POINT('Ctrl Pts',(2.84609044767663,-1.51287976787604,302.966303088094));
#4457=CARTESIAN_POINT('Ctrl Pts',(2.82033191745928,-1.56037282525552,302.962890297893));
#4458=CARTESIAN_POINT('Ctrl Pts',(2.67283357490284,-1.81673320848036,302.943987694369));
#4459=CARTESIAN_POINT('Ctrl Pts',(2.52909632679752,-2.01201272774872,302.927721540704));
#4460=CARTESIAN_POINT('Ctrl Pts',(2.29623140226047,-2.26355059429498,302.904617794217));
#4461=CARTESIAN_POINT('Ctrl Pts',(2.22408910706801,-2.33447412570847,302.897823960675));
#4462=CARTESIAN_POINT('Ctrl Pts',(2.11636223527207,-2.43084644778694,302.88829597584));
#4463=CARTESIAN_POINT('Ctrl Pts',(2.08341213465356,-2.45914574121506,302.885458206472));
#4464=CARTESIAN_POINT('Ctrl Pts',(2.02320811965574,-2.50877319129619,302.880422682717));
#4465=CARTESIAN_POINT('Ctrl Pts',(1.99616380274306,-2.53034470235584,302.878212562607));
#4466=CARTESIAN_POINT('Ctrl Pts',(1.95208924029284,-2.56435360433839,302.874700045792));
#4467=CARTESIAN_POINT('Ctrl Pts',(1.93527568376051,-2.57706614370546,302.873380452149));
#4468=CARTESIAN_POINT('Ctrl Pts',(1.90101496141205,-2.6024458570146,302.870734430252));
#4469=CARTESIAN_POINT('Ctrl Pts',(1.88356309473785,-2.61510467298162,302.869408525631));
#4470=CARTESIAN_POINT('Ctrl Pts',(1.83587386969106,-2.64897123900244,302.865840548283));
#4471=CARTESIAN_POINT('Ctrl Pts',(1.80539602270693,-2.66983650200855,302.863619557783));
#4472=CARTESIAN_POINT('Ctrl Pts',(1.61973046894774,-2.79231019303226,302.8503994142));
#4473=CARTESIAN_POINT('Ctrl Pts',(1.45635000823409,-2.88089961067451,302.840034391468));
#4474=CARTESIAN_POINT('Ctrl Pts',(1.16269295093685,-3.00872373829066,302.822059298298));
#4475=CARTESIAN_POINT('Ctrl Pts',(1.03589936654935,-3.05469857648612,302.814492063085));
#4476=CARTESIAN_POINT('Ctrl Pts',(0.846290048557142,-3.11028317168793,302.803111409237));
#4477=CARTESIAN_POINT('Ctrl Pts',(0.785472195981641,-3.12619593767203,302.799452838664));
#4478=CARTESIAN_POINT('Ctrl Pts',(0.672187800579716,-3.15232193788623,302.792591819323));
#4479=CARTESIAN_POINT('Ctrl Pts',(0.619857332590626,-3.16302805046279,302.789404582625));
#4480=CARTESIAN_POINT('Ctrl Pts',(0.53154926625777,-3.17881911603224,302.783983312327));
#4481=CARTESIAN_POINT('Ctrl Pts',(0.495707161687191,-3.1846051311663,302.781771284133));
#4482=CARTESIAN_POINT('Ctrl Pts',(0.423215331552128,-3.1950541156918,302.777270376426));
#4483=CARTESIAN_POINT('Ctrl Pts',(0.386567977348554,-3.19969483559144,302.774981169959));
#4484=CARTESIAN_POINT('Ctrl Pts',(0.293287485980368,-3.20988122754678,302.769116063972));
#4485=CARTESIAN_POINT('Ctrl Pts',(0.236574230213031,-3.21455860695353,302.765514324017));
#4486=CARTESIAN_POINT('Ctrl Pts',(-0.036566787012202,-3.22981856003294,
302.747986798995));
#4487=CARTESIAN_POINT('Ctrl Pts',(-0.253541444060071,-3.22005530422065,
302.733465946025));
#4488=CARTESIAN_POINT('Ctrl Pts',(-0.630607992416144,-3.1647287216089,302.707764851886));
#4489=CARTESIAN_POINT('Ctrl Pts',(-0.791301066712531,-3.12842222518099,
302.696674878214));
#4490=CARTESIAN_POINT('Ctrl Pts',(-0.981135095872506,-3.06996016606138,
302.683861922834));
#4491=CARTESIAN_POINT('Ctrl Pts',(-1.0135804364278,-3.05940131524089,302.681683042893));
#4492=CARTESIAN_POINT('Ctrl Pts',(-1.06569997050893,-3.04151958504009,302.678207510384));
#4493=CARTESIAN_POINT('Ctrl Pts',(-1.08548039255301,-3.03451646987384,302.67689427096));
#4494=CARTESIAN_POINT('Ctrl Pts',(-1.12555158747701,-3.01988757260093,302.674247707146));
#4495=CARTESIAN_POINT('Ctrl Pts',(-1.14583647819923,-3.01224935116519,302.672915110734));
#4496=CARTESIAN_POINT('Ctrl Pts',(-1.20099843193554,-2.9908403885497,302.669306930165));
#4497=CARTESIAN_POINT('Ctrl Pts',(-1.23571569256085,-2.97666431713816,302.667053245252));
#4498=CARTESIAN_POINT('Ctrl Pts',(-1.33974785891755,-2.93205100418127,302.66032965188));
#4499=CARTESIAN_POINT('Ctrl Pts',(-1.40821778573291,-2.8997864605469,302.65594455659));
#4500=CARTESIAN_POINT('Ctrl Pts',(-1.47546411936631,-2.86515674875958,302.651619072379));
#4501=CARTESIAN_POINT('Ctrl Pts',(-1.47546400229876,-2.86515680904563,302.404343180173));
#4502=CARTESIAN_POINT('Ctrl Pts',(-1.47073118624233,-2.86759405775003,302.404674727153));
#4503=CARTESIAN_POINT('Ctrl Pts',(-1.46599232228165,-2.87001958418981,302.405006677517));
#4504=CARTESIAN_POINT('Ctrl Pts',(-1.41265079463178,-2.89715517325867,302.408742979947));
#4505=CARTESIAN_POINT('Ctrl Pts',(-1.36343707625227,-2.92063848148305,302.412188592157));
#4506=CARTESIAN_POINT('Ctrl Pts',(-1.09617202871527,-3.03994200400015,302.43090242102));
#4507=CARTESIAN_POINT('Ctrl Pts',(-0.86862901796382,-3.11260185013267,302.446919076186));
#4508=CARTESIAN_POINT('Ctrl Pts',(-0.534459251722771,-3.17978471014962,
302.469896306618));
#4509=CARTESIAN_POINT('Ctrl Pts',(-0.432797805361918,-3.19520976496153,
302.476804626933));
#4510=CARTESIAN_POINT('Ctrl Pts',(-0.286956688052462,-3.21024854093123,
302.486472526695));
#4511=CARTESIAN_POINT('Ctrl Pts',(-0.243254973779329,-3.2138555034111,302.489338426503));
#4512=CARTESIAN_POINT('Ctrl Pts',(-0.164716151259587,-3.21872647520065,
302.494418409729));
#4513=CARTESIAN_POINT('Ctrl Pts',(-0.129906570391553,-3.22031924493887,
302.496645152468));
#4514=CARTESIAN_POINT('Ctrl Pts',(-0.0739435201431905,-3.22197096638263,
302.500178229253));
#4515=CARTESIAN_POINT('Ctrl Pts',(-0.0528041435150932,-3.22238674650866,
302.501502075628));
#4516=CARTESIAN_POINT('Ctrl Pts',(-0.0101291085400843,-3.22280602078181,
302.50415089681));
#4517=CARTESIAN_POINT('Ctrl Pts',(0.0114054518002629,-3.22280176589306,
302.505475433915));
#4518=CARTESIAN_POINT('Ctrl Pts',(0.0696809240949528,-3.22220611352631,
302.509030908092));
#4519=CARTESIAN_POINT('Ctrl Pts',(0.10641542374083,-3.22120221022146,302.511241044003));
#4520=CARTESIAN_POINT('Ctrl Pts',(0.332366381158546,-3.21115753204423,302.524687294124));
#4521=CARTESIAN_POINT('Ctrl Pts',(0.520517618063955,-3.18607552435117,302.535259539811));
#4522=CARTESIAN_POINT('Ctrl Pts',(0.834655131401481,-3.11560879406432,302.553329585848));
#4523=CARTESIAN_POINT('Ctrl Pts',(0.962002931064495,-3.07867100874392,302.560775190834));
#4524=CARTESIAN_POINT('Ctrl Pts',(1.14536707144118,-3.01299415473027,302.571998593587));
#4525=CARTESIAN_POINT('Ctrl Pts',(1.20339906949475,-2.99028920927167,302.575626733216));
#4526=CARTESIAN_POINT('Ctrl Pts',(1.30958088626837,-2.94515408251542,302.582437933963));
#4527=CARTESIAN_POINT('Ctrl Pts',(1.35790484512252,-2.92318809327359,302.585606211378));
#4528=CARTESIAN_POINT('Ctrl Pts',(1.4383038180321,-2.88421834563816,302.591006589947));
#4529=CARTESIAN_POINT('Ctrl Pts',(1.47067467203613,-2.86784748275387,302.593217147003));
#4530=CARTESIAN_POINT('Ctrl Pts',(1.53554975619119,-2.83365105415766,302.597724720318));
#4531=CARTESIAN_POINT('Ctrl Pts',(1.56803644807082,-2.81580412477582,302.600022227241));
#4532=CARTESIAN_POINT('Ctrl Pts',(1.65006177195242,-2.76888289886511,302.605930131731));
#4533=CARTESIAN_POINT('Ctrl Pts',(1.69914248232862,-2.73903824824186,302.609567085062));
#4534=CARTESIAN_POINT('Ctrl Pts',(1.9235588087959,-2.59422325144197,302.626686718665));
#4535=CARTESIAN_POINT('Ctrl Pts',(2.08818379566014,-2.46364320786856,302.640719492988));
#4536=CARTESIAN_POINT('Ctrl Pts',(2.32374576687523,-2.23611808026006,302.662804903421));
#4537=CARTESIAN_POINT('Ctrl Pts',(2.40399355096707,-2.14961288248822,302.670760825514));
#4538=CARTESIAN_POINT('Ctrl Pts',(2.50956150784151,-2.02248830197332,302.6816874032));
#4539=CARTESIAN_POINT('Ctrl Pts',(2.53899591464482,-1.98541130565433,302.684789793274));
#4540=CARTESIAN_POINT('Ctrl Pts',(2.58988827498364,-1.91832110299869,302.690237741653));
#4541=CARTESIAN_POINT('Ctrl Pts',(2.61166768733984,-1.88856275588037,302.692598608586));
#4542=CARTESIAN_POINT('Ctrl Pts',(2.64536526867472,-1.84082182232138,302.696290891586));
#4543=CARTESIAN_POINT('Ctrl Pts',(2.65762130397304,-1.8230829525313,302.69764252059));
#4544=CARTESIAN_POINT('Ctrl Pts',(2.68010611390223,-1.78983071272968,302.700136685735));
#4545=CARTESIAN_POINT('Ctrl Pts',(2.69038036243288,-1.77434954194624,302.701282176299));
#4546=CARTESIAN_POINT('Ctrl Pts',(2.71804315638984,-1.73187468052494,302.704384854147));
#4547=CARTESIAN_POINT('Ctrl Pts',(2.73516361706921,-1.70470779669856,302.706325639925));
#4548=CARTESIAN_POINT('Ctrl Pts',(2.81653828565511,-1.57119886370915,302.715675644608));
#4549=CARTESIAN_POINT('Ctrl Pts',(2.87501821711156,-1.46144792323411,302.722791891237));
#4550=CARTESIAN_POINT('Ctrl Pts',(2.98285306220959,-1.22739909297677,302.737362824025));
#4551=CARTESIAN_POINT('Ctrl Pts',(3.0311078479289,-1.10286296536373,302.744791730176));
#4552=CARTESIAN_POINT('Ctrl Pts',(3.11528559822034,-0.837869584490296,302.760498505911));
#4553=CARTESIAN_POINT('Ctrl Pts',(3.14973659919007,-0.697268268618499,302.768779802692));
#4554=CARTESIAN_POINT('Ctrl Pts',(3.18307834439978,-0.506495929627978,302.780257793227));
#4555=CARTESIAN_POINT('Ctrl Pts',(3.19042151169116,-0.457969510802434,302.783196887772));
#4556=CARTESIAN_POINT('Ctrl Pts',(3.20117748000664,-0.373964071771196,302.788328118672));
#4557=CARTESIAN_POINT('Ctrl Pts',(3.20511512978323,-0.338560533890505,302.790503780196));
#4558=CARTESIAN_POINT('Ctrl Pts',(3.21205961313571,-0.265049717864161,302.795051718627));
#4559=CARTESIAN_POINT('Ctrl Pts',(3.21497689582935,-0.226939802926653,302.797426387712));
#4560=CARTESIAN_POINT('Ctrl Pts',(3.22093863610593,-0.125343420396632,302.803805373462));
#4561=CARTESIAN_POINT('Ctrl Pts',(3.22278385710846,-0.0618061141021424,
302.807845217358));
#4562=CARTESIAN_POINT('Ctrl Pts',(3.22261075162948,0.25864997648741,302.828484081738));
#4563=CARTESIAN_POINT('Ctrl Pts',(3.19175126853861,0.514593732784742,302.845924818716));
#4564=CARTESIAN_POINT('Ctrl Pts',(3.10330441094823,0.876996154347947,302.870975938121));
#4565=CARTESIAN_POINT('Ctrl Pts',(3.0696650687625,0.988322617464399,302.878704430591));
#4566=CARTESIAN_POINT('Ctrl Pts',(3.01926688378704,1.12745442980147,302.888223283326));
#4567=CARTESIAN_POINT('Ctrl Pts',(3.00801029837313,1.15715177289447,302.890246489179));
#4568=CARTESIAN_POINT('Ctrl Pts',(2.98882481859061,1.20559432260662,302.893527139406));
#4569=CARTESIAN_POINT('Ctrl Pts',(2.98115425020853,1.22443900955153,302.894798374417));
#4570=CARTESIAN_POINT('Ctrl Pts',(2.96469060871092,1.26381401286018,302.897442417982));
#4571=CARTESIAN_POINT('Ctrl Pts',(2.95586173361889,1.28432773945447,302.898813185237));
#4572=CARTESIAN_POINT('Ctrl Pts',(2.9303515257064,1.34194342556025,302.902648568309));
#4573=CARTESIAN_POINT('Ctrl Pts',(2.91317944215478,1.37882489511807,302.90508646073));
#4574=CARTESIAN_POINT('Ctrl Pts',(2.8715341634513,1.46401522768814,302.910699278798));
#4575=CARTESIAN_POINT('Ctrl Pts',(2.84653229818124,1.51205273629969,302.913850255582));
#4576=CARTESIAN_POINT('Ctrl Pts',(2.74617891591497,1.69354724448225,302.925784793454));
#4577=CARTESIAN_POINT('Ctrl Pts',(2.66255291101688,1.82220122979056,302.934315251613));
#4578=CARTESIAN_POINT('Ctrl Pts',(2.47339160539816,2.07222983097413,302.951938808824));
#4579=CARTESIAN_POINT('Ctrl Pts',(2.36730662596435,2.19263660830288,302.961018786929));
#4580=CARTESIAN_POINT('Ctrl Pts',(2.21147956025781,2.34495208503251,302.973830815243));
#4581=CARTESIAN_POINT('Ctrl Pts',(2.16917432184813,2.38414015872624,302.97726110704));
#4582=CARTESIAN_POINT('Ctrl Pts',(2.09795386841559,2.44664750544897,302.982975639701));
#4583=CARTESIAN_POINT('Ctrl Pts',(2.06964550137172,2.4706399525505,302.985232113078));
#4584=CARTESIAN_POINT('Ctrl Pts',(2.01288184600661,2.5170891350449,302.989731576848));
#4585=CARTESIAN_POINT('Ctrl Pts',(1.98444941896548,2.53956519435411,302.991973330519));
#4586=CARTESIAN_POINT('Ctrl Pts',(1.9136024405337,2.59365400375975,302.997533276792));
#4587=CARTESIAN_POINT('Ctrl Pts',(1.87077824453454,2.62471020010579,303.000871942451));
#4588=CARTESIAN_POINT('Ctrl Pts',(1.6663142656951,2.7654414522541,303.016719160653));
#4589=CARTESIAN_POINT('Ctrl Pts',(1.4957052382413,2.86131356461579,303.029711100135));
#4590=CARTESIAN_POINT('Ctrl Pts',(1.14465155149746,3.01856916110233,303.055622931002));
#4591=CARTESIAN_POINT('Ctrl Pts',(0.965309747860758,3.08061244993346,303.068476524314));
#4592=CARTESIAN_POINT('Ctrl Pts',(0.745898209242017,3.13545909671536,303.083106399989));
#4593=CARTESIAN_POINT('Ctrl Pts',(0.710096840959386,3.14376058577432,303.08545896521));
#4594=CARTESIAN_POINT('Ctrl Pts',(0.653102158562313,3.15595292155799,303.089141401667));
#4595=CARTESIAN_POINT('Ctrl Pts',(0.631999340417796,3.16024653579823,303.090491314491));
#4596=CARTESIAN_POINT('Ctrl Pts',(0.590095776164454,3.16833576443631,303.093142913525));
#4597=CARTESIAN_POINT('Ctrl Pts',(0.569297704291204,3.1721388227948,303.094444889453));
#4598=CARTESIAN_POINT('Ctrl Pts',(0.514131956612587,3.18166618002054,303.097864601036));
#4599=CARTESIAN_POINT('Ctrl Pts',(0.479705293320635,3.18703849991994,303.099964204537));
#4600=CARTESIAN_POINT('Ctrl Pts',(0.401777805202147,3.19790775962321,303.104652681084));
#4601=CARTESIAN_POINT('Ctrl Pts',(0.35823786897593,3.20307749029294,303.107227401044));
#4602=CARTESIAN_POINT('Ctrl Pts',(0.212352988394196,3.21738708739144,303.115744010839));
#4603=CARTESIAN_POINT('Ctrl Pts',(0.109674848605747,3.22252186847198,303.121558811112));
#4604=CARTESIAN_POINT('Ctrl Pts',(-0.231264026754964,3.22325415432443,303.140741777871));
#4605=CARTESIAN_POINT('Ctrl Pts',(-0.468751265253419,3.19736035322521,303.153962012385));
#4606=CARTESIAN_POINT('Ctrl Pts',(-0.754422865009971,3.13367767926094,303.171217721134));
#4607=CARTESIAN_POINT('Ctrl Pts',(-0.80732165319049,3.12046805758551,303.174468417191));
#4608=CARTESIAN_POINT('Ctrl Pts',(-0.891549973011353,3.09714991238025,303.179746952336));
#4609=CARTESIAN_POINT('Ctrl Pts',(-0.923105044203148,3.08789181975811,303.18174788583));
#4610=CARTESIAN_POINT('Ctrl Pts',(-0.988991136293969,3.06746103702494,303.185977874329));
#4611=CARTESIAN_POINT('Ctrl Pts',(-1.02328698497413,3.05619113650004,303.188209798947));
#4612=CARTESIAN_POINT('Ctrl Pts',(-1.10656455137934,3.02726656109742,303.193706300597));
#4613=CARTESIAN_POINT('Ctrl Pts',(-1.1553203326412,3.00899690495565,303.196990283259));
#4614=CARTESIAN_POINT('Ctrl Pts',(-1.3914325832045,2.91393691341763,303.213228028599));
#4615=CARTESIAN_POINT('Ctrl Pts',(-1.57168400618003,2.82079774467714,303.226708918506));
#4616=CARTESIAN_POINT('Ctrl Pts',(-1.89647521547669,2.6121291731121,303.252723428358));
#4617=CARTESIAN_POINT('Ctrl Pts',(-2.04221078422254,2.49984419389492,303.26517140535));
#4618=CARTESIAN_POINT('Ctrl Pts',(-2.20487479584916,2.35074753952906,303.279448856976));
#4619=CARTESIAN_POINT('Ctrl Pts',(-2.23172214386057,2.3252749076172,303.281818430088));
#4620=CARTESIAN_POINT('Ctrl Pts',(-2.2735276733419,2.28421878838031,303.28552103702));
#4621=CARTESIAN_POINT('Ctrl Pts',(-2.28877745225841,2.26893838386441,303.286874464034));
#4622=CARTESIAN_POINT('Ctrl Pts',(-2.31862457417345,2.23842415523771,303.289526868143));
#4623=CARTESIAN_POINT('Ctrl Pts',(-2.33322802772809,2.22319806325703,303.290826225489));
#4624=CARTESIAN_POINT('Ctrl Pts',(-2.37139441016025,2.18261408264355,303.294229903876));
#4625=CARTESIAN_POINT('Ctrl Pts',(-2.39470084180177,2.15701733309623,303.296316402392));
#4626=CARTESIAN_POINT('Ctrl Pts',(-2.44632778321765,2.09844859421542,303.300970002786));
#4627=CARTESIAN_POINT('Ctrl Pts',(-2.4744031209738,2.06526890475891,303.303523269194));
#4628=CARTESIAN_POINT('Ctrl Pts',(-2.5655817152442,1.95298378535035,303.311930437607));
#4629=CARTESIAN_POINT('Ctrl Pts',(-2.62563267707783,1.87147281167556,303.317660676606));
#4630=CARTESIAN_POINT('Ctrl Pts',(-2.81569372539025,1.58629080278081,303.336949523175));
#4631=CARTESIAN_POINT('Ctrl Pts',(-2.92660846150452,1.37091327505838,303.350344338374));
#4632=CARTESIAN_POINT('Ctrl Pts',(-3.03163722981131,1.09463097391607,303.367777357582));
#4633=CARTESIAN_POINT('Ctrl Pts',(-3.04957501095754,1.0436153599602,303.371002559855));
#4634=CARTESIAN_POINT('Ctrl Pts',(-3.07632202155272,0.960956303316408,303.376251042861));
#4635=CARTESIAN_POINT('Ctrl Pts',(-3.08594609560629,0.929586344529534,303.378248024955));
#4636=CARTESIAN_POINT('Ctrl Pts',(-3.10516834700565,0.863339612859892,303.382478743651));
#4637=CARTESIAN_POINT('Ctrl Pts',(-3.11466162469535,0.82843741352914,303.384715489576));
#4638=CARTESIAN_POINT('Ctrl Pts',(-3.13648284051657,0.742526935923535,303.390243232737));
#4639=CARTESIAN_POINT('Ctrl Pts',(-3.14815586945379,0.691364575490198,303.393554159819));
#4640=CARTESIAN_POINT('Ctrl Pts',(-3.19952951293693,0.437798800746816,303.410065432128));
#4641=CARTESIAN_POINT('Ctrl Pts',(-3.22097927321176,0.232219546214998,303.423813819264));
#4642=CARTESIAN_POINT('Ctrl Pts',(-3.22408194811515,-0.15186893454161,303.449704216477));
#4643=CARTESIAN_POINT('Ctrl Pts',(-3.21078554084386,-0.329595601194456,
303.46175161882));
#4644=CARTESIAN_POINT('Ctrl Pts',(-3.1769947099357,-0.542433264828102,303.475703594132));
#4645=CARTESIAN_POINT('Ctrl Pts',(-3.17045463772679,-0.579436707839862,
303.478110739751));
#4646=CARTESIAN_POINT('Ctrl Pts',(-3.15911805593236,-0.637621918302519,
303.481857872273));
#4647=CARTESIAN_POINT('Ctrl Pts',(-3.15475226010913,-0.658883025528071,
303.483219036873));
#4648=CARTESIAN_POINT('Ctrl Pts',(-3.1457400139075,-0.700627125412806,303.485873522869));
#4649=CARTESIAN_POINT('Ctrl Pts',(-3.14110752252592,-0.721111762154714,
303.487167420926));
#4650=CARTESIAN_POINT('Ctrl Pts',(-3.12841983970934,-0.774772414640497,
303.49053735861));
#4651=CARTESIAN_POINT('Ctrl Pts',(-3.12003692285038,-0.807869293173191,
303.492596223553));
#4652=CARTESIAN_POINT('Ctrl Pts',(-3.06806031743263,-1.00018675913143,303.504477624436));
#4653=CARTESIAN_POINT('Ctrl Pts',(-3.01280598652666,-1.15601884162136,303.513782491706));
#4654=CARTESIAN_POINT('Ctrl Pts',(-2.85829448932416,-1.50428718918191,303.535182829026));
#4655=CARTESIAN_POINT('Ctrl Pts',(-2.75114249946419,-1.69231587262444,303.547229867387));
#4656=CARTESIAN_POINT('Ctrl Pts',(-2.59296814802093,-1.91464909170332,303.563282079689));
#4657=CARTESIAN_POINT('Ctrl Pts',(-2.55870943262058,-1.96019652785262,303.56667392179));
#4658=CARTESIAN_POINT('Ctrl Pts',(-2.50025749546235,-2.03376439634545,303.572342092101));
#4659=CARTESIAN_POINT('Ctrl Pts',(-2.47675637025817,-2.06231977976725,303.574591597428));
#4660=CARTESIAN_POINT('Ctrl Pts',(-2.42919792277136,-2.11812076322277,303.579090524794));
#4661=CARTESIAN_POINT('Ctrl Pts',(-2.40516074822255,-2.14537635916619,303.581338943004));
#4662=CARTESIAN_POINT('Ctrl Pts',(-2.34464074878341,-2.21170395879428,303.586941404644));
#4663=CARTESIAN_POINT('Ctrl Pts',(-2.30763797041343,-2.25028467235845,303.590316642938));
#4664=CARTESIAN_POINT('Ctrl Pts',(-2.22503573099356,-2.33222870419721,303.597748933199));
#4665=CARTESIAN_POINT('Ctrl Pts',(-2.17909173714081,-2.37521222929232,303.601819436283));
#4666=CARTESIAN_POINT('Ctrl Pts',(-2.03076261350509,-2.506055998836,303.614762178431));
#4667=CARTESIAN_POINT('Ctrl Pts',(-1.9241084167384,-2.58884435303294,303.623791871355));
#4668=CARTESIAN_POINT('Ctrl Pts',(-1.70435177593856,-2.73832775044546,303.641700132459));
#4669=CARTESIAN_POINT('Ctrl Pts',(-1.59176505135959,-2.80526550205583,303.650554729941));
#4670=CARTESIAN_POINT('Ctrl Pts',(-1.47546383039573,-2.86515689757018,303.659226720281));
#4671=CARTESIAN_POINT('Origin',(0.,0.,294.689226550727));
#4672=CARTESIAN_POINT('',(-1.47546404664855,-2.86515678620691,305.155887179421));
#4673=CARTESIAN_POINT('',(-1.47546400239266,-2.86515680899727,304.907226776837));
#4674=CARTESIAN_POINT('',(-1.47546400239267,-2.86515680899727,294.689226550727));
#4675=CARTESIAN_POINT('Ctrl Pts',(-1.47546404664855,-2.86515678620691,305.155887179421));
#4676=CARTESIAN_POINT('Ctrl Pts',(-1.49316374364744,-2.85604200872452,305.154720915483));
#4677=CARTESIAN_POINT('Ctrl Pts',(-1.5107819037227,-2.8467617142584,305.153549744734));
#4678=CARTESIAN_POINT('Ctrl Pts',(-1.57449668637968,-2.81244184882883,305.149274969888));
#4679=CARTESIAN_POINT('Ctrl Pts',(-1.62006092853701,-2.78644416795494,305.146142369751));
#4680=CARTESIAN_POINT('Ctrl Pts',(-1.69591126983339,-2.74067666114335,305.140785984996));
#4681=CARTESIAN_POINT('Ctrl Pts',(-1.72653663150235,-2.72148758859424,305.138582960081));
#4682=CARTESIAN_POINT('Ctrl Pts',(-1.78430624294524,-2.68392302332692,305.134346362532));
#4683=CARTESIAN_POINT('Ctrl Pts',(-1.81150563956517,-2.66564040297228,305.132316372654));
#4684=CARTESIAN_POINT('Ctrl Pts',(-1.88274691770939,-2.61616020606856,305.126902653766));
#4685=CARTESIAN_POINT('Ctrl Pts',(-1.9262905287871,-2.5842667103688,305.123493416488));
#4686=CARTESIAN_POINT('Ctrl Pts',(-2.16072392027659,-2.40333834129658,305.104568210095));
#4687=CARTESIAN_POINT('Ctrl Pts',(-2.33512218897093,-2.23426314333312,305.0882725942));
#4688=CARTESIAN_POINT('Ctrl Pts',(-2.55302653029998,-1.96935467844235,305.065153258795));
#4689=CARTESIAN_POINT('Ctrl Pts',(-2.61344362514271,-1.88844289890856,305.058372279037));
#4690=CARTESIAN_POINT('Ctrl Pts',(-2.69426177257947,-1.7688847075046,305.048859923564));
#4691=CARTESIAN_POINT('Ctrl Pts',(-2.71783006194092,-1.7324548181515,305.046025233074));
#4692=CARTESIAN_POINT('Ctrl Pts',(-2.75884091741652,-1.66616594427883,305.040994526723));
#4693=CARTESIAN_POINT('Ctrl Pts',(-2.77655207708742,-1.63648126893127,305.038786177897));
#4694=CARTESIAN_POINT('Ctrl Pts',(-2.80428713421642,-1.58824911455079,305.035275759083));
#4695=CARTESIAN_POINT('Ctrl Pts',(-2.81461224766097,-1.56987883212058,305.03395652675));
#4696=CARTESIAN_POINT('Ctrl Pts',(-2.83513743179889,-1.53250719314596,305.031310546652));
#4697=CARTESIAN_POINT('Ctrl Pts',(-2.84532839740595,-1.51350220531433,305.029984333198));
#4698=CARTESIAN_POINT('Ctrl Pts',(-2.87246667299078,-1.46164935258219,305.026414336919));
#4699=CARTESIAN_POINT('Ctrl Pts',(-2.88904139628843,-1.42860900326692,305.024191679205));
#4700=CARTESIAN_POINT('Ctrl Pts',(-2.98495192823632,-1.22891966931751,305.011025125885));
#4701=CARTESIAN_POINT('Ctrl Pts',(-3.05042850666079,-1.05597453408301,305.000708662556));
#4702=CARTESIAN_POINT('Ctrl Pts',(-3.15575627952288,-0.684151336469236,
304.97901935552));
#4703=CARTESIAN_POINT('Ctrl Pts',(-3.19239832983542,-0.485224844343754,
304.967670947032));
#4704=CARTESIAN_POINT('Ctrl Pts',(-3.21477415564542,-0.232466607196427,
304.95267509705));
#4705=CARTESIAN_POINT('Ctrl Pts',(-3.21810202310599,-0.180644738732072,
304.949572888072));
#4706=CARTESIAN_POINT('Ctrl Pts',(-3.22161674848267,-0.0927493535312843,
304.944252604883));
#4707=CARTESIAN_POINT('Ctrl Pts',(-3.22245257605405,-0.0567111239931853,
304.942054610426));
#4708=CARTESIAN_POINT('Ctrl Pts',(-3.22289447443074,0.01219399505377,304.937817071601));
#4709=CARTESIAN_POINT('Ctrl Pts',(-3.22260257160361,0.045055828071636,304.935780931109));
#4710=CARTESIAN_POINT('Ctrl Pts',(-3.2204898432914,0.132427263979405,304.930324533378));
#4711=CARTESIAN_POINT('Ctrl Pts',(-3.21778783173552,0.186902957202241,304.926877996607));
#4712=CARTESIAN_POINT('Ctrl Pts',(-3.19589392540861,0.478514993889393,304.908179726014));
#4713=CARTESIAN_POINT('Ctrl Pts',(-3.15187114207106,0.713014122122916,304.892181500064));
#4714=CARTESIAN_POINT('Ctrl Pts',(-3.05243256585465,1.03892441235154,304.869211572598));
#4715=CARTESIAN_POINT('Ctrl Pts',(-3.01770073760766,1.13586647693936,304.862292821137));
#4716=CARTESIAN_POINT('Ctrl Pts',(-2.96163150045991,1.27152700900264,304.852613029857));
#4717=CARTESIAN_POINT('Ctrl Pts',(-2.94404801618804,1.31172546736024,304.84974538177));
#4718=CARTESIAN_POINT('Ctrl Pts',(-2.91103300150666,1.38319158874947,304.844663102886));
#4719=CARTESIAN_POINT('Ctrl Pts',(-2.89590459572361,1.41459142629879,304.842435785033));
#4720=CARTESIAN_POINT('Ctrl Pts',(-2.87079041445604,1.46462500581743,304.838902923953));
#4721=CARTESIAN_POINT('Ctrl Pts',(-2.86112584457242,1.4834159839704,304.837579844716));
#4722=CARTESIAN_POINT('Ctrl Pts',(-2.84125709313927,1.52113044032037,304.834933983126));
#4723=CARTESIAN_POINT('Ctrl Pts',(-2.8310470278782,1.54004950296656,304.83361161504));
#4724=CARTESIAN_POINT('Ctrl Pts',(-2.80292824391191,1.5909282924235,304.830064880375));
#4725=CARTESIAN_POINT('Ctrl Pts',(-2.78466216429091,1.62268803322388,304.827861168992));
#4726=CARTESIAN_POINT('Ctrl Pts',(-2.66798007151201,1.81779113570213,304.814344452143));
#4727=CARTESIAN_POINT('Ctrl Pts',(-2.55575840042095,1.97245970458257,304.803705390371));
#4728=CARTESIAN_POINT('Ctrl Pts',(-2.30290373160404,2.26285437228965,304.782092698221));
#4729=CARTESIAN_POINT('Ctrl Pts',(-2.16232317970976,2.39754544054297,304.771150909799));
#4730=CARTESIAN_POINT('Ctrl Pts',(-1.96919146406032,2.55170392376792,304.756559507566));
#4731=CARTESIAN_POINT('Ctrl Pts',(-1.92710459841531,2.58363606944183,304.753405726438));
#4732=CARTESIAN_POINT('Ctrl Pts',(-1.85488340600002,2.63568506461599,304.748024222789));
#4733=CARTESIAN_POINT('Ctrl Pts',(-1.82515951082132,2.65635479702645,304.745817740689));
#4734=CARTESIAN_POINT('Ctrl Pts',(-1.76430688753924,2.69716759318922,304.741313721397));
#4735=CARTESIAN_POINT('Ctrl Pts',(-1.73316623046602,2.7172829182394,304.739015612972));
#4736=CARTESIAN_POINT('Ctrl Pts',(-1.6527645920479,2.767273997165,304.733096008376));
#4737=CARTESIAN_POINT('Ctrl Pts',(-1.60303853246442,2.79637318172693,304.729447689896));
#4738=CARTESIAN_POINT('Ctrl Pts',(-1.37208669979633,2.92333897249458,304.712551974839));
#4739=CARTESIAN_POINT('Ctrl Pts',(-1.18254061012296,3.0050138347113,304.698777106955));
#4740=CARTESIAN_POINT('Ctrl Pts',(-0.872085231278484,3.10484082869179,304.676786954529));
#4741=CARTESIAN_POINT('Ctrl Pts',(-0.75566763338803,3.13520936077227,304.668670935858));
#4742=CARTESIAN_POINT('Ctrl Pts',(-0.590946363926448,3.16846758784061,304.657555009922));
#4743=CARTESIAN_POINT('Ctrl Pts',(-0.543863667735707,3.17688797338381,304.654419401677));
#4744=CARTESIAN_POINT('Ctrl Pts',(-0.459906743603022,3.18998168726016,304.648920527274));
#4745=CARTESIAN_POINT('Ctrl Pts',(-0.423106517064948,3.19507097248516,304.646541555823));
#4746=CARTESIAN_POINT('Ctrl Pts',(-0.364777809486342,3.20211202001002,304.6428286337));
#4747=CARTESIAN_POINT('Ctrl Pts',(-0.343304608254074,3.20448533248845,304.641474084295));
#4748=CARTESIAN_POINT('Ctrl Pts',(-0.30087268998837,3.20874366510589,304.638823880528));
#4749=CARTESIAN_POINT('Ctrl Pts',(-0.279916362748223,3.21063968000682,304.637527780647));
#4750=CARTESIAN_POINT('Ctrl Pts',(-0.224645954322845,3.21509496779267,304.634139632036));
#4751=CARTESIAN_POINT('Ctrl Pts',(-0.190305820533833,3.2173102683198,304.63206513669));
#4752=CARTESIAN_POINT('Ctrl Pts',(0.0548844912920111,3.22918790628011,304.61742992429));
#4753=CARTESIAN_POINT('Ctrl Pts',(0.26622330660073,3.21866637499759,304.605722496545));
#4754=CARTESIAN_POINT('Ctrl Pts',(0.641281462629434,3.16277212319044,304.58442108968));
#4755=CARTESIAN_POINT('Ctrl Pts',(0.805320483147841,3.12503139196682,304.574917732615));
#4756=CARTESIAN_POINT('Ctrl Pts',(1.02061127270893,3.05741519424331,304.561649176959));
#4757=CARTESIAN_POINT('Ctrl Pts',(1.0750871668516,3.0386875512137,304.558222437333));
#4758=CARTESIAN_POINT('Ctrl Pts',(1.16374926039165,3.00552479814698,304.552513792548));
#4759=CARTESIAN_POINT('Ctrl Pts',(1.19824099991222,2.99194083941493,304.550259593611));
#4760=CARTESIAN_POINT('Ctrl Pts',(1.26555320246021,2.96408048557714,304.545790559052));
#4761=CARTESIAN_POINT('Ctrl Pts',(1.29838538264591,2.9498463130635,304.543577383026));
#4762=CARTESIAN_POINT('Ctrl Pts',(1.37876990448207,2.91339415002311,304.538072902596));
#4763=CARTESIAN_POINT('Ctrl Pts',(1.42602812312218,2.8905562111598,304.534761254982));
#4764=CARTESIAN_POINT('Ctrl Pts',(1.69746549132284,2.75110503862986,304.515285323597));
#4765=CARTESIAN_POINT('Ctrl Pts',(1.90783311337018,2.60961688034789,304.498255595423));
#4766=CARTESIAN_POINT('Ctrl Pts',(2.17246739918002,2.38238481161996,304.474757591511));
#4767=CARTESIAN_POINT('Ctrl Pts',(2.24261382289641,2.31647511840793,304.468302749959));
#4768=CARTESIAN_POINT('Ctrl Pts',(2.33913904247339,2.21727916905321,304.45918885652));
#4769=CARTESIAN_POINT('Ctrl Pts',(2.36797323943586,2.18645864898127,304.456434207468));
#4770=CARTESIAN_POINT('Ctrl Pts',(2.41883679209558,2.12990435704553,304.451529156999));
#4771=CARTESIAN_POINT('Ctrl Pts',(2.44108150076025,2.10437290197028,304.449367263377));
#4772=CARTESIAN_POINT('Ctrl Pts',(2.4764199913087,2.06249841101479,304.445911814753));
#4773=CARTESIAN_POINT('Ctrl Pts',(2.48976373756538,2.04637051317138,304.444602002801));
#4774=CARTESIAN_POINT('Ctrl Pts',(2.51664464129725,2.01322873372171,304.441954944974));
#4775=CARTESIAN_POINT('Ctrl Pts',(2.53016853505408,1.99620575860901,304.440618541443));
#4776=CARTESIAN_POINT('Ctrl Pts',(2.56674258417041,1.94919988934794,304.436987430651));
#4777=CARTESIAN_POINT('Ctrl Pts',(2.58943956409225,1.91894520991004,304.434715094447));
#4778=CARTESIAN_POINT('Ctrl Pts',(2.74106846761206,1.70923556457782,304.419349333768));
#4779=CARTESIAN_POINT('Ctrl Pts',(2.85179303507868,1.51731383440288,304.407151278844));
#4780=CARTESIAN_POINT('Ctrl Pts',(2.99629973149484,1.19414882465384,304.387233964455));
#4781=CARTESIAN_POINT('Ctrl Pts',(3.04301688720277,1.06950826454934,304.379692200525));
#4782=CARTESIAN_POINT('Ctrl Pts',(3.10168370022079,0.877641101643442,304.367984795442));
#4783=CARTESIAN_POINT('Ctrl Pts',(3.11942458627493,0.812333067949683,304.363984693996));
#4784=CARTESIAN_POINT('Ctrl Pts',(3.14412273901258,0.708610093902216,304.357580362979));
#4785=CARTESIAN_POINT('Ctrl Pts',(3.15246067521097,0.670542732267735,304.355219305203));
#4786=CARTESIAN_POINT('Ctrl Pts',(3.16703610866834,0.597701700178213,304.350676781026));
#4787=CARTESIAN_POINT('Ctrl Pts',(3.17339612318629,0.562958193332626,304.34849950599));
#4788=CARTESIAN_POINT('Ctrl Pts',(3.18676820314149,0.482460500210809,304.343427616852));
#4789=CARTESIAN_POINT('Ctrl Pts',(3.19336797874565,0.436646675162563,304.340520730888));
#4790=CARTESIAN_POINT('Ctrl Pts',(3.21244026604963,0.280489707996374,304.330538429997));
#4791=CARTESIAN_POINT('Ctrl Pts',(3.22019535865749,0.169659834785927,304.323325110275));
#4792=CARTESIAN_POINT('Ctrl Pts',(3.22258796276283,0.0382331994695072,304.314634770256));
#4793=CARTESIAN_POINT('Ctrl Pts',(3.22276557763011,0.0178035706015105,304.313280132694));
#4794=CARTESIAN_POINT('Ctrl Pts',(3.22263452749977,-0.143019708263997,304.30258870143));
#4795=CARTESIAN_POINT('Ctrl Pts',(3.21334617871903,-0.283251278918383,304.293091111162));
#4796=CARTESIAN_POINT('Ctrl Pts',(3.1771700584407,-0.556864925498543,304.274507747648));
#4797=CARTESIAN_POINT('Ctrl Pts',(3.15092484735525,-0.690063204470942,304.265438596113));
#4798=CARTESIAN_POINT('Ctrl Pts',(3.10812548675147,-0.852477754685679,304.254626826507));
#4799=CARTESIAN_POINT('Ctrl Pts',(3.09941869919516,-0.883609796852329,304.252566198727));
#4800=CARTESIAN_POINT('Ctrl Pts',(3.08496537620158,-0.932444224090226,304.249358064959));
#4801=CARTESIAN_POINT('Ctrl Pts',(3.07953161619108,-0.95023611530413,304.24819435824));
#4802=CARTESIAN_POINT('Ctrl Pts',(3.06749714181303,-0.988453101375741,304.245707242786));
#4803=CARTESIAN_POINT('Ctrl Pts',(3.06084579618803,-1.00886139792871,304.244386806468));
#4804=CARTESIAN_POINT('Ctrl Pts',(3.04234348808644,-1.06376399127046,304.240851631853));
#4805=CARTESIAN_POINT('Ctrl Pts',(3.03010973815845,-1.09812701934421,304.238657318256));
#4806=CARTESIAN_POINT('Ctrl Pts',(3.00090570111415,-1.17595004655124,304.233714096154));
#4807=CARTESIAN_POINT('Ctrl Pts',(2.98356963825308,-1.21926459158721,304.230981786844));
#4808=CARTESIAN_POINT('Ctrl Pts',(2.92031969953649,-1.36785953148776,304.22162569127));
#4809=CARTESIAN_POINT('Ctrl Pts',(2.86972204020532,-1.47105577370453,304.215156659433));
#4810=CARTESIAN_POINT('Ctrl Pts',(2.70895547560288,-1.75893337525869,304.19663767952));
#4811=CARTESIAN_POINT('Ctrl Pts',(2.58570208625026,-1.93556758003063,304.184644633481));
#4812=CARTESIAN_POINT('Ctrl Pts',(2.40864786459496,-2.14191206046656,304.168650110785));
#4813=CARTESIAN_POINT('Ctrl Pts',(2.37035897601791,-2.18420913855521,304.165254878936));
#4814=CARTESIAN_POINT('Ctrl Pts',(2.30544259355637,-2.25220303101069,304.159584230742));
#4815=CARTESIAN_POINT('Ctrl Pts',(2.27945850618761,-2.2784979245228,304.157335746622));
#4816=CARTESIAN_POINT('Ctrl Pts',(2.22708560205572,-2.32970464415134,304.152841436414));
#4817=CARTESIAN_POINT('Ctrl Pts',(2.20071690282306,-2.3546292604049,304.150596655651));
#4818=CARTESIAN_POINT('Ctrl Pts',(2.13459837089485,-2.41504586990703,304.145008587956));
#4819=CARTESIAN_POINT('Ctrl Pts',(2.09437951490615,-2.45000626084511,304.141644296002));
#4820=CARTESIAN_POINT('Ctrl Pts',(2.00502239007602,-2.52387172156856,304.134239742906));
#4821=CARTESIAN_POINT('Ctrl Pts',(1.95557921687508,-2.56237241380963,304.130186191668));
#4822=CARTESIAN_POINT('Ctrl Pts',(1.79701268065843,-2.6785823674287,304.117324573989));
#4823=CARTESIAN_POINT('Ctrl Pts',(1.68415472921881,-2.75094089642649,304.108361225245));
#4824=CARTESIAN_POINT('Ctrl Pts',(1.40383780298862,-2.90693647913362,304.086747954692));
#4825=CARTESIAN_POINT('Ctrl Pts',(1.23293943748096,-2.98343921469679,304.074071436949));
#4826=CARTESIAN_POINT('Ctrl Pts',(1.02152704943106,-3.05678913817226,304.059593968997));
#4827=CARTESIAN_POINT('Ctrl Pts',(0.986482440994274,-3.06827801910034,304.05723288439));
#4828=CARTESIAN_POINT('Ctrl Pts',(0.930659950212072,-3.08552327545251,304.053541188323));
#4829=CARTESIAN_POINT('Ctrl Pts',(0.910009220843388,-3.09167674653208,304.052190348411));
#4830=CARTESIAN_POINT('Ctrl Pts',(0.869029013173711,-3.10344176922206,304.049541095819));
#4831=CARTESIAN_POINT('Ctrl Pts',(0.848703248760924,-3.10906176845595,304.048242331822));
#4832=CARTESIAN_POINT('Ctrl Pts',(0.794848170145396,-3.12338498990013,304.044837779364));
#4833=CARTESIAN_POINT('Ctrl Pts',(0.761230189213781,-3.13174810973855,304.042749860165));
#4834=CARTESIAN_POINT('Ctrl Pts',(0.685094696938178,-3.14938978324987,304.038091805848));
#4835=CARTESIAN_POINT('Ctrl Pts',(0.642510528896745,-3.15835262445451,304.035535558507));
#4836=CARTESIAN_POINT('Ctrl Pts',(0.500087224827143,-3.18532896403729,304.027110702863));
#4837=CARTESIAN_POINT('Ctrl Pts',(0.399576880784147,-3.19949189806946,304.021366354643));
#4838=CARTESIAN_POINT('Ctrl Pts',(0.058595382843254,-3.23121744376429,304.002093056539));
#4839=CARTESIAN_POINT('Ctrl Pts',(-0.183095845248976,-3.22655638666897,
303.988725313126));
#4840=CARTESIAN_POINT('Ctrl Pts',(-0.475657243538987,-3.1879141596626,303.971321021085));
#4841=CARTESIAN_POINT('Ctrl Pts',(-0.529121446324816,-3.17947739437225,
303.968093096521));
#4842=CARTESIAN_POINT('Ctrl Pts',(-0.614601548931674,-3.16377275658393,
303.962842894413));
#4843=CARTESIAN_POINT('Ctrl Pts',(-0.646764083781591,-3.15735478195386,
303.960847001965));
#4844=CARTESIAN_POINT('Ctrl Pts',(-0.714125520810718,-3.14284051298556,
303.956620892032));
#4845=CARTESIAN_POINT('Ctrl Pts',(-0.749297309101026,-3.13464114804011,
303.954387705999));
#4846=CARTESIAN_POINT('Ctrl Pts',(-0.835059302489682,-3.11312219198475,
303.948873958713));
#4847=CARTESIAN_POINT('Ctrl Pts',(-0.8854758371264,-3.09915889598517,303.945573647391));
#4848=CARTESIAN_POINT('Ctrl Pts',(-0.993997922765274,-3.06623857812937,
303.938337138034));
#4849=CARTESIAN_POINT('Ctrl Pts',(-1.05194844810441,-3.04684338497022,303.93438872369));
#4850=CARTESIAN_POINT('Ctrl Pts',(-1.22931376673303,-2.98181852584549,303.922045481515));
#4851=CARTESIAN_POINT('Ctrl Pts',(-1.34658497608694,-2.93072658628545,303.913509295283));
#4852=CARTESIAN_POINT('Ctrl Pts',(-1.46549794937883,-2.87027258315036,303.904529264724));
#4853=CARTESIAN_POINT('Ctrl Pts',(-1.47048445786938,-2.86772111497051,303.904152093631));
#4854=CARTESIAN_POINT('Ctrl Pts',(-1.47546400670695,-2.86515680677555,303.903774856397));
#4855=CARTESIAN_POINT('',(3.22274993609481,0.000641795043669797,304.064226550727));
#4856=CARTESIAN_POINT('Ctrl Pts',(-1.47546383039573,-2.86515689757018,303.659226720281));
#4857=CARTESIAN_POINT('Ctrl Pts',(-1.42721028503122,-2.89000592448876,303.662824741659));
#4858=CARTESIAN_POINT('Ctrl Pts',(-1.37831726698886,-2.9136420047774,303.666390446996));
#4859=CARTESIAN_POINT('Ctrl Pts',(-1.29516402843274,-2.95127654637207,303.672295924761));
#4860=CARTESIAN_POINT('Ctrl Pts',(-1.26123696973024,-2.96593403202772,303.674662149003));
#4861=CARTESIAN_POINT('Ctrl Pts',(-1.20711247731433,-2.98822063647225,303.678360785038));
#4862=CARTESIAN_POINT('Ctrl Pts',(-1.18707856567608,-2.99623557903244,303.679713520622));
#4863=CARTESIAN_POINT('Ctrl Pts',(-1.14729213728501,-3.0116911760669,303.682365758989));
#4864=CARTESIAN_POINT('Ctrl Pts',(-1.12754418368385,-3.01914013351242,303.68366562428));
#4865=CARTESIAN_POINT('Ctrl Pts',(-1.07517786037837,-3.03830730683537,303.687072420292));
#4866=CARTESIAN_POINT('Ctrl Pts',(-1.04244021666449,-3.04969462935961,303.689161468369));
#4867=CARTESIAN_POINT('Ctrl Pts',(-0.968182958571903,-3.07418840267462,
303.693821848812));
#4868=CARTESIAN_POINT('Ctrl Pts',(-0.926568233904473,-3.0869862672627,303.696379284248));
#4869=CARTESIAN_POINT('Ctrl Pts',(-0.78712094784443,-3.1267966028928,303.704807641956));
#4870=CARTESIAN_POINT('Ctrl Pts',(-0.688269642230302,-3.15003230638495,
303.71055424094));
#4871=CARTESIAN_POINT('Ctrl Pts',(-0.351661565381582,-3.21254885106674,
303.729822265074));
#4872=CARTESIAN_POINT('Ctrl Pts',(-0.110678289315643,-3.22984162327145,
303.743183048115));
#4873=CARTESIAN_POINT('Ctrl Pts',(0.184091553859675,-3.2179436110702,303.760581510385));
#4874=CARTESIAN_POINT('Ctrl Pts',(0.238140564724718,-3.21439564431528,303.7638117457));
#4875=CARTESIAN_POINT('Ctrl Pts',(0.324763550402713,-3.20651271082044,303.769066157839));
#4876=CARTESIAN_POINT('Ctrl Pts',(0.357406440570748,-3.20303850182447,303.771063916562));
#4877=CARTESIAN_POINT('Ctrl Pts',(0.425878714440959,-3.19469122883886,303.775294468203));
#4878=CARTESIAN_POINT('Ctrl Pts',(0.461690384211446,-3.18971261251982,303.7775302426));
#4879=CARTESIAN_POINT('Ctrl Pts',(0.549171294162807,-3.17604677324705,303.783051710502));
#4880=CARTESIAN_POINT('Ctrl Pts',(0.60072555925839,-3.16670025675986,303.786357228347));
#4881=CARTESIAN_POINT('Ctrl Pts',(0.848976813832634,-3.1154134170457,303.802533857509));
#4882=CARTESIAN_POINT('Ctrl Pts',(1.04165774162688,-3.05638505111758,303.815923010318));
#4883=CARTESIAN_POINT('Ctrl Pts',(1.3979614468484,-2.90960264591401,303.841889773519));
#4884=CARTESIAN_POINT('Ctrl Pts',(1.56204209193491,-2.82491010690087,303.854384928862));
#4885=CARTESIAN_POINT('Ctrl Pts',(1.74928030508781,-2.70693620975969,303.868704018369));
#4886=CARTESIAN_POINT('Ctrl Pts',(1.78022927902662,-2.68668368189604,303.871072134484));
#4887=CARTESIAN_POINT('Ctrl Pts',(1.82867739590745,-2.65377511119295,303.874773013877));
#4888=CARTESIAN_POINT('Ctrl Pts',(1.84640890386678,-2.6414688300028,303.876126140142));
#4889=CARTESIAN_POINT('Ctrl Pts',(1.8812286054825,-2.61678079157132,303.878778472229));
#4890=CARTESIAN_POINT('Ctrl Pts',(1.89832133571935,-2.60440759616097,303.880078050584));
#4891=CARTESIAN_POINT('Ctrl Pts',(1.9431449627143,-2.57128463172423,303.883483084594));
#4892=CARTESIAN_POINT('Ctrl Pts',(1.97066585772615,-2.55025357478157,303.885570691602));
#4893=CARTESIAN_POINT('Ctrl Pts',(2.03196857446068,-2.50182186425688,303.890227239359));
#4894=CARTESIAN_POINT('Ctrl Pts',(2.06554585056862,-2.47417250740885,303.892782317946));
#4895=CARTESIAN_POINT('Ctrl Pts',(2.17544385569904,-2.37987936369645,303.90119869178));
#4896=CARTESIAN_POINT('Ctrl Pts',(2.24918385394179,-2.3103151274614,303.906936037426));
#4897=CARTESIAN_POINT('Ctrl Pts',(2.48700622966486,-2.06376188313354,303.926215813664));
#4898=CARTESIAN_POINT('Ctrl Pts',(2.63444675915894,-1.87189582875144,303.939595825552));
#4899=CARTESIAN_POINT('Ctrl Pts',(2.78705964178637,-1.61905650342582,303.957013812769));
#4900=CARTESIAN_POINT('Ctrl Pts',(2.81384878923454,-1.57203686447769,303.960241207534));
#4901=CARTESIAN_POINT('Ctrl Pts',(2.85496367024925,-1.49545212041664,303.965492273484));
#4902=CARTESIAN_POINT('Ctrl Pts',(2.87004375258331,-1.46630260889329,303.967489594026));
#4903=CARTESIAN_POINT('Ctrl Pts',(2.90079951909344,-1.40455952313598,303.971720239599));
#4904=CARTESIAN_POINT('Ctrl Pts',(2.91637689450022,-1.37192235473578,303.973956561811));
#4905=CARTESIAN_POINT('Ctrl Pts',(2.95318807135371,-1.29133547228735,303.979481567271));
#4906=CARTESIAN_POINT('Ctrl Pts',(2.97380647823742,-1.24311769876269,303.982790134306));
#4907=CARTESIAN_POINT('Ctrl Pts',(3.06981177862278,-1.00252675031615,303.999321334109));
#4908=CARTESIAN_POINT('Ctrl Pts',(3.12774357035196,-0.803741738681032,304.01309427373));
#4909=CARTESIAN_POINT('Ctrl Pts',(3.1952597383578,-0.447935055643875,304.037505795203));
#4910=CARTESIAN_POINT('Ctrl Pts',(3.21316021117902,-0.293149978724763,304.048034960677));
#4911=CARTESIAN_POINT('Ctrl Pts',(3.22177552726619,-0.0916576274483147,
304.061238275884));
#4912=CARTESIAN_POINT('Ctrl Pts',(3.22275646548227,-0.045605109878821,304.064221202948));
#4913=CARTESIAN_POINT('Ctrl Pts',(3.22274996793341,0.000454626470845607,
304.067160013823));
#4914=CARTESIAN_POINT('Ctrl Pts',(3.22274993609481,0.000641795043669797,
304.064226550727));
#4915=CARTESIAN_POINT('Ctrl Pts',(3.22274270887017,0.0369330347259519,304.066479769874));
#4916=CARTESIAN_POINT('Ctrl Pts',(3.2221224892191,0.0732173351279854,304.068732989021));
#4917=CARTESIAN_POINT('Ctrl Pts',(3.22088986744413,0.109480702846282,304.070986208168));
#4918=CARTESIAN_POINT('Ctrl Pts',(3.21750812042288,0.208970699090797,304.077168004802));
#4919=CARTESIAN_POINT('Ctrl Pts',(3.20950662367668,0.308472350520246,304.083349801435));
#4920=CARTESIAN_POINT('Ctrl Pts',(3.19688017044917,0.407522684385618,304.089531598069));
#4921=CARTESIAN_POINT('Ctrl Pts',(3.18427039939254,0.506442152158601,304.095705227263));
#4922=CARTESIAN_POINT('Ctrl Pts',(3.16704787283313,0.604911061938199,304.101878856457));
#4923=CARTESIAN_POINT('Ctrl Pts',(3.14525937378961,0.702467817119461,304.108052485652));
#4924=CARTESIAN_POINT('Ctrl Pts',(3.12349328461099,0.799924233415559,304.114219765157));
#4925=CARTESIAN_POINT('Ctrl Pts',(3.09717065431162,0.89646994031363,304.120387044662));
#4926=CARTESIAN_POINT('Ctrl Pts',(3.06638978326791,0.991650775006099,304.126554324167));
#4927=CARTESIAN_POINT('Ctrl Pts',(3.03563043930724,1.08676504349487,304.132717290489));
#4928=CARTESIAN_POINT('Ctrl Pts',(3.00041918691307,1.18051592712785,304.138880256811));
#4929=CARTESIAN_POINT('Ctrl Pts',(2.96090467180656,1.27246260729898,304.145043223133));
#4930=CARTESIAN_POINT('Ctrl Pts',(2.92140428172553,1.36437641982142,304.151203986415));
#4931=CARTESIAN_POINT('Ctrl Pts',(2.87760385661249,1.45448691337522,304.157364749697));
#4932=CARTESIAN_POINT('Ctrl Pts',(2.82970054147019,1.54237233121686,304.163525512979));
#4933=CARTESIAN_POINT('Ctrl Pts',(2.78180165436517,1.63024962519682,304.169685706779));
#4934=CARTESIAN_POINT('Ctrl Pts',(2.72980083863594,1.7159018725651,304.175845900578));
#4935=CARTESIAN_POINT('Ctrl Pts',(2.67394118373631,1.79893193546028,304.182006094378));
#4936=CARTESIAN_POINT('Ctrl Pts',(2.61807188827152,1.88197632813843,304.188167351338));
#4937=CARTESIAN_POINT('Ctrl Pts',(2.5583426722861,1.96239727833134,304.194328608297));
#4938=CARTESIAN_POINT('Ctrl Pts',(2.49503936435757,2.03982747623572,304.200489865257));
#4939=CARTESIAN_POINT('Ctrl Pts',(2.43166966342175,2.11733888354072,304.206657584192));
#4940=CARTESIAN_POINT('Ctrl Pts',(2.36471866053422,2.19185294013554,304.212825303126));
#4941=CARTESIAN_POINT('Ctrl Pts',(2.2945117214989,2.26303635021715,304.21899302206));
#4942=CARTESIAN_POINT('Ctrl Pts',(2.22426479073441,2.33426030825166,304.225164254291));
#4943=CARTESIAN_POINT('Ctrl Pts',(2.1507585479264,2.40214954778274,304.231335486521));
#4944=CARTESIAN_POINT('Ctrl Pts',(2.07435286996306,2.46640988754425,304.237506718751));
#4945=CARTESIAN_POINT('Ctrl Pts',(1.99782617432783,2.53077200818016,304.243687725493));
#4946=CARTESIAN_POINT('Ctrl Pts',(1.91839121605936,2.59149348779603,304.249868732234));
#4947=CARTESIAN_POINT('Ctrl Pts',(1.8364383890743,2.64832241345993,304.256049738976));
#4948=CARTESIAN_POINT('Ctrl Pts',(1.78626370496904,2.6831152753797,304.259833989893));
#4949=CARTESIAN_POINT('Ctrl Pts',(1.73514577394337,2.71644993843564,304.263618240811));
#4950=CARTESIAN_POINT('Ctrl Pts',(1.68317857908835,2.74827717550435,304.267402491728));
#4951=CARTESIAN_POINT('Ctrl Pts',(1.59828709345055,2.800268849214,304.273584289366));
#4952=CARTESIAN_POINT('Ctrl Pts',(1.5108406362507,2.84841158071823,304.279766087004));
#4953=CARTESIAN_POINT('Ctrl Pts',(1.42122270787832,2.89244595059458,304.285947884642));
#4954=CARTESIAN_POINT('Ctrl Pts',(1.33172318347992,2.93642214188458,304.292121514836));
#4955=CARTESIAN_POINT('Ctrl Pts',(1.24005827613208,2.97630057223439,304.29829514503));
#4956=CARTESIAN_POINT('Ctrl Pts',(1.14663898146327,3.01186596791572,304.304468775224));
#4957=CARTESIAN_POINT('Ctrl Pts',(1.05331577030405,3.04739478391563,304.310636055723));
#4958=CARTESIAN_POINT('Ctrl Pts',(0.958242161946662,3.0786192323306,304.316803336222));
#4959=CARTESIAN_POINT('Ctrl Pts',(0.861851331633066,3.10537112832948,304.322970616721));
#4960=CARTESIAN_POINT('Ctrl Pts',(0.76552791394728,3.13210431491791,304.329133584023));
#4961=CARTESIAN_POINT('Ctrl Pts',(0.667889521836277,3.15437105312516,304.335296551325));
#4962=CARTESIAN_POINT('Ctrl Pts',(0.569385931973019,3.17205252525415,304.341459518628));
#4963=CARTESIAN_POINT('Ctrl Pts',(0.470917553749367,3.18972767686604,304.347620282881));
#4964=CARTESIAN_POINT('Ctrl Pts',(0.371585017917073,3.20282074334881,304.353781047135));
#4965=CARTESIAN_POINT('Ctrl Pts',(0.271848913885091,3.21126388366318,304.359941811389));
#4966=CARTESIAN_POINT('Ctrl Pts',(0.172122029311349,3.21970624350611,304.366102006151));
#4967=CARTESIAN_POINT('Ctrl Pts',(0.071992081938208,3.2234994955584,304.372262200913));
#4968=CARTESIAN_POINT('Ctrl Pts',(-0.0280755712182601,3.22262770496388,
304.378422395675));
#4969=CARTESIAN_POINT('Ctrl Pts',(-0.128160494419948,3.22175576391252,304.384583653586));
#4970=CARTESIAN_POINT('Ctrl Pts',(-0.228182669313109,3.21621718470132,304.390744911497));
#4971=CARTESIAN_POINT('Ctrl Pts',(-0.327678084504641,3.20604813367413,304.396906169408));
#4972=CARTESIAN_POINT('Ctrl Pts',(-0.427277850894759,3.19586841730461,304.403073889272));
#4973=CARTESIAN_POINT('Ctrl Pts',(-0.526349323288656,3.18104857672552,304.409241609135));
#4974=CARTESIAN_POINT('Ctrl Pts',(-0.624435093329909,3.16167651361079,304.415409328999));
#4975=CARTESIAN_POINT('Ctrl Pts',(-0.722576735433399,3.14229341569339,304.421580562147));
#4976=CARTESIAN_POINT('Ctrl Pts',(-0.819731136896843,3.11835303448159,304.427751795295));
#4977=CARTESIAN_POINT('Ctrl Pts',(-0.915454518139479,3.08999362260151,304.433923028444));
#4978=CARTESIAN_POINT('Ctrl Pts',(-1.0113295136034,3.06158929285401,304.440104036076));
#4979=CARTESIAN_POINT('Ctrl Pts',(-1.10576855380984,3.02875209677308,304.446285043709));
#4980=CARTESIAN_POINT('Ctrl Pts',(-1.19834632044172,2.99166904232133,304.452466051342));
#4981=CARTESIAN_POINT('Ctrl Pts',(-1.25502585073748,2.96896542584055,304.456250292657));
#4982=CARTESIAN_POINT('Ctrl Pts',(-1.31100814087214,2.94467124833667,304.460034533973));
#4983=CARTESIAN_POINT('Ctrl Pts',(-1.3662003297416,2.91883782035144,304.463818775288));
#4984=CARTESIAN_POINT('Ctrl Pts',(-1.45636028043439,2.87663727275434,304.470000574151));
#4985=CARTESIAN_POINT('Ctrl Pts',(-1.54471579429518,2.83018393049281,304.476182373015));
#4986=CARTESIAN_POINT('Ctrl Pts',(-1.63083908656621,2.77965491315521,304.482364171878));
#4987=CARTESIAN_POINT('Ctrl Pts',(-1.71684859223722,2.72919265505235,304.488537803312));
#4988=CARTESIAN_POINT('Ctrl Pts',(-1.8006313687029,2.67466564314972,304.494711434746));
#4989=CARTESIAN_POINT('Ctrl Pts',(-1.88178132407699,2.61629826488783,304.50088506618));
#4990=CARTESIAN_POINT('Ctrl Pts',(-1.96284781537727,2.55799091844166,304.507052347932));
#4991=CARTESIAN_POINT('Ctrl Pts',(-2.04128652024617,2.49585131065189,304.513219629684));
#4992=CARTESIAN_POINT('Ctrl Pts',(-2.11671842451974,2.43014828226565,304.519386911436));
#4993=CARTESIAN_POINT('Ctrl Pts',(-2.19209757434309,2.36449120429222,304.525549880006));
#4994=CARTESIAN_POINT('Ctrl Pts',(-2.26447377934179,2.29527594436833,304.531712848575));
#4995=CARTESIAN_POINT('Ctrl Pts',(-2.33350007763975,2.22281239652726,304.537875817145));
#4996=CARTESIAN_POINT('Ctrl Pts',(-2.40250170151066,2.15037475180673,304.544036582674));
#4997=CARTESIAN_POINT('Ctrl Pts',(-2.46815550023419,2.0746914397404,304.550197348203));
#4998=CARTESIAN_POINT('Ctrl Pts',(-2.53015109670326,1.99610946351929,304.556358113733));
#4999=CARTESIAN_POINT('Ctrl Pts',(-2.59214096245767,1.91753475121545,304.562518309777));
#5000=CARTESIAN_POINT('Ctrl Pts',(-2.65047303046909,1.836062247411,304.56867850582));
#5001=CARTESIAN_POINT('Ctrl Pts',(-2.70487761467672,1.75207153167922,304.574838701864));
#5002=CARTESIAN_POINT('Ctrl Pts',(-2.75929158826951,1.66806632045609,304.580999961062));
#5003=CARTESIAN_POINT('Ctrl Pts',(-2.80977649635269,1.58154239721343,304.58716122026));
#5004=CARTESIAN_POINT('Ctrl Pts',(-2.85610687473354,1.49290692362244,304.593322479458));
#5005=CARTESIAN_POINT('Ctrl Pts',(-2.90248584459074,1.40417848881099,304.599490200608));
#5006=CARTESIAN_POINT('Ctrl Pts',(-2.94470138412596,1.31333446610857,304.605657921758));
#5007=CARTESIAN_POINT('Ctrl Pts',(-2.98257484224445,1.22080501019225,304.611825642907));
#5008=CARTESIAN_POINT('Ctrl Pts',(-3.02046987401923,1.12822284721463,304.617996877343));
#5009=CARTESIAN_POINT('Ctrl Pts',(-3.0540177534552,1.03395374656585,304.624168111779));
#5010=CARTESIAN_POINT('Ctrl Pts',(-3.08308935805661,0.938444229956196,304.630339346215));
#5011=CARTESIAN_POINT('Ctrl Pts',(-3.11220700849388,0.84278343805284,304.636520355126));
#5012=CARTESIAN_POINT('Ctrl Pts',(-3.13683411875208,0.745878725935652,304.642701364036));
#5013=CARTESIAN_POINT('Ctrl Pts',(-3.15689242578227,0.648188070345756,304.648882372946));
#5014=CARTESIAN_POINT('Ctrl Pts',(-3.16917281898703,0.588378453249517,304.65266660158));
#5015=CARTESIAN_POINT('Ctrl Pts',(-3.17974169464408,0.528274395310344,304.656450830215));
#5016=CARTESIAN_POINT('Ctrl Pts',(-3.18859071179392,0.467981661138088,304.660235058849));
#5017=CARTESIAN_POINT('Ctrl Pts',(-3.20304617518148,0.369489433514989,304.666416850289));
#5018=CARTESIAN_POINT('Ctrl Pts',(-3.21295837398269,0.270160007624854,304.67259864173));
#5019=CARTESIAN_POINT('Ctrl Pts',(-3.21823943364067,0.170447969363531,304.67878043317));
#5020=CARTESIAN_POINT('Ctrl Pts',(-3.22351351591203,0.0708676716027387,
304.684954057169));
#5021=CARTESIAN_POINT('Ctrl Pts',(-3.22416859929969,-0.029093805070177,
304.691127681167));
#5022=CARTESIAN_POINT('Ctrl Pts',(-3.22016820776668,-0.128973936083073,
304.697301305165));
#5023=CARTESIAN_POINT('Ctrl Pts',(-3.21617193070947,-0.22875133855581,304.703468579478));
#5024=CARTESIAN_POINT('Ctrl Pts',(-3.2075297165177,-0.328447131537302,304.709635853792));
#5025=CARTESIAN_POINT('Ctrl Pts',(-3.19425710561108,-0.427596896332428,
304.715803128105));
#5026=CARTESIAN_POINT('Ctrl Pts',(-3.18099377706077,-0.526677319575138,
304.721966089262));
#5027=CARTESIAN_POINT('Ctrl Pts',(-3.16310654793605,-0.625212046189163,
304.72812905042));
#5028=CARTESIAN_POINT('Ctrl Pts',(-3.1406628783991,-0.722740788074029,304.734292011577));
#5029=CARTESIAN_POINT('Ctrl Pts',(-3.11822723160842,-0.820234667195105,
304.740452769714));
#5030=CARTESIAN_POINT('Ctrl Pts',(-3.09123847817242,-0.916722854915224,
304.74661352785));
#5031=CARTESIAN_POINT('Ctrl Pts',(-3.05981520363205,-1.01175514929361,304.752774285987));
#5032=CARTESIAN_POINT('Ctrl Pts',(-3.02839483363719,-1.10677865955807,304.758934474667));
#5033=CARTESIAN_POINT('Ctrl Pts',(-2.99254089362575,-1.20034613325871,304.765094663346));
#5034=CARTESIAN_POINT('Ctrl Pts',(-2.95242157408443,-1.29202337880583,304.771254852026));
#5035=CARTESIAN_POINT('Ctrl Pts',(-2.91229533031941,-1.38371644699806,304.777416103897));
#5036=CARTESIAN_POINT('Ctrl Pts',(-2.8679024181892,-1.47351824254347,304.783577355768));
#5037=CARTESIAN_POINT('Ctrl Pts',(-2.81945841049582,-1.56101628242129,304.78973860764));
#5038=CARTESIAN_POINT('Ctrl Pts',(-2.7709635936813,-1.64860609213236,304.795906321565));
#5039=CARTESIAN_POINT('Ctrl Pts',(-2.71840940790595,-1.73388694266899,304.80207403549));
#5040=CARTESIAN_POINT('Ctrl Pts',(-2.66205640614232,-1.81647275041952,304.808241749415));
#5041=CARTESIAN_POINT('Ctrl Pts',(-2.60567130385045,-1.89910560176969,304.814412976674));
#5042=CARTESIAN_POINT('Ctrl Pts',(-2.5454833361712,-1.97904000729206,304.820584203932));
#5043=CARTESIAN_POINT('Ctrl Pts',(-2.48179400269614,-2.0559221995692,304.826755431191));
#5044=CARTESIAN_POINT('Ctrl Pts',(-2.418003791556,-2.13292616570736,304.832936433068));
#5045=CARTESIAN_POINT('Ctrl Pts',(-2.35070143055836,-2.20686794414452,304.839117434946));
#5046=CARTESIAN_POINT('Ctrl Pts',(-2.28022599988325,-2.27742990055817,304.845298436824));
#5047=CARTESIAN_POINT('Ctrl Pts',(-2.23707760601933,-2.32063126957402,304.849082738686));
#5048=CARTESIAN_POINT('Ctrl Pts',(-2.19274048532147,-2.36256648331417,304.852867040547));
#5049=CARTESIAN_POINT('Ctrl Pts',(-2.14729831213303,-2.40317030632676,304.856651342409));
#5050=CARTESIAN_POINT('Ctrl Pts',(-2.07306817973536,-2.46949695724588,304.862833028022));
#5051=CARTESIAN_POINT('Ctrl Pts',(-1.99563638067943,-2.53249344176403,304.869014713635));
#5052=CARTESIAN_POINT('Ctrl Pts',(-1.91533385259366,-2.59183598933434,304.875196399248));
#5053=CARTESIAN_POINT('Ctrl Pts',(-1.83514776257405,-2.65109249065375,304.881369121463));
#5054=CARTESIAN_POINT('Ctrl Pts',(-1.75209956719673,-2.7067053372349,304.887541843678));
#5055=CARTESIAN_POINT('Ctrl Pts',(-1.66655500082802,-2.75838938362863,304.893714565893));
#5056=CARTESIAN_POINT('Ctrl Pts',(-1.60413541858516,-2.79610185002436,304.898218636207));
#5057=CARTESIAN_POINT('Ctrl Pts',(-1.54038748697828,-2.83172329355576,304.902722706522));
#5058=CARTESIAN_POINT('Ctrl Pts',(-1.47546400239266,-2.86515680899727,304.907226776837));
#5059=CARTESIAN_POINT('Origin',(0.,0.,294.689226550727));
#5060=CARTESIAN_POINT('',(-1.47546400239267,-2.86515680899727,306.403639991207));
#5061=CARTESIAN_POINT('',(-1.47546400238963,-2.86515680899883,306.154894777109));
#5062=CARTESIAN_POINT('',(-1.47546400239267,-2.86515680899727,294.689226550727));
#5063=CARTESIAN_POINT('',(3.22274909182747,0.00241942662847882,305.560773449333));
#5064=CARTESIAN_POINT('Ctrl Pts',(3.22274909182747,0.00241942662847882,
305.560773449333));
#5065=CARTESIAN_POINT('Ctrl Pts',(3.22266144451175,0.119168289285173,305.567961004005));
#5066=CARTESIAN_POINT('Ctrl Pts',(3.21622575765141,0.235660092573957,305.575148558678));
#5067=CARTESIAN_POINT('Ctrl Pts',(3.20354916784432,0.351269542807173,305.58233611335));
#5068=CARTESIAN_POINT('Ctrl Pts',(3.19074689796521,0.468025184899005,305.589594927912));
#5069=CARTESIAN_POINT('Ctrl Pts',(3.17157944877209,0.583880777920902,305.596853742474));
#5070=CARTESIAN_POINT('Ctrl Pts',(3.14620685056165,0.69821201363122,305.604112557036));
#5071=CARTESIAN_POINT('Ctrl Pts',(3.12176984277167,0.8083273937952,305.611103709717));
#5072=CARTESIAN_POINT('Ctrl Pts',(3.09157724993706,0.917028816844444,305.618094862397));
#5073=CARTESIAN_POINT('Ctrl Pts',(3.05581386047934,1.02377693498258,305.625086015078));
#5074=CARTESIAN_POINT('Ctrl Pts',(3.02418624482621,1.11818041584281,305.631268692204));
#5075=CARTESIAN_POINT('Ctrl Pts',(2.98812642735059,1.21127659330337,305.637451369331));
#5076=CARTESIAN_POINT('Ctrl Pts',(2.94776157123372,1.30262016016095,305.643634046457));
#5077=CARTESIAN_POINT('Ctrl Pts',(2.90745005343074,1.39384302519247,305.649808553764));
#5078=CARTESIAN_POINT('Ctrl Pts',(2.86284497866514,1.48331749083947,305.655983061071));
#5079=CARTESIAN_POINT('Ctrl Pts',(2.81412294498844,1.57061440620848,305.662157568379));
#5080=CARTESIAN_POINT('Ctrl Pts',(2.76545104354432,1.65782149796103,305.668325722465));
#5081=CARTESIAN_POINT('Ctrl Pts',(2.71267081576087,1.74285511862323,305.674493876552));
#5082=CARTESIAN_POINT('Ctrl Pts',(2.65600611370655,1.82530794291085,305.680662030638));
#5083=CARTESIAN_POINT('Ctrl Pts',(2.59938111668075,1.90770299240003,305.686825862691));
#5084=CARTESIAN_POINT('Ctrl Pts',(2.53887730176894,1.9875204856622,305.692989694744));
#5085=CARTESIAN_POINT('Ctrl Pts',(2.47476296555049,2.06438025248251,305.699153526797));
#5086=CARTESIAN_POINT('Ctrl Pts',(2.41067160505096,2.14121247618996,305.705315150008));
#5087=CARTESIAN_POINT('Ctrl Pts',(2.34297257137275,2.21508874797334,305.711476773218));
#5088=CARTESIAN_POINT('Ctrl Pts',(2.27197520644782,2.28566100368938,305.717638396429));
#5089=CARTESIAN_POINT('Ctrl Pts',(2.20098448217963,2.3562266585108,305.723799443319));
#5090=CARTESIAN_POINT('Ctrl Pts',(2.12669634706602,2.42348860692162,305.729960490209));
#5091=CARTESIAN_POINT('Ctrl Pts',(2.04945715566873,2.48713548677555,305.736121537099));
#5092=CARTESIAN_POINT('Ctrl Pts',(1.97220473453455,2.55079326823861,305.74228363927));
#5093=CARTESIAN_POINT('Ctrl Pts',(1.892000586925,2.61083447604423,305.748445741441));
#5094=CARTESIAN_POINT('Ctrl Pts',(1.80922352338026,2.66698852733707,305.754607843612));
#5095=CARTESIAN_POINT('Ctrl Pts',(1.72635988471605,2.72320130919476,305.760776390621));
#5096=CARTESIAN_POINT('Ctrl Pts',(1.64091831588962,2.77551857399083,305.766944937629));
#5097=CARTESIAN_POINT('Ctrl Pts',(1.55330582060207,2.82371361688535,305.773113484638));
#5098=CARTESIAN_POINT('Ctrl Pts',(1.46564354584226,2.8719360431319,305.779285536477));
#5099=CARTESIAN_POINT('Ctrl Pts',(1.37580827627961,2.91603139226436,305.785457588317));
#5100=CARTESIAN_POINT('Ctrl Pts',(1.28422894017585,2.95582029083549,305.791629640157));
#5101=CARTESIAN_POINT('Ctrl Pts',(1.19250489049869,2.99567206378351,305.797811445067));
#5102=CARTESIAN_POINT('Ctrl Pts',(1.09903167471182,3.03120364246141,305.803993249977));
#5103=CARTESIAN_POINT('Ctrl Pts',(1.00425541741988,3.06228486902881,305.810175054887));
#5104=CARTESIAN_POINT('Ctrl Pts',(0.946367589946561,3.08126878686438,305.813950802804));
#5105=CARTESIAN_POINT('Ctrl Pts',(0.887993923017348,3.09859345610937,305.817726550721));
#5106=CARTESIAN_POINT('Ctrl Pts',(0.829237818619394,3.11423862327076,305.821502298639));
#5107=CARTESIAN_POINT('Ctrl Pts',(0.73303586325626,3.13985461140222,305.827684368338));
#5108=CARTESIAN_POINT('Ctrl Pts',(0.635483189190926,3.16105208401201,305.833866438036));
#5109=CARTESIAN_POINT('Ctrl Pts',(0.537021435084952,3.17769185742723,305.840048507735));
#5110=CARTESIAN_POINT('Ctrl Pts',(0.438689601616051,3.19430967460185,305.846222420171));
#5111=CARTESIAN_POINT('Ctrl Pts',(0.339451495731243,3.20638167574098,305.852396332606));
#5112=CARTESIAN_POINT('Ctrl Pts',(0.239762506137257,3.21381883483665,305.858570245042));
#5113=CARTESIAN_POINT('Ctrl Pts',(0.140175888083489,3.22124835664525,305.86473781743));
#5114=CARTESIAN_POINT('Ctrl Pts',(0.0401397362372681,3.2240524679527,305.870905389818));
#5115=CARTESIAN_POINT('Ctrl Pts',(-0.0598827445386845,3.22219360365055,
305.877072962207));
#5116=CARTESIAN_POINT('Ctrl Pts',(-0.159835487309292,3.22033603539193,305.88323623442));
#5117=CARTESIAN_POINT('Ctrl Pts',(-0.259774146540478,3.21382196388716,305.889399506633));
#5118=CARTESIAN_POINT('Ctrl Pts',(-0.359233696008545,3.20266587613383,305.895562778846));
#5119=CARTESIAN_POINT('Ctrl Pts',(-0.458657821243816,3.19151376181343,305.901723855903));
#5120=CARTESIAN_POINT('Ctrl Pts',(-0.557602746265318,3.17572296510507,305.90788493296));
#5121=CARTESIAN_POINT('Ctrl Pts',(-0.655607631094898,3.15535991553264,305.914046010018));
#5122=CARTESIAN_POINT('Ctrl Pts',(-0.753603575423269,3.13499872358057,305.92020652503));
#5123=CARTESIAN_POINT('Ctrl Pts',(-0.850659226471839,3.1100661963613,305.926367040043));
#5124=CARTESIAN_POINT('Ctrl Pts',(-0.946323988758447,3.08067987152192,305.932527555056));
#5125=CARTESIAN_POINT('Ctrl Pts',(-1.04200536918741,3.05128844191754,305.938689140225));
#5126=CARTESIAN_POINT('Ctrl Pts',(-1.13629496728062,3.01744180488538,305.944850725395));
#5127=CARTESIAN_POINT('Ctrl Pts',(-1.22875834596989,2.97930704857847,305.951012310565));
#5128=CARTESIAN_POINT('Ctrl Pts',(-1.32131882448577,2.94113224530076,305.957180366284));
#5129=CARTESIAN_POINT('Ctrl Pts',(-1.41204885382933,2.89866049697703,305.963348422003));
#5130=CARTESIAN_POINT('Ctrl Pts',(-1.50053508857693,2.85210659170541,305.969516477722));
#5131=CARTESIAN_POINT('Ctrl Pts',(-1.58907180069417,2.80552612954964,305.975688052036));
#5132=CARTESIAN_POINT('Ctrl Pts',(-1.67536179601707,2.75485909172001,305.98185962635));
#5133=CARTESIAN_POINT('Ctrl Pts',(-1.75901915928313,2.70036463459564,305.988031200664));
#5134=CARTESIAN_POINT('Ctrl Pts',(-1.84280908563422,2.64578382579737,305.994212554427));
#5135=CARTESIAN_POINT('Ctrl Pts',(-1.92395769789876,2.58736373851854,306.000393908191));
#5136=CARTESIAN_POINT('Ctrl Pts',(-2.00211068653864,2.52540498957054,306.006575261954));
#5137=CARTESIAN_POINT('Ctrl Pts',(-2.04991652391241,2.48750509696709,306.010356368702));
#5138=CARTESIAN_POINT('Ctrl Pts',(-2.09660216060085,2.44828190783947,306.014137475451));
#5139=CARTESIAN_POINT('Ctrl Pts',(-2.14209342392823,2.4078108990665,306.017918582199));
#5140=CARTESIAN_POINT('Ctrl Pts',(-2.21641229141797,2.34169359833276,306.024095758888));
#5141=CARTESIAN_POINT('Ctrl Pts',(-2.2877942136428,2.27201918274831,306.030272935578));
#5142=CARTESIAN_POINT('Ctrl Pts',(-2.35587991540464,2.19907875863804,306.036450112267));
#5143=CARTESIAN_POINT('Ctrl Pts',(-2.42387544698635,2.12623493412226,306.042619108133));
#5144=CARTESIAN_POINT('Ctrl Pts',(-2.48858314210488,2.05013401311274,306.048788103999));
#5145=CARTESIAN_POINT('Ctrl Pts',(-2.5496779625577,1.97110625024316,306.054957099864));
#5146=CARTESIAN_POINT('Ctrl Pts',(-2.61070982913654,1.89215991987125,306.061119739018));
#5147=CARTESIAN_POINT('Ctrl Pts',(-2.66813595915531,1.81029308516022,306.067282378171));
#5148=CARTESIAN_POINT('Ctrl Pts',(-2.72166992036475,1.72587091263562,306.073445017324));
#5149=CARTESIAN_POINT('Ctrl Pts',(-2.77516648941635,1.64150770692628,306.079603352026));
#5150=CARTESIAN_POINT('Ctrl Pts',(-2.82477606335493,1.55459307714627,306.085761686727));
#5151=CARTESIAN_POINT('Ctrl Pts',(-2.87025462220028,1.46552242092638,306.091920021428));
#5152=CARTESIAN_POINT('Ctrl Pts',(-2.91571696477754,1.37648352458801,306.098076160255));
#5153=CARTESIAN_POINT('Ctrl Pts',(-2.95705102247069,1.28529051520153,306.104232299082));
#5154=CARTESIAN_POINT('Ctrl Pts',(-2.99405841563676,1.19236394035324,306.110388437908));
#5155=CARTESIAN_POINT('Ctrl Pts',(-3.03106246233952,1.09944576856569,306.116544020055));
#5156=CARTESIAN_POINT('Ctrl Pts',(-3.06374046223571,1.00479474580364,306.122699602201));
#5157=CARTESIAN_POINT('Ctrl Pts',(-3.09194232469225,0.908851045703676,306.128855184347));
#5158=CARTESIAN_POINT('Ctrl Pts',(-3.12014914255469,0.812890487143475,306.135011848103));
#5159=CARTESIAN_POINT('Ctrl Pts',(-3.14387813842437,0.715637215955306,306.141168511859));
#5160=CARTESIAN_POINT('Ctrl Pts',(-3.16302947394644,0.617545228664362,306.147325175615));
#5161=CARTESIAN_POINT('Ctrl Pts',(-3.18220108500312,0.519349391306045,306.153488357436));
#5162=CARTESIAN_POINT('Ctrl Pts',(-3.19678527627672,0.420313491141804,306.159651539257));
#5163=CARTESIAN_POINT('Ctrl Pts',(-3.20673363715653,0.320900206962954,306.165814721078));
#5164=CARTESIAN_POINT('Ctrl Pts',(-3.2166877094249,0.221429849272094,306.171981441203));
#5165=CARTESIAN_POINT('Ctrl Pts',(-3.22200062815385,0.121582108828924,306.178148161329));
#5166=CARTESIAN_POINT('Ctrl Pts',(-3.22267612359271,0.0218212035753486,
306.184314881454));
#5167=CARTESIAN_POINT('Ctrl Pts',(-3.22335269893809,-0.078099188251534,
306.190491460241));
#5168=CARTESIAN_POINT('Ctrl Pts',(-3.21937706276582,-0.17793203468609,306.196668039028));
#5169=CARTESIAN_POINT('Ctrl Pts',(-3.21080495877509,-0.27721666473225,306.202844617815));
#5170=CARTESIAN_POINT('Ctrl Pts',(-3.20548941632324,-0.338782841063894,
306.206674700463));
#5171=CARTESIAN_POINT('Ctrl Pts',(-3.19840746086269,-0.400138356556447,
306.210504783111));
#5172=CARTESIAN_POINT('Ctrl Pts',(-3.18958220591318,-0.461175578518668,
306.214334865759));
#5173=CARTESIAN_POINT('Ctrl Pts',(-3.17531600614771,-0.559843459120906,
306.220526270368));
#5174=CARTESIAN_POINT('Ctrl Pts',(-3.15644338444273,-0.658013392929032,
306.226717674978));
#5175=CARTESIAN_POINT('Ctrl Pts',(-3.13301053890264,-0.755223493824845,
306.232909079587));
#5176=CARTESIAN_POINT('Ctrl Pts',(-3.109608797346,-0.852304561250731,306.239092265931));
#5177=CARTESIAN_POINT('Ctrl Pts',(-3.08165896594509,-0.94842791267856,306.245275452275));
#5178=CARTESIAN_POINT('Ctrl Pts',(-3.0492587632197,-1.04313880065305,306.251458638618));
#5179=CARTESIAN_POINT('Ctrl Pts',(-3.01603218714236,-1.14026530789463,306.25779952831));
#5180=CARTESIAN_POINT('Ctrl Pts',(-2.97812518973203,-1.23590586522933,306.264140418001));
#5181=CARTESIAN_POINT('Ctrl Pts',(-2.93569870836832,-1.32958288804595,306.270481307692));
#5182=CARTESIAN_POINT('Ctrl Pts',(-2.89440134291617,-1.42076684017628,306.276653444302));
#5183=CARTESIAN_POINT('Ctrl Pts',(-2.84882222087939,-1.51009003848377,306.282825580912));
#5184=CARTESIAN_POINT('Ctrl Pts',(-2.79915925542181,-1.59713024681346,306.288997717523));
#5185=CARTESIAN_POINT('Ctrl Pts',(-2.74951451705358,-1.68413851001784,306.295167588862));
#5186=CARTESIAN_POINT('Ctrl Pts',(-2.69578912819948,-1.76886507464778,306.301337460201));
#5187=CARTESIAN_POINT('Ctrl Pts',(-2.63822703105574,-1.85091212517148,306.30750733154));
#5188=CARTESIAN_POINT('Ctrl Pts',(-2.58067093502755,-1.9329506219097,306.313676559641));
#5189=CARTESIAN_POINT('Ctrl Pts',(-2.51927917443115,-2.01230980750277,306.319845787742));
#5190=CARTESIAN_POINT('Ctrl Pts',(-2.45433856368175,-2.08862150169067,306.326015015844));
#5191=CARTESIAN_POINT('Ctrl Pts',(-2.38624504605583,-2.16863817589936,306.332483763791));
#5192=CARTESIAN_POINT('Ctrl Pts',(-2.3142497026075,-2.2453035666458,306.338952511738));
#5193=CARTESIAN_POINT('Ctrl Pts',(-2.23872910567104,-2.31823414562061,306.345421259684));
#5194=CARTESIAN_POINT('Ctrl Pts',(-2.16662622299446,-2.38786422261512,306.351597261904));
#5195=CARTESIAN_POINT('Ctrl Pts',(-2.09131057325942,-2.4540898996024,306.357773264123));
#5196=CARTESIAN_POINT('Ctrl Pts',(-2.01314499640124,-2.51661772742001,306.363949266342));
#5197=CARTESIAN_POINT('Ctrl Pts',(-1.93493489802835,-2.57918116981014,306.370128786286));
#5198=CARTESIAN_POINT('Ctrl Pts',(-1.85387198813786,-2.63804231506044,306.37630830623));
#5199=CARTESIAN_POINT('Ctrl Pts',(-1.77034878227916,-2.6929505661231,306.382487826174));
#5200=CARTESIAN_POINT('Ctrl Pts',(-1.6867174754312,-2.74792988289973,306.388675344041));
#5201=CARTESIAN_POINT('Ctrl Pts',(-1.60061988868109,-2.79894587746375,306.394862861909));
#5202=CARTESIAN_POINT('Ctrl Pts',(-1.51247353856827,-2.8457936252706,306.401050379776));
#5203=CARTESIAN_POINT('Ctrl Pts',(-1.50017648070243,-2.85232922731116,306.401913583586));
#5204=CARTESIAN_POINT('Ctrl Pts',(-1.4878395809603,-2.85878378235245,306.402776787397));
#5205=CARTESIAN_POINT('Ctrl Pts',(-1.47546400239267,-2.86515680899727,306.403639991207));
#5206=CARTESIAN_POINT('Ctrl Pts',(3.22274915228586,0.0023375073901473,305.562210368046));
#5207=CARTESIAN_POINT('Ctrl Pts',(3.22279738454772,-0.0641608838811988,
305.558419269476));
#5208=CARTESIAN_POINT('Ctrl Pts',(3.22078741422796,-0.130642986175323,305.554593488903));
#5209=CARTESIAN_POINT('Ctrl Pts',(3.21376905799516,-0.24523453273071,305.547898612221));
#5210=CARTESIAN_POINT('Ctrl Pts',(3.20973188335,-0.293381060341542,305.545055013601));
#5211=CARTESIAN_POINT('Ctrl Pts',(3.20079801594267,-0.377236269941363,305.540036903916));
#5212=CARTESIAN_POINT('Ctrl Pts',(3.19638170288744,-0.412987894215753,305.537876554609));
#5213=CARTESIAN_POINT('Ctrl Pts',(3.18678008582499,-0.481285696811891,305.533705256271));
#5214=CARTESIAN_POINT('Ctrl Pts',(3.18169300051384,-0.513841187180296,305.531697528279));
#5215=CARTESIAN_POINT('Ctrl Pts',(3.16990460305418,-0.582375680949159,305.527427145115));
#5216=CARTESIAN_POINT('Ctrl Pts',(3.16308784364899,-0.61832980479687,305.525161172483));
#5217=CARTESIAN_POINT('Ctrl Pts',(3.14447933456213,-0.708097190678513,305.519436008275));
#5218=CARTESIAN_POINT('Ctrl Pts',(3.13191760949911,-0.761737107938731,305.515953416078));
#5219=CARTESIAN_POINT('Ctrl Pts',(3.05734023786875,-1.04704244149266,305.497088532235));
#5220=CARTESIAN_POINT('Ctrl Pts',(2.97099276275974,-1.27153250959755,305.48094824535));
#5221=CARTESIAN_POINT('Ctrl Pts',(2.81407054632813,-1.57395003949105,305.457983127357));
#5222=CARTESIAN_POINT('Ctrl Pts',(2.76337950172971,-1.6613390229864,305.451198597535));
#5223=CARTESIAN_POINT('Ctrl Pts',(2.68515676415591,-1.78267591450199,305.441682256568));
#5224=CARTESIAN_POINT('Ctrl Pts',(2.66091118365575,-1.81866771901611,305.438846968483));
#5225=CARTESIAN_POINT('Ctrl Pts',(2.61605893058713,-1.88243139100973,305.433815529988));
#5226=CARTESIAN_POINT('Ctrl Pts',(2.59571828446063,-1.91038191911443,305.431607030086));
#5227=CARTESIAN_POINT('Ctrl Pts',(2.56226331397612,-1.95483196796648,305.428096855314));
#5228=CARTESIAN_POINT('Ctrl Pts',(2.54943041332456,-1.97153898075036,305.426778000909));
#5229=CARTESIAN_POINT('Ctrl Pts',(2.52313439430977,-2.00508732356597,305.424132674688));
#5230=CARTESIAN_POINT('Ctrl Pts',(2.50966434298004,-2.02192168314089,305.422806735148));
#5231=CARTESIAN_POINT('Ctrl Pts',(2.47266357033739,-2.06722432989454,305.41923866428));
#5232=CARTESIAN_POINT('Ctrl Pts',(2.44881012460269,-2.09542615990716,305.417017615641));
#5233=CARTESIAN_POINT('Ctrl Pts',(2.30227811936734,-2.26274961630145,305.403797837255));
#5234=CARTESIAN_POINT('Ctrl Pts',(2.16824835500139,-2.39149207429904,305.393433162139));
#5235=CARTESIAN_POINT('Ctrl Pts',(1.86767476857334,-2.63404527363734,305.371755889497));
#5236=CARTESIAN_POINT('Ctrl Pts',(1.700058864202,-2.74521274179289,305.360468491671));
#5237=CARTESIAN_POINT('Ctrl Pts',(1.47732750217437,-2.86466940300555,305.345533701254));
#5238=CARTESIAN_POINT('Ctrl Pts',(1.43086597756843,-2.88815675575768,305.342423901105));
#5239=CARTESIAN_POINT('Ctrl Pts',(1.35127887614507,-2.92599800070194,305.337094330183));
#5240=CARTESIAN_POINT('Ctrl Pts',(1.31844317752434,-2.94093970158709,305.334894801031));
#5241=CARTESIAN_POINT('Ctrl Pts',(1.25524343168215,-2.96842726017984,305.330656773708));
#5242=CARTESIAN_POINT('Ctrl Pts',(1.22492468307446,-2.98106623007257,305.328621721622));
#5243=CARTESIAN_POINT('Ctrl Pts',(1.14387956744896,-3.01340638411414,305.323174289503));
#5244=CARTESIAN_POINT('Ctrl Pts',(1.09284015930307,-3.0322892878481,305.319735805423));
#5245=CARTESIAN_POINT('Ctrl Pts',(0.815397097240796,-3.12701961240845,305.300992656832));
#5246=CARTESIAN_POINT('Ctrl Pts',(0.581602149451182,-3.17880935548137,305.284935039072));
#5247=CARTESIAN_POINT('Ctrl Pts',(0.242410204319315,-3.215253009967,305.261939713227));
#5248=CARTESIAN_POINT('Ctrl Pts',(0.140072620152158,-3.22133453201706,305.2550527869));
#5249=CARTESIAN_POINT('Ctrl Pts',(-0.00614124198249999,-3.22304122512347,
305.24541150769));
#5250=CARTESIAN_POINT('Ctrl Pts',(-0.0499056063542504,-3.22266073704752,
305.242551356178));
#5251=CARTESIAN_POINT('Ctrl Pts',(-0.128422588832258,-3.22037813324722,
305.2374807151));
#5252=CARTESIAN_POINT('Ctrl Pts',(-0.163177660860009,-3.21880427427332,
305.235257624708));
#5253=CARTESIAN_POINT('Ctrl Pts',(-0.218982064994394,-3.21537096920916,
305.231729555455));
#5254=CARTESIAN_POINT('Ctrl Pts',(-0.240049704208506,-3.21386680230251,
305.230407131546));
#5255=CARTESIAN_POINT('Ctrl Pts',(-0.282547455671316,-3.21041234903641,
305.227760779551));
#5256=CARTESIAN_POINT('Ctrl Pts',(-0.303975766826593,-3.20845434886205,
305.226437294569));
#5257=CARTESIAN_POINT('Ctrl Pts',(-0.361919166548094,-3.2025740706638,305.222884104706));
#5258=CARTESIAN_POINT('Ctrl Pts',(-0.398390459072767,-3.19824193193941,
305.220675181146));
#5259=CARTESIAN_POINT('Ctrl Pts',(-0.62256497884837,-3.16771949301166,305.207224627413));
#5260=CARTESIAN_POINT('Ctrl Pts',(-0.807748577709249,-3.12563464350403,
305.196647578715));
#5261=CARTESIAN_POINT('Ctrl Pts',(-1.1559066838095,-3.01347817234163,305.176117070411));
#5262=CARTESIAN_POINT('Ctrl Pts',(-1.31887666628459,-2.94579427557508,305.166204995306));
#5263=CARTESIAN_POINT('Ctrl Pts',(-1.47546404664855,-2.86515678620691,305.155887179421));
#5264=CARTESIAN_POINT('',(3.22274911409335,-0.00238958375982015,305.314226550667));
#5265=CARTESIAN_POINT('Ctrl Pts',(-1.47546400239266,-2.86515680899727,304.907226776837));
#5266=CARTESIAN_POINT('Ctrl Pts',(-1.38661581666349,-2.91091077935925,304.913390624609));
#5267=CARTESIAN_POINT('Ctrl Pts',(-1.29556523018675,-2.95256529986578,304.919554472382));
#5268=CARTESIAN_POINT('Ctrl Pts',(-1.20272725222983,-2.98991048682794,304.925718320154));
#5269=CARTESIAN_POINT('Ctrl Pts',(-1.10992910335228,-3.02723965206657,304.931879523531));
#5270=CARTESIAN_POINT('Ctrl Pts',(-1.01534548768882,-3.06026299628952,304.938040726907));
#5271=CARTESIAN_POINT('Ctrl Pts',(-0.919412680228528,-3.0888182021503,304.944201930284));
#5272=CARTESIAN_POINT('Ctrl Pts',(-0.823495604790409,-3.11736872524254,
304.950362123285));
#5273=CARTESIAN_POINT('Ctrl Pts',(-0.726230192106002,-3.14145244322592,
304.956522316285));
#5274=CARTESIAN_POINT('Ctrl Pts',(-0.628068269559386,-3.16095678731499,
304.962682509286));
#5275=CARTESIAN_POINT('Ctrl Pts',(-0.529896429498429,-3.18046310197072,
304.968843324665));
#5276=CARTESIAN_POINT('Ctrl Pts',(-0.430828324213773,-3.19538903968609,
304.975004140043));
#5277=CARTESIAN_POINT('Ctrl Pts',(-0.331325398497885,-3.20567325889745,
304.981164955422));
#5278=CARTESIAN_POINT('Ctrl Pts',(-0.231722120686853,-3.21596785009474,
304.987331984193));
#5279=CARTESIAN_POINT('Ctrl Pts',(-0.131683577892903,-3.22161132786834,
304.993499012964));
#5280=CARTESIAN_POINT('Ctrl Pts',(-0.0316756594900992,-3.2225943298988,
304.999666041735));
#5281=CARTESIAN_POINT('Ctrl Pts',(0.068382807393181,-3.2235778287825,305.005836187598));
#5282=CARTESIAN_POINT('Ctrl Pts',(0.168410186318461,-3.21989617493667,305.012006333462));
#5283=CARTESIAN_POINT('Ctrl Pts',(0.267943338381552,-3.21159211761347,305.018176479325));
#5284=CARTESIAN_POINT('Ctrl Pts',(0.367642069890415,-3.20327424598637,305.024356889601));
#5285=CARTESIAN_POINT('Ctrl Pts',(0.466844502000891,-3.19031866253762,305.030537299877));
#5286=CARTESIAN_POINT('Ctrl Pts',(0.565095113419139,-3.17281973570668,305.036717710153));
#5287=CARTESIAN_POINT('Ctrl Pts',(0.651733872217161,-3.15738893808573,305.042167682092));
#5288=CARTESIAN_POINT('Ctrl Pts',(0.737632465830545,-3.13842606930804,305.047617654031));
#5289=CARTESIAN_POINT('Ctrl Pts',(0.822488845369692,-3.11602786600865,305.053067625969));
#5290=CARTESIAN_POINT('Ctrl Pts',(0.918739972166001,-3.09062197057113,305.059249435079));
#5291=CARTESIAN_POINT('Ctrl Pts',(1.01397585255009,-3.06070922671192,305.06543124419));
#5292=CARTESIAN_POINT('Ctrl Pts',(1.10774393125943,-3.02638744136601,305.0716130533));
#5293=CARTESIAN_POINT('Ctrl Pts',(1.20138812469359,-2.99211100155645,305.077786695077));
#5294=CARTESIAN_POINT('Ctrl Pts',(1.29356796830591,-2.95343724725102,305.083960336855));
#5295=CARTESIAN_POINT('Ctrl Pts',(1.38384380190918,-2.91051436938861,305.090133978632));
#5296=CARTESIAN_POINT('Ctrl Pts',(1.47402678665652,-2.86763563778266,305.096301270808));
#5297=CARTESIAN_POINT('Ctrl Pts',(1.56230926626287,-2.82051665690766,305.102468562983));
#5298=CARTESIAN_POINT('Ctrl Pts',(1.64827027679501,-2.76935419495848,305.108635855159));
#5299=CARTESIAN_POINT('Ctrl Pts',(1.73417117034408,-2.71822751356654,305.114798834228));
#5300=CARTESIAN_POINT('Ctrl Pts',(1.81775345210234,-2.66306319446985,305.120961813297));
#5301=CARTESIAN_POINT('Ctrl Pts',(1.89862035653628,-2.60410412699762,305.127124792366));
#5302=CARTESIAN_POINT('Ctrl Pts',(1.97945835455678,-2.54516613483665,305.133285568438));
#5303=CARTESIAN_POINT('Ctrl Pts',(2.05758255485718,-2.48243634467617,305.139446344509));
#5304=CARTESIAN_POINT('Ctrl Pts',(2.13262555474417,-2.41620069649691,305.14560712058));
#5305=CARTESIAN_POINT('Ctrl Pts',(2.20766161821294,-2.3499711706496,305.151767327195));
#5306=CARTESIAN_POINT('Ctrl Pts',(2.27961672326234,-2.28023671765377,305.15792753381));
#5307=CARTESIAN_POINT('Ctrl Pts',(2.34815768035134,-2.2073226023187,305.164087740424));
#5308=CARTESIAN_POINT('Ctrl Pts',(2.41671046669684,-2.13439590297826,305.170249010209));
#5309=CARTESIAN_POINT('Ctrl Pts',(2.48184763821471,-2.05828876652911,305.176410279993));
#5310=CARTESIAN_POINT('Ctrl Pts',(2.54327458513247,-1.97936149985779,305.182571549778));
#5311=CARTESIAN_POINT('Ctrl Pts',(2.60476595634082,-1.90035145464352,305.188739281472));
#5312=CARTESIAN_POINT('Ctrl Pts',(2.66253906736249,-1.81851571582787,305.194907013167));
#5313=CARTESIAN_POINT('Ctrl Pts',(2.71634125793352,-1.73424558034557,305.201074744862));
#5314=CARTESIAN_POINT('Ctrl Pts',(2.77017409543476,-1.64992744271069,305.207245989835));
#5315=CARTESIAN_POINT('Ctrl Pts',(2.82003129213083,-1.56317252181083,305.213417234808));
#5316=CARTESIAN_POINT('Ctrl Pts',(2.8657059933397,-1.47439707075025,305.219588479781));
#5317=CARTESIAN_POINT('Ctrl Pts',(2.91145303664756,-1.38548101225713,305.22576949911));
#5318=CARTESIAN_POINT('Ctrl Pts',(2.95300417532736,-1.29453842608024,305.231950518439));
#5319=CARTESIAN_POINT('Ctrl Pts',(2.99020054766132,-1.20200592646873,305.238131537769));
#5320=CARTESIAN_POINT('Ctrl Pts',(3.01297279197949,-1.14535597497329,305.241915661689));
#5321=CARTESIAN_POINT('Ctrl Pts',(3.03411379820523,-1.0881104430503,305.245699785609));
#5322=CARTESIAN_POINT('Ctrl Pts',(3.05359645756159,-1.03037189250643,305.24948390953));
#5323=CARTESIAN_POINT('Ctrl Pts',(3.09095665410658,-0.919651710159401,305.256740393916));
#5324=CARTESIAN_POINT('Ctrl Pts',(3.12231949147421,-0.806813452707642,305.263996878302));
#5325=CARTESIAN_POINT('Ctrl Pts',(3.14747759241214,-0.692461094765246,305.271253362688));
#5326=CARTESIAN_POINT('Ctrl Pts',(3.17240408855982,-0.579161461507495,305.278443044077));
#5327=CARTESIAN_POINT('Ctrl Pts',(3.19123950516091,-0.464375585045444,305.285632725466));
#5328=CARTESIAN_POINT('Ctrl Pts',(3.2038286399983,-0.348711353452439,305.292822406854));
#5329=CARTESIAN_POINT('Ctrl Pts',(3.21632152797467,-0.233931401785546,305.299957121459));
#5330=CARTESIAN_POINT('Ctrl Pts',(3.22266317951585,-0.11828658144667,305.307091836063));
#5331=CARTESIAN_POINT('Ctrl Pts',(3.22274911409335,-0.00238958375982015,
305.314226550667));
#5332=CARTESIAN_POINT('Ctrl Pts',(-1.47546400238914,-2.86515680899909,306.154894777109));
#5333=CARTESIAN_POINT('Ctrl Pts',(-1.54120577339087,-2.83130190225831,306.15009572013));
#5334=CARTESIAN_POINT('Ctrl Pts',(-1.60576667935371,-2.79519238498628,306.145364940917));
#5335=CARTESIAN_POINT('Ctrl Pts',(-1.70378779340339,-2.7358500295457,306.13815242811));
#5336=CARTESIAN_POINT('Ctrl Pts',(-1.73814339871503,-2.7141529048128,306.135618390634));
#5337=CARTESIAN_POINT('Ctrl Pts',(-1.8013865847504,-2.67251846954085,306.13093951029));
#5338=CARTESIAN_POINT('Ctrl Pts',(-1.83037619021467,-2.65274796191372,306.12878905642));
#5339=CARTESIAN_POINT('Ctrl Pts',(-1.8952869281816,-2.60690895150876,306.123957630973));
#5340=CARTESIAN_POINT('Ctrl Pts',(-1.93100442929171,-2.58056369834513,306.121287479076));
#5341=CARTESIAN_POINT('Ctrl Pts',(-2.04565014840141,-2.49228730828378,306.112665485442));
#5342=CARTESIAN_POINT('Ctrl Pts',(-2.122235963126,-2.42740554134186,306.106826040344));
#5343=CARTESIAN_POINT('Ctrl Pts',(-2.31623079573151,-2.24684584400522,306.091637293359));
#5344=CARTESIAN_POINT('Ctrl Pts',(-2.42800778127637,-2.12556377185198,306.082471941505));
#5345=CARTESIAN_POINT('Ctrl Pts',(-2.61522231912282,-1.88829198837817,306.065460915656));
#5346=CARTESIAN_POINT('Ctrl Pts',(-2.69341070268958,-1.77498344110131,306.057659415432));
#5347=CARTESIAN_POINT('Ctrl Pts',(-2.78392762681998,-1.62399175666936,306.047214502878));
#5348=CARTESIAN_POINT('Ctrl Pts',(-2.80314423472668,-1.59059245870692,306.044900923218));
#5349=CARTESIAN_POINT('Ctrl Pts',(-2.83233754541609,-1.53768050607672,306.04121806514));
#5350=CARTESIAN_POINT('Ctrl Pts',(-2.84272246467814,-1.51839594174772,306.039872192632));
#5351=CARTESIAN_POINT('Ctrl Pts',(-2.86260852849442,-1.48054880777078,306.037220927243));
#5352=CARTESIAN_POINT('Ctrl Pts',(-2.87212753092623,-1.46199716964992,306.035916614605));
#5353=CARTESIAN_POINT('Ctrl Pts',(-2.89642247136811,-1.41349557703836,306.032496764883));
#5354=CARTESIAN_POINT('Ctrl Pts',(-2.91091381170227,-1.38340646970513,306.030365569318));
#5355=CARTESIAN_POINT('Ctrl Pts',(-2.94232481132743,-1.31550669998958,306.025543578747));
#5356=CARTESIAN_POINT('Ctrl Pts',(-2.95898824271441,-1.27758422570415,306.022841835903));
#5357=CARTESIAN_POINT('Ctrl Pts',(-3.01073482689689,-1.15337286075936,306.013987431154));
#5358=CARTESIAN_POINT('Ctrl Pts',(-3.04280824483958,-1.06588436263582,306.007744111887));
#5359=CARTESIAN_POINT('Ctrl Pts',(-3.14979881620179,-0.729622568371299,
305.983981210183));
#5360=CARTESIAN_POINT('Ctrl Pts',(-3.19835445754483,-0.473449805534653,
305.966451779303));
#5361=CARTESIAN_POINT('Ctrl Pts',(-3.21904268845474,-0.162873764190184,
305.946605969192));
#5362=CARTESIAN_POINT('Ctrl Pts',(-3.22123245658054,-0.111470311267066,
305.943362372282));
#5363=CARTESIAN_POINT('Ctrl Pts',(-3.22285439103549,-0.0244166800758755,
305.937935643973));
#5364=CARTESIAN_POINT('Ctrl Pts',(-3.22292740963356,0.0112103012952112,
305.935733497365));
#5365=CARTESIAN_POINT('Ctrl Pts',(-3.22186683887805,0.0841854093056658,
305.931258748623));
#5366=CARTESIAN_POINT('Ctrl Pts',(-3.22067452399695,0.121527354379492,305.928988275965));
#5367=CARTESIAN_POINT('Ctrl Pts',(-3.21592207828865,0.217833069758899,305.923177320646));
#5368=CARTESIAN_POINT('Ctrl Pts',(-3.21138970784864,0.27673604173398,305.919666645779));
#5369=CARTESIAN_POINT('Ctrl Pts',(-3.1977306672811,0.407235606546508,305.91196103802));
#5370=CARTESIAN_POINT('Ctrl Pts',(-3.18781314804363,0.478717546992175,305.90778911631));
#5371=CARTESIAN_POINT('Ctrl Pts',(-3.14506201187071,0.72563285301452,305.893453819092));
#5372=CARTESIAN_POINT('Ctrl Pts',(-3.10007053350801,0.89862195044624,305.883560934002));
#5373=CARTESIAN_POINT('Ctrl Pts',(-2.9979694329104,1.18961433340329,305.86614767089));
#5374=CARTESIAN_POINT('Ctrl Pts',(-2.94757466662236,1.30950366840756,305.858722798735));
#5375=CARTESIAN_POINT('Ctrl Pts',(-2.87581245723878,1.45494369530914,305.849026643093));
#5376=CARTESIAN_POINT('Ctrl Pts',(-2.86110370898222,1.48365893473528,305.847077081509));
#5377=CARTESIAN_POINT('Ctrl Pts',(-2.83723961823572,1.5285728235668,305.843964348531));
#5378=CARTESIAN_POINT('Ctrl Pts',(-2.82837039630401,1.54492213356405,305.8428177914));
#5379=CARTESIAN_POINT('Ctrl Pts',(-2.80893920972284,1.58001292826479,305.840325752334));
#5380=CARTESIAN_POINT('Ctrl Pts',(-2.79833024049248,1.5987270379951,305.838977378938));
#5381=CARTESIAN_POINT('Ctrl Pts',(-2.7691493039314,1.64902149702494,305.835303875091));
#5382=CARTESIAN_POINT('Ctrl Pts',(-2.75022537698769,1.68039277687754,305.832958859233));
#5383=CARTESIAN_POINT('Ctrl Pts',(-2.70585547743292,1.75118962371925,305.827554762237));
#5384=CARTESIAN_POINT('Ctrl Pts',(-2.6800750937533,1.79039550089485,305.824480701171));
#5385=CARTESIAN_POINT('Ctrl Pts',(-2.58761037021346,1.924538424704,305.813710933626));
#5386=CARTESIAN_POINT('Ctrl Pts',(-2.51666458427771,2.01642576769474,305.805886723518));
#5387=CARTESIAN_POINT('Ctrl Pts',(-2.30197280152104,2.26546343879954,305.78371283706));
#5388=CARTESIAN_POINT('Ctrl Pts',(-2.1473806643742,2.41250575573752,305.769457067012));
#5389=CARTESIAN_POINT('Ctrl Pts',(-1.93424294673985,2.57839022501302,305.752148225552));
#5390=CARTESIAN_POINT('Ctrl Pts',(-1.88815583062837,2.61232849006755,305.748524920742));
#5391=CARTESIAN_POINT('Ctrl Pts',(-1.8107974012959,2.66617729254169,305.742632743126));
#5392=CARTESIAN_POINT('Ctrl Pts',(-1.78004455512285,2.68680668153204,305.740337609816));
#5393=CARTESIAN_POINT('Ctrl Pts',(-1.71844550132972,2.72660611407057,305.735830293627));
#5394=CARTESIAN_POINT('Ctrl Pts',(-1.68761732113617,2.74579383478301,305.733617695064));
#5395=CARTESIAN_POINT('Ctrl Pts',(-1.61078391801753,2.79183262629923,305.728204213755));
#5396=CARTESIAN_POINT('Ctrl Pts',(-1.56442399183894,2.81807244273501,305.725025114396));
#5397=CARTESIAN_POINT('Ctrl Pts',(-1.46220591709482,2.87262776001456,305.718186161945));
#5398=CARTESIAN_POINT('Ctrl Pts',(-1.40612978071229,2.90048893601899,305.714541314258));
#5399=CARTESIAN_POINT('Ctrl Pts',(-1.2278848961713,2.9826638765305,305.7032337901));
#5400=CARTESIAN_POINT('Ctrl Pts',(-1.10312596642887,3.0310230538844,305.695723447262));
#5401=CARTESIAN_POINT('Ctrl Pts',(-0.79728409916959,3.12817972548102,305.677711786067));
#5402=CARTESIAN_POINT('Ctrl Pts',(-0.614266223535925,3.1692005441263,305.66725728637));
#5403=CARTESIAN_POINT('Ctrl Pts',(-0.392195285316613,3.19900930278619,305.653938465533));
#5404=CARTESIAN_POINT('Ctrl Pts',(-0.355563765608199,3.2032876572366,305.65172063925));
#5405=CARTESIAN_POINT('Ctrl Pts',(-0.297409615858438,3.20906997831661,305.648155534628));
#5406=CARTESIAN_POINT('Ctrl Pts',(-0.275930400798075,3.21098815925837,305.64682923957));
#5407=CARTESIAN_POINT('Ctrl Pts',(-0.233376210144597,3.21435830760118,305.644179945453));
#5408=CARTESIAN_POINT('Ctrl Pts',(-0.212303112336628,3.21581888529505,305.642857431246));
#5409=CARTESIAN_POINT('Ctrl Pts',(-0.156536700056764,3.21913355842895,305.639332343744));
#5410=CARTESIAN_POINT('Ctrl Pts',(-0.121825882328664,3.2206339186488,305.637112393289));
#5411=CARTESIAN_POINT('Ctrl Pts',(-0.0434422639353102,3.22275311761159,
305.632050916455));
#5412=CARTESIAN_POINT('Ctrl Pts',(0.000232304049122911,3.22304584098117,
305.629196859065));
#5413=CARTESIAN_POINT('Ctrl Pts',(0.145939241060622,3.22106097320073,305.619589374183));
#5414=CARTESIAN_POINT('Ctrl Pts',(0.247853123107453,3.21482488036991,305.612730821619));
#5415=CARTESIAN_POINT('Ctrl Pts',(0.587494445676255,3.17779508729527,305.589701226514));
#5416=CARTESIAN_POINT('Ctrl Pts',(0.822094956060486,3.12533609918711,305.573578857673));
#5417=CARTESIAN_POINT('Ctrl Pts',(1.10009290415081,3.02966391329495,305.554784270479));
#5418=CARTESIAN_POINT('Ctrl Pts',(1.15100003995775,3.01069216165385,305.551351922311));
#5419=CARTESIAN_POINT('Ctrl Pts',(1.23188900686097,2.97819513156612,305.545910211351));
#5420=CARTESIAN_POINT('Ctrl Pts',(1.26218401024456,2.96548283012213,305.543874887003));
#5421=CARTESIAN_POINT('Ctrl Pts',(1.32537656401891,2.93782228223062,305.539633278719));
#5422=CARTESIAN_POINT('Ctrl Pts',(1.35822790940455,2.92277948291799,305.537430493718));
#5423=CARTESIAN_POINT('Ctrl Pts',(1.43794330569549,2.88464302977454,305.532086715117));
#5424=CARTESIAN_POINT('Ctrl Pts',(1.48451289960264,2.86095582990454,305.528966181846));
#5425=CARTESIAN_POINT('Ctrl Pts',(1.58414514037029,2.80719062900998,305.522277421181));
#5426=CARTESIAN_POINT('Ctrl Pts',(1.63697163585747,2.77671739887506,305.518722995895));
#5427=CARTESIAN_POINT('Ctrl Pts',(1.79728754809476,2.67807200151811,305.507864346878));
#5428=CARTESIAN_POINT('Ctrl Pts',(1.90162988284369,2.60501793374903,305.500698250105));
#5429=CARTESIAN_POINT('Ctrl Pts',(2.15794215086522,2.40193704988895,305.482338349691));
#5430=CARTESIAN_POINT('Ctrl Pts',(2.30261310545755,2.26361892423968,305.471225653588));
#5431=CARTESIAN_POINT('Ctrl Pts',(2.45696749190021,2.08583453884996,305.457211670341));
#5432=CARTESIAN_POINT('Ctrl Pts',(2.47994749324397,2.05845941820207,305.455059906568));
#5433=CARTESIAN_POINT('Ctrl Pts',(2.5159050079647,2.01414855464152,305.451576199186));
#5434=CARTESIAN_POINT('Ctrl Pts',(2.52917844559253,1.99745556677226,305.450263635706));
#5435=CARTESIAN_POINT('Ctrl Pts',(2.55539839805466,1.96380036679041,305.447614244218));
#5436=CARTESIAN_POINT('Ctrl Pts',(2.56834408048018,1.94683884243167,305.44627747202));
#5437=CARTESIAN_POINT('Ctrl Pts',(2.60255309698528,1.90108289034236,305.442670059651));
#5438=CARTESIAN_POINT('Ctrl Pts',(2.62350615554648,1.87206142787561,305.440380663702));
#5439=CARTESIAN_POINT('Ctrl Pts',(2.73341057930168,1.71436657637412,305.427959100111));
#5440=CARTESIAN_POINT('Ctrl Pts',(2.81338168121197,1.57970313136928,305.417426739239));
#5441=CARTESIAN_POINT('Ctrl Pts',(2.98280767114599,1.2404162234776,305.391852585261));
#5442=CARTESIAN_POINT('Ctrl Pts',(3.0614300791327,1.03123601340176,305.376899055731));
#5443=CARTESIAN_POINT('Ctrl Pts',(3.13208222382635,0.761147541781223,305.35902161058));
#5444=CARTESIAN_POINT('Ctrl Pts',(3.14489648417329,0.706336577932702,305.35546044052));
#5445=CARTESIAN_POINT('Ctrl Pts',(3.16371501180644,0.615128125025562,305.349641203021));
#5446=CARTESIAN_POINT('Ctrl Pts',(3.17054145761828,0.578914784215165,305.347358166146));
#5447=CARTESIAN_POINT('Ctrl Pts',(3.18231225242936,0.509999502206581,305.343062923321));
#5448=CARTESIAN_POINT('Ctrl Pts',(3.18737719530871,0.477323268478193,305.341047245641));
#5449=CARTESIAN_POINT('Ctrl Pts',(3.19688425795968,0.409064745182176,305.336877370407));
#5450=CARTESIAN_POINT('Ctrl Pts',(3.20123723659135,0.373474535477898,305.334726120791));
#5451=CARTESIAN_POINT('Ctrl Pts',(3.21002020796147,0.290147473544569,305.329737832409));
#5452=CARTESIAN_POINT('Ctrl Pts',(3.21398082970572,0.242369215415285,305.326914654041));
#5453=CARTESIAN_POINT('Ctrl Pts',(3.22083683804161,0.128987203713608,305.32028691449));
#5454=CARTESIAN_POINT('Ctrl Pts',(3.2227961534329,0.0633484734362306,305.316507037163));
#5455=CARTESIAN_POINT('Ctrl Pts',(3.22274917497873,-0.00230600822049255,
305.312761555685));
#5456=CARTESIAN_POINT('Origin',(0.,0.,177.));
#5457=CARTESIAN_POINT('',(3.933,-4.81653586104654E-16,177.));
#5458=CARTESIAN_POINT('Origin',(0.,0.,177.));
#5459=CARTESIAN_POINT('',(-1.8148060950507,-3.48926465567845,297.));
#5460=CARTESIAN_POINT('',(1.74869447533119,-3.52286199445084,297.));
#5461=CARTESIAN_POINT('Origin',(0.,0.,297.));
#5462=CARTESIAN_POINT('',(3.93481960852658,-0.00239843926903071,297.220836477965));
#5463=CARTESIAN_POINT('Ctrl Pts',(1.74869447533119,-3.52286199445084,297.));
#5464=CARTESIAN_POINT('Ctrl Pts',(2.90806357314772,-2.94736901759993,297.06547209452));
#5465=CARTESIAN_POINT('Ctrl Pts',(3.85617209864057,-1.61095470252649,297.139084253842));
#5466=CARTESIAN_POINT('Ctrl Pts',(3.93703630563088,-0.162725864948754,297.212696413163));
#5467=CARTESIAN_POINT('Ctrl Pts',(3.93582492032101,-0.00239905204916439,
297.220836477965));
#5468=CARTESIAN_POINT('',(3.93299999230081,-0.000246093130879474,298.470836477922));
#5469=CARTESIAN_POINT('Ctrl Pts',(3.93299926936306,-0.00239732969518293,
297.220836477965));
#5470=CARTESIAN_POINT('Ctrl Pts',(3.93306845839146,0.111112463605089,297.22660373228));
#5471=CARTESIAN_POINT('Ctrl Pts',(3.92821947420302,0.224824526215857,297.232370986595));
#5472=CARTESIAN_POINT('Ctrl Pts',(3.91842619360132,0.338267889843326,297.238138240911));
#5473=CARTESIAN_POINT('Ctrl Pts',(3.90864407754512,0.451581925654531,297.243898920435));
#5474=CARTESIAN_POINT('Ctrl Pts',(3.89392890351192,0.564627447569545,297.249659599959));
#5475=CARTESIAN_POINT('Ctrl Pts',(3.87430656947808,0.676932497150927,297.255420279483));
#5476=CARTESIAN_POINT('Ctrl Pts',(3.85470123276484,0.78914026549506,297.261175968973));
#5477=CARTESIAN_POINT('Ctrl Pts',(3.83019726034436,0.900608416330806,297.266931658463));
#5478=CARTESIAN_POINT('Ctrl Pts',(3.80087237107529,1.01087003061545,297.272687347953));
#5479=CARTESIAN_POINT('Ctrl Pts',(3.77156117378215,1.12108016305631,297.278440350076));
#5480=CARTESIAN_POINT('Ctrl Pts',(3.73743364047043,1.23008446439066,297.284193352198));
#5481=CARTESIAN_POINT('Ctrl Pts',(3.69861844832742,1.33742684797788,297.28994635432));
#5482=CARTESIAN_POINT('Ctrl Pts',(3.65981124973277,1.4447471256193,297.295698171677));
#5483=CARTESIAN_POINT('Ctrl Pts',(3.61631845628518,1.55040576251832,297.301449989034));
#5484=CARTESIAN_POINT('Ctrl Pts',(3.56831812451651,1.65396334972906,297.30720180639));
#5485=CARTESIAN_POINT('Ctrl Pts',(3.52031515156675,1.75752663511586,297.312953940237));
#5486=CARTESIAN_POINT('Ctrl Pts',(3.46780432886449,1.85898825253657,297.318706074083));
#5487=CARTESIAN_POINT('Ctrl Pts',(3.41101082659864,1.95793108684316,297.324458207929));
#5488=CARTESIAN_POINT('Ctrl Pts',(3.3541638766531,2.05696703505725,297.330215755038));
#5489=CARTESIAN_POINT('Ctrl Pts',(3.29302641127215,2.15347909324372,297.335973302148));
#5490=CARTESIAN_POINT('Ctrl Pts',(3.22786831331998,2.24707702401694,297.341730849258));
#5491=CARTESIAN_POINT('Ctrl Pts',(3.16268027161153,2.3407179682254,297.34749104228));
#5492=CARTESIAN_POINT('Ctrl Pts',(3.09346817959316,2.43144177848841,297.353251235301));
#5493=CARTESIAN_POINT('Ctrl Pts',(3.02054257162309,2.5188909410716,297.359011428323));
#5494=CARTESIAN_POINT('Ctrl Pts',(2.94749854717352,2.60648210345782,297.364780974737));
#5495=CARTESIAN_POINT('Ctrl Pts',(2.87072925049777,2.69078767941243,297.37055052115));
#5496=CARTESIAN_POINT('Ctrl Pts',(2.79058269164137,2.77148646778432,297.376320067564));
#5497=CARTESIAN_POINT('Ctrl Pts',(2.71412260721627,2.84847338100879,297.381824234083));
#5498=CARTESIAN_POINT('Ctrl Pts',(2.63458931482961,2.92217775913654,297.387328400602));
#5499=CARTESIAN_POINT('Ctrl Pts',(2.55231123269053,2.99235632428388,297.39283256712));
#5500=CARTESIAN_POINT('Ctrl Pts',(2.46440430868021,3.06733597418787,297.398713286935));
#5501=CARTESIAN_POINT('Ctrl Pts',(2.37304650350017,3.1385615346114,297.404594006749));
#5502=CARTESIAN_POINT('Ctrl Pts',(2.27859167607231,3.2056994515603,297.410474726564));
#5503=CARTESIAN_POINT('Ctrl Pts',(2.18425831965925,3.27275102765054,297.416347883641));
#5504=CARTESIAN_POINT('Ctrl Pts',(2.08683619493552,3.33572517840853,297.422221040719));
#5505=CARTESIAN_POINT('Ctrl Pts',(1.98671351319032,3.39432738793814,297.428094197796));
#5506=CARTESIAN_POINT('Ctrl Pts',(1.88669302508281,3.45286978311935,297.433961360235));
#5507=CARTESIAN_POINT('Ctrl Pts',(1.78397781660011,3.5070489067515,297.439828522674));
#5508=CARTESIAN_POINT('Ctrl Pts',(1.67898593072027,3.55661288931525,297.445695685113));
#5509=CARTESIAN_POINT('Ctrl Pts',(1.57195010680406,3.60714176272126,297.451677067012));
#5510=CARTESIAN_POINT('Ctrl Pts',(1.46254838908129,3.65287367102504,297.45765844891));
#5511=CARTESIAN_POINT('Ctrl Pts',(1.3512514380898,3.69359019804042,297.463639830809));
#5512=CARTESIAN_POINT('Ctrl Pts',(1.24220562620391,3.73348317539526,297.469500230753));
#5513=CARTESIAN_POINT('Ctrl Pts',(1.13134093193654,3.76856160093073,297.475360630697));
#5514=CARTESIAN_POINT('Ctrl Pts',(1.01912052783599,3.79866849695302,297.481221030641));
#5515=CARTESIAN_POINT('Ctrl Pts',(0.906917788079268,3.82877065392124,297.487080508113));
#5516=CARTESIAN_POINT('Ctrl Pts',(0.793360160715912,3.85390273093425,297.492939985585));
#5517=CARTESIAN_POINT('Ctrl Pts',(0.678925050333358,3.87395789549007,297.498799463058));
#5518=CARTESIAN_POINT('Ctrl Pts',(0.564480460267666,3.89401472139445,297.504659425923));
#5519=CARTESIAN_POINT('Ctrl Pts',(0.449158648561752,3.90899372783572,297.510519388788));
#5520=CARTESIAN_POINT('Ctrl Pts',(0.333445570025453,3.91883950319867,297.516379351654));
#5521=CARTESIAN_POINT('Ctrl Pts',(0.213536475921912,3.92904230844292,297.522451809906));
#5522=CARTESIAN_POINT('Ctrl Pts',(0.0932076757285175,3.9337324905987,297.528524268158));
#5523=CARTESIAN_POINT('Ctrl Pts',(-0.0269975551490727,3.93290733834602,
297.534596726411));
#5524=CARTESIAN_POINT('Ctrl Pts',(-0.143162287133464,3.9321099222138,297.540465069079));
#5525=CARTESIAN_POINT('Ctrl Pts',(-0.259211207929003,3.92616206917407,297.546333411748));
#5526=CARTESIAN_POINT('Ctrl Pts',(-0.374658128173509,3.91511433894255,297.552201754417));
#5527=CARTESIAN_POINT('Ctrl Pts',(-0.496128345835865,3.90349020732382,297.558376270461));
#5528=CARTESIAN_POINT('Ctrl Pts',(-0.616931525781467,3.88621976691363,297.564550786505));
#5529=CARTESIAN_POINT('Ctrl Pts',(-0.736513664123003,3.86342291531229,297.570725302549));
#5530=CARTESIAN_POINT('Ctrl Pts',(-0.85609580246454,3.84062606371095,297.576899818593));
#5531=CARTESIAN_POINT('Ctrl Pts',(-0.974456405796253,3.8123029905964,297.583074334637));
#5532=CARTESIAN_POINT('Ctrl Pts',(-1.09106157979183,3.77863383104293,297.589248850681));
#5533=CARTESIAN_POINT('Ctrl Pts',(-1.20228880561966,3.74651752706804,297.595138591821));
#5534=CARTESIAN_POINT('Ctrl Pts',(-1.31227030455785,3.709435880047,297.601028332961));
#5535=CARTESIAN_POINT('Ctrl Pts',(-1.42053173693775,3.66750304490025,297.606918074101));
#5536=CARTESIAN_POINT('Ctrl Pts',(-1.52865914675956,3.6256221206299,297.612800524018));
#5537=CARTESIAN_POINT('Ctrl Pts',(-1.63507034575995,3.57890210032103,297.618682973936));
#5538=CARTESIAN_POINT('Ctrl Pts',(-1.73930492813322,3.52750724548817,297.624565423854));
#5539=CARTESIAN_POINT('Ctrl Pts',(-1.84343785049158,3.4761625160704,297.630442136616));
#5540=CARTESIAN_POINT('Ctrl Pts',(-1.94539801331448,3.42015220315325,297.636318849379));
#5541=CARTESIAN_POINT('Ctrl Pts',(-2.04474441607394,3.3596888654955,297.642195562142));
#5542=CARTESIAN_POINT('Ctrl Pts',(-2.14580137930282,3.29818446150446,297.648173460979));
#5543=CARTESIAN_POINT('Ctrl Pts',(-2.24415333475831,3.23207241709213,297.654151359817));
#5544=CARTESIAN_POINT('Ctrl Pts',(-2.33936135744235,3.16162575889454,297.660129258654));
#5545=CARTESIAN_POINT('Ctrl Pts',(-2.43285922939206,3.09244448150049,297.665999780951));
#5546=CARTESIAN_POINT('Ctrl Pts',(-2.52332483473946,3.01908327348623,297.671870303248));
#5547=CARTESIAN_POINT('Ctrl Pts',(-2.61037181737141,2.94184431523375,297.677740825546));
#5548=CARTESIAN_POINT('Ctrl Pts',(-2.69740801732825,2.86461492471775,297.68361062065));
#5549=CARTESIAN_POINT('Ctrl Pts',(-2.78102612986177,2.78350901163158,297.689480415754));
#5550=CARTESIAN_POINT('Ctrl Pts',(-2.86087395423676,2.69886813645456,297.695350210859));
#5551=CARTESIAN_POINT('Ctrl Pts',(-2.94073087962143,2.61421761395866,297.701220674999));
#5552=CARTESIAN_POINT('Ctrl Pts',(-3.01681638079674,2.52603162682772,297.707091139139));
#5553=CARTESIAN_POINT('Ctrl Pts',(-3.08881657645025,2.4346870757956,297.71296160328));
#5554=CARTESIAN_POINT('Ctrl Pts',(-3.16312456313294,2.34041469750521,297.71902023086));
#5555=CARTESIAN_POINT('Ctrl Pts',(-3.23308065213613,2.24277823071728,297.72507885844));
#5556=CARTESIAN_POINT('Ctrl Pts',(-3.29838705336314,2.14222590923703,297.73113748602));
#5557=CARTESIAN_POINT('Ctrl Pts',(-3.36175944418768,2.04465138521739,297.737016690932));
#5558=CARTESIAN_POINT('Ctrl Pts',(-3.42075350303013,1.94433166484596,297.742895895844));
#5559=CARTESIAN_POINT('Ctrl Pts',(-3.47514360823768,1.84170190370885,297.748775100755));
#5560=CARTESIAN_POINT('Ctrl Pts',(-3.53202354445589,1.73437403138183,297.75492343967));
#5561=CARTESIAN_POINT('Ctrl Pts',(-3.58386779070879,1.62452006884419,297.761071778584));
#5562=CARTESIAN_POINT('Ctrl Pts',(-3.63047482275331,1.51266042499774,297.767220117498));
#5563=CARTESIAN_POINT('Ctrl Pts',(-3.67708185479782,1.4008007811513,297.773368456412));
#5564=CARTESIAN_POINT('Ctrl Pts',(-3.71845156387867,1.28693595500757,297.779516795327));
#5565=CARTESIAN_POINT('Ctrl Pts',(-3.75444230825449,1.17160230197313,297.785665134241));
#5566=CARTESIAN_POINT('Ctrl Pts',(-3.78884670506842,1.06135215755922,297.791542475636));
#5567=CARTESIAN_POINT('Ctrl Pts',(-3.8184469033587,0.949405204907577,297.797419817031));
#5568=CARTESIAN_POINT('Ctrl Pts',(-3.8430754740714,0.836217615570792,297.803297158426));
#5569=CARTESIAN_POINT('Ctrl Pts',(-3.86767267882028,0.723174177426265,297.809167014673));
#5570=CARTESIAN_POINT('Ctrl Pts',(-3.88731076127924,0.608893644422506,297.815036870921));
#5571=CARTESIAN_POINT('Ctrl Pts',(-3.90187169702593,0.493848417986708,297.820906727169));
#5572=CARTESIAN_POINT('Ctrl Pts',(-3.9164179628193,0.378919098119767,297.826770669612));
#5573=CARTESIAN_POINT('Ctrl Pts',(-3.92589720538806,0.263227024224401,297.832634612056));
#5574=CARTESIAN_POINT('Ctrl Pts',(-3.93024234526173,0.147255246125917,297.8384985545));
#5575=CARTESIAN_POINT('Ctrl Pts',(-3.93467542384946,0.0289363838527769,
297.844481173804));
#5576=CARTESIAN_POINT('Ctrl Pts',(-3.93376423865397,-0.0896732009304856,
297.850463793109));
#5577=CARTESIAN_POINT('Ctrl Pts',(-3.92749315512083,-0.208054119110971,
297.856446412413));
#5578=CARTESIAN_POINT('Ctrl Pts',(-3.92135332922841,-0.323957251762902,
297.86230381181));
#5579=CARTESIAN_POINT('Ctrl Pts',(-3.91007581159166,-0.439640765396489,
297.868161211208));
#5580=CARTESIAN_POINT('Ctrl Pts',(-3.89369855941713,-0.554617461312753,
297.874018610605));
#5581=CARTESIAN_POINT('Ctrl Pts',(-3.87732364307123,-0.669577758515963,
297.879875174583));
#5582=CARTESIAN_POINT('Ctrl Pts',(-3.85585049677704,-0.783831030207,297.88573173856));
#5583=CARTESIAN_POINT('Ctrl Pts',(-3.82936877675414,-0.896896745239102,
297.891588302538));
#5584=CARTESIAN_POINT('Ctrl Pts',(-3.80288445395497,-1.00997357302219,297.897445442133));
#5585=CARTESIAN_POINT('Ctrl Pts',(-3.77139067295981,-1.12186221049407,297.903302581727));
#5586=CARTESIAN_POINT('Ctrl Pts',(-3.73502772160115,-1.23209452513634,297.909159721322));
#5587=CARTESIAN_POINT('Ctrl Pts',(-3.69730099994697,-1.34646103545575,297.915236529362));
#5588=CARTESIAN_POINT('Ctrl Pts',(-3.6543328677155,-1.45904409174705,297.921313337402));
#5589=CARTESIAN_POINT('Ctrl Pts',(-3.6063353876151,-1.56934192323886,297.927390145442));
#5590=CARTESIAN_POINT('Ctrl Pts',(-3.56000478352882,-1.67580928676987,297.93325591562));
#5591=CARTESIAN_POINT('Ctrl Pts',(-3.50898858329163,-1.7801471603624,297.939121685798));
#5592=CARTESIAN_POINT('Ctrl Pts',(-3.45352462110269,-1.88192898150741,297.944987455977));
#5593=CARTESIAN_POINT('Ctrl Pts',(-3.39802257169273,-1.98378069644589,297.950857254192));
#5594=CARTESIAN_POINT('Ctrl Pts',(-3.33806689116138,-2.08307251172606,297.956727052407));
#5595=CARTESIAN_POINT('Ctrl Pts',(-3.27393888723683,-2.17940660791842,297.962596850622));
#5596=CARTESIAN_POINT('Ctrl Pts',(-3.2097214767929,-2.2758750119905,297.968474832442));
#5597=CARTESIAN_POINT('Ctrl Pts',(-3.14132037904824,-2.36937713800281,297.974352814262));
#5598=CARTESIAN_POINT('Ctrl Pts',(-3.06905726829611,-2.45954802431642,297.980230796081));
#5599=CARTESIAN_POINT('Ctrl Pts',(-3.06147350420917,-2.46901114764719,297.980847669988));
#5600=CARTESIAN_POINT('Ctrl Pts',(-3.05384723796947,-2.47843761515068,297.981464543895));
#5601=CARTESIAN_POINT('Ctrl Pts',(-3.04617886433616,-2.48782702904998,297.982081417801));
#5602=CARTESIAN_POINT('Ctrl Pts',(-2.97306131840848,-2.57735460488876,297.987963278591));
#5603=CARTESIAN_POINT('Ctrl Pts',(-2.89587582608214,-2.66380025802543,297.99384513938));
#5604=CARTESIAN_POINT('Ctrl Pts',(-2.8149117811643,-2.74677277259376,297.99972700017));
#5605=CARTESIAN_POINT('Ctrl Pts',(-2.73405011246422,-2.82964037130435,298.005601423551));
#5606=CARTESIAN_POINT('Ctrl Pts',(-2.64941967868757,-2.90904327365463,298.011475846932));
#5607=CARTESIAN_POINT('Ctrl Pts',(-2.56135058815952,-2.98462261676998,298.017350270313));
#5608=CARTESIAN_POINT('Ctrl Pts',(-2.4733695321063,-3.0601264102488,298.02321882158));
#5609=CARTESIAN_POINT('Ctrl Pts',(-2.38195696772714,-3.13181398091997,298.029087372847));
#5610=CARTESIAN_POINT('Ctrl Pts',(-2.28747990829278,-3.19936316618743,298.034955924114));
#5611=CARTESIAN_POINT('Ctrl Pts',(-2.19119404201578,-3.26820561173689,298.040936831499));
#5612=CARTESIAN_POINT('Ctrl Pts',(-2.09172543363303,-3.33274926684149,298.046917738884));
#5613=CARTESIAN_POINT('Ctrl Pts',(-1.98949837687786,-3.3926958614648,298.05289864627));
#5614=CARTESIAN_POINT('Ctrl Pts',(-1.88930232427782,-3.45145146236658,298.058760727503));
#5615=CARTESIAN_POINT('Ctrl Pts',(-1.78645679038421,-3.50579076493241,298.064622808737));
#5616=CARTESIAN_POINT('Ctrl Pts',(-1.68139000228497,-3.55547699475276,298.07048488997));
#5617=CARTESIAN_POINT('Ctrl Pts',(-1.57633784817784,-3.60515630413795,298.076346154717));
#5618=CARTESIAN_POINT('Ctrl Pts',(-1.46906542726807,-3.65018365366576,298.082207419464));
#5619=CARTESIAN_POINT('Ctrl Pts',(-1.36002385382962,-3.69036910308636,298.088068684211));
#5620=CARTESIAN_POINT('Ctrl Pts',(-1.2509713171273,-3.73055859283462,298.093930538261));
#5621=CARTESIAN_POINT('Ctrl Pts',(-1.14014966065168,-3.76590507234974,298.099792392312));
#5622=CARTESIAN_POINT('Ctrl Pts',(-1.02802752287924,-3.79626769501345,298.105654246362));
#5623=CARTESIAN_POINT('Ctrl Pts',(-0.911918583241552,-3.82770994176456,
298.111724534279));
#5624=CARTESIAN_POINT('Ctrl Pts',(-0.794415415532427,-3.85380717801685,
298.117794822195));
#5625=CARTESIAN_POINT('Ctrl Pts',(-0.676051312214117,-3.87446042995067,
298.123865110112));
#5626=CARTESIAN_POINT('Ctrl Pts',(-0.561583339555891,-3.89443384935222,
298.129735585465));
#5627=CARTESIAN_POINT('Ctrl Pts',(-0.446310640159776,-3.90931604677284,
298.135606060819));
#5628=CARTESIAN_POINT('Ctrl Pts',(-0.330720874565897,-3.91907038762082,
298.141476536172));
#5629=CARTESIAN_POINT('Ctrl Pts',(-0.209229639513829,-3.92932273920792,
298.14764673037));
#5630=CARTESIAN_POINT('Ctrl Pts',(-0.0873886365315712,-3.93390978520482,
298.153816924568));
#5631=CARTESIAN_POINT('Ctrl Pts',(0.0342372277062223,-3.9328509776292,298.159987118767));
#5632=CARTESIAN_POINT('Ctrl Pts',(0.155863091944016,-3.93179217005359,298.166157312965));
#5633=CARTESIAN_POINT('Ctrl Pts',(0.2772733014266,-3.9250876078748,298.172327507163));
#5634=CARTESIAN_POINT('Ctrl Pts',(0.397912027585362,-3.91281931838194,298.178497701361));
#5635=CARTESIAN_POINT('Ctrl Pts',(0.51292160164584,-3.9011234824431,298.18437998667));
#5636=CARTESIAN_POINT('Ctrl Pts',(0.627599782461963,-3.88433385978971,298.190262271979));
#5637=CARTESIAN_POINT('Ctrl Pts',(0.741460574344983,-3.86247656519648,298.196144557288));
#5638=CARTESIAN_POINT('Ctrl Pts',(0.855177758129014,-3.84064683834166,298.202019423505));
#5639=CARTESIAN_POINT('Ctrl Pts',(0.968079202550166,-3.81376222860767,298.207894289721));
#5640=CARTESIAN_POINT('Ctrl Pts',(1.0796834978317,-3.78190065238498,298.213769155937));
#5641=CARTESIAN_POINT('Ctrl Pts',(1.19117657663295,-3.75007082702236,298.219638167701));
#5642=CARTESIAN_POINT('Ctrl Pts',(1.30137468405352,-3.71327401370545,298.225507179466));
#5643=CARTESIAN_POINT('Ctrl Pts',(1.40980672183624,-3.67163914445107,298.23137619123));
#5644=CARTESIAN_POINT('Ctrl Pts',(1.52030300364343,-3.629211663236,298.237356932634));
#5645=CARTESIAN_POINT('Ctrl Pts',(1.6289648586505,-3.58176011558691,298.243337674038));
#5646=CARTESIAN_POINT('Ctrl Pts',(1.73530974020645,-3.52947433841707,298.249318415442));
#5647=CARTESIAN_POINT('Ctrl Pts',(1.83955361368677,-3.47822154787025,298.255180998023));
#5648=CARTESIAN_POINT('Ctrl Pts',(1.94157083928183,-3.42232398115469,298.261043580604));
#5649=CARTESIAN_POINT('Ctrl Pts',(2.04092787734249,-3.36200868521875,298.266906163185));
#5650=CARTESIAN_POINT('Ctrl Pts',(2.14027132221888,-3.30170164110822,298.272767943698));
#5651=CARTESIAN_POINT('Ctrl Pts',(2.23695495152024,-3.23697828332267,298.278629724211));
#5652=CARTESIAN_POINT('Ctrl Pts',(2.33057171244451,-3.16811055570248,298.284491504723));
#5653=CARTESIAN_POINT('Ctrl Pts',(2.42419810691866,-3.09923574130976,298.290353888437));
#5654=CARTESIAN_POINT('Ctrl Pts',(2.51475667401381,-3.02621595322321,298.296216272151));
#5655=CARTESIAN_POINT('Ctrl Pts',(2.60187168643205,-2.94936480065509,298.302078655865));
#5656=CARTESIAN_POINT('Ctrl Pts',(2.69206609233749,-2.8697970676477,298.30814826662));
#5657=CARTESIAN_POINT('Ctrl Pts',(2.7785686291232,-2.78612240259129,298.314217877374));
#5658=CARTESIAN_POINT('Ctrl Pts',(2.86100312929294,-2.69873120080085,298.320287488129));
#5659=CARTESIAN_POINT('Ctrl Pts',(2.94074067128642,-2.61419912250503,298.326158523211));
#5660=CARTESIAN_POINT('Ctrl Pts',(3.01667197149979,-2.5261902455251,298.332029558292));
#5661=CARTESIAN_POINT('Ctrl Pts',(3.08849779704574,-2.43509144749096,298.337900593374));
#5662=CARTESIAN_POINT('Ctrl Pts',(3.16396766357847,-2.33937080555374,298.344069491965));
#5663=CARTESIAN_POINT('Ctrl Pts',(3.23490424229983,-2.24023891656768,298.350238390556));
#5664=CARTESIAN_POINT('Ctrl Pts',(3.30101281914729,-2.13817758098462,298.356407289148));
#5665=CARTESIAN_POINT('Ctrl Pts',(3.36712139599475,-2.03611624540157,298.362576187739));
#5666=CARTESIAN_POINT('Ctrl Pts',(3.42840176972213,-1.9311259475968,298.36874508633));
#5667=CARTESIAN_POINT('Ctrl Pts',(3.48461638307562,-1.82371534588077,298.374913984921));
#5668=CARTESIAN_POINT('Ctrl Pts',(3.54119133411491,-1.71561623835913,298.381122426373));
#5669=CARTESIAN_POINT('Ctrl Pts',(3.59280149957876,-1.60475036607249,298.387330867826));
#5670=CARTESIAN_POINT('Ctrl Pts',(3.63918375830147,-1.49158659598255,298.393539309278));
#5671=CARTESIAN_POINT('Ctrl Pts',(3.68730664204182,-1.37417603639303,298.399980739998));
#5672=CARTESIAN_POINT('Ctrl Pts',(3.72980133461905,-1.25429201603047,298.406422170718));
#5673=CARTESIAN_POINT('Ctrl Pts',(3.76642526142513,-1.13248830020386,298.412863601439));
#5674=CARTESIAN_POINT('Ctrl Pts',(3.80157304731997,-1.01559392817932,298.419045407912));
#5675=CARTESIAN_POINT('Ctrl Pts',(3.83131393489967,-0.896931964919147,298.425227214386));
#5676=CARTESIAN_POINT('Ctrl Pts',(3.85548160318599,-0.777013904312119,298.431409020859));
#5677=CARTESIAN_POINT('Ctrl Pts',(3.87961344366601,-0.657273618449312,298.437581662999));
#5678=CARTESIAN_POINT('Ctrl Pts',(3.8981884529318,-0.536281279144689,298.44375430514));
#5679=CARTESIAN_POINT('Ctrl Pts',(3.91109020884378,-0.414562876155478,298.44992694728));
#5680=CARTESIAN_POINT('Ctrl Pts',(3.92396831058168,-0.293067632580642,298.456088272453));
#5681=CARTESIAN_POINT('Ctrl Pts',(3.93119385558125,-0.170849319328,298.462249597626));
#5682=CARTESIAN_POINT('Ctrl Pts',(3.93270165298957,-0.0484428382023322,
298.468410922799));
#5683=CARTESIAN_POINT('Ctrl Pts',(3.93289951333215,-0.0323800779427963,
298.469219441173));
#5684=CARTESIAN_POINT('Ctrl Pts',(3.93299898690451,-0.0163140899041396,
298.470027959547));
#5685=CARTESIAN_POINT('Ctrl Pts',(3.93299999230081,-0.000246093130890435,
298.470836477922));
#5686=CARTESIAN_POINT('',(3.93299898658193,0.00282339255091959,299.720836477927));
#5687=CARTESIAN_POINT('Ctrl Pts',(3.93299999230086,-0.000246092268270265,
298.470836477965));
#5688=CARTESIAN_POINT('Ctrl Pts',(3.93300758397887,0.121082666815665,298.476941565764));
#5689=CARTESIAN_POINT('Ctrl Pts',(3.92739656637158,0.242318400603063,298.483046653563));
#5690=CARTESIAN_POINT('Ctrl Pts',(3.91621860102681,0.362933697762562,298.489151741363));
#5691=CARTESIAN_POINT('Ctrl Pts',(3.90502744511325,0.483691327119881,298.495264033477));
#5692=CARTESIAN_POINT('Ctrl Pts',(3.88825627369643,0.603826702702683,298.501376325591));
#5693=CARTESIAN_POINT('Ctrl Pts',(3.8660081877617,0.722820650064391,298.507488617705));
#5694=CARTESIAN_POINT('Ctrl Pts',(3.84371180437189,0.842072916494249,298.513614178742));
#5695=CARTESIAN_POINT('Ctrl Pts',(3.81591481002405,0.960178448721801,298.51973973978));
#5696=CARTESIAN_POINT('Ctrl Pts',(3.78277103273396,1.0766300729168,298.525865300818));
#5697=CARTESIAN_POINT('Ctrl Pts',(3.74958808912236,1.19321930912004,298.53199810049));
#5698=CARTESIAN_POINT('Ctrl Pts',(3.71104587195854,1.30815039850082,298.538130900162));
#5699=CARTESIAN_POINT('Ctrl Pts',(3.66734688988072,1.42093482935785,298.544263699834));
#5700=CARTESIAN_POINT('Ctrl Pts',(3.62355526516608,1.53395836525966,298.550409501154));
#5701=CARTESIAN_POINT('Ctrl Pts',(3.57458516905893,1.64482581782616,298.556555302473));
#5702=CARTESIAN_POINT('Ctrl Pts',(3.52068620194426,1.75307092481716,298.562701103792));
#5703=CARTESIAN_POINT('Ctrl Pts',(3.49546014165026,1.8037323334055,298.565577492022));
#5704=CARTESIAN_POINT('Ctrl Pts',(3.46915506050871,1.85381971458082,298.568453880252));
#5705=CARTESIAN_POINT('Ctrl Pts',(3.441799798319,1.90328745813429,298.571330268483));
#5706=CARTESIAN_POINT('Ctrl Pts',(3.38586408220222,2.00443851423291,298.577211873066));
#5707=CARTESIAN_POINT('Ctrl Pts',(3.3253754113875,2.10328456294611,298.58309347765));
#5708=CARTESIAN_POINT('Ctrl Pts',(3.26054858194923,2.19938899350453,298.588975082234));
#5709=CARTESIAN_POINT('Ctrl Pts',(3.19580367793401,2.29537197132188,298.594849253893));
#5710=CARTESIAN_POINT('Ctrl Pts',(3.1267317472171,2.38861988338595,298.600723425552));
#5711=CARTESIAN_POINT('Ctrl Pts',(3.05359342725983,2.4787206742583,298.606597597212));
#5712=CARTESIAN_POINT('Ctrl Pts',(2.98052816033606,2.56873146940617,298.612465901549));
#5713=CARTESIAN_POINT('Ctrl Pts',(2.90340484192547,2.65560107857684,298.618334205886));
#5714=CARTESIAN_POINT('Ctrl Pts',(2.82252697930556,2.73894696025538,298.624202510223));
#5715=CARTESIAN_POINT('Ctrl Pts',(2.74009590391267,2.82389345159158,298.630183511966));
#5716=CARTESIAN_POINT('Ctrl Pts',(2.65376483056407,2.90517911534441,298.636164513708));
#5717=CARTESIAN_POINT('Ctrl Pts',(2.56389795662498,2.98243462091196,298.642145515451));
#5718=CARTESIAN_POINT('Ctrl Pts',(2.47582141525793,3.05815103824905,298.648007363363));
#5719=CARTESIAN_POINT('Ctrl Pts',(2.38434897673669,3.1299961093033,298.653869211275));
#5720=CARTESIAN_POINT('Ctrl Pts',(2.28985963840239,3.19766036914737,298.659731059188));
#5721=CARTESIAN_POINT('Ctrl Pts',(2.19538337205763,3.26531526807821,298.665592096151));
#5722=CARTESIAN_POINT('Ctrl Pts',(2.09789137063639,3.32879026634996,298.671453133115));
#5723=CARTESIAN_POINT('Ctrl Pts',(1.99779351867686,3.38781789013706,298.677314170078));
#5724=CARTESIAN_POINT('Ctrl Pts',(1.89768550270672,3.44685150763315,298.683175802176));
#5725=CARTESIAN_POINT('Ctrl Pts',(1.79497146490819,3.50143664374584,298.689037434273));
#5726=CARTESIAN_POINT('Ctrl Pts',(1.69008730354519,3.55135099735232,298.694899066371));
#5727=CARTESIAN_POINT('Ctrl Pts',(1.58146358301208,3.60304500649806,298.700969690177));
#5728=CARTESIAN_POINT('Ctrl Pts',(1.47051253188316,3.64972874368019,298.707040313983));
#5729=CARTESIAN_POINT('Ctrl Pts',(1.35774128006391,3.69120950589511,298.713110937788));
#5730=CARTESIAN_POINT('Ctrl Pts',(1.24869190767526,3.73132124548092,298.718981207962));
#5731=CARTESIAN_POINT('Ctrl Pts',(1.13794100334679,3.76656795945754,298.724851478137));
#5732=CARTESIAN_POINT('Ctrl Pts',(1.02596180108698,3.79682648835977,298.730721748311));
#5733=CARTESIAN_POINT('Ctrl Pts',(0.908249786059665,3.82863411278434,298.736892548932));
#5734=CARTESIAN_POINT('Ctrl Pts',(0.78918089541764,3.85492917728933,298.743063349554));
#5735=CARTESIAN_POINT('Ctrl Pts',(0.669314601046263,3.87562987975197,298.749234150176));
#5736=CARTESIAN_POINT('Ctrl Pts',(0.549448306674884,3.89633058221461,298.755404950798));
#5737=CARTESIAN_POINT('Ctrl Pts',(0.428785134362634,3.91143692789991,298.76157575142));
#5738=CARTESIAN_POINT('Ctrl Pts',(0.307886798785825,3.92093033846987,298.767746552042));
#5739=CARTESIAN_POINT('Ctrl Pts',(0.192654567450534,3.92997882435463,298.773628147693));
#5740=CARTESIAN_POINT('Ctrl Pts',(0.0768375326098742,3.93395774820178,298.779509743344));
#5741=CARTESIAN_POINT('Ctrl Pts',(-0.0390815948845062,3.93280582141317,
298.785391338996));
#5742=CARTESIAN_POINT('Ctrl Pts',(-0.154854251100143,3.93165535015819,298.791265502873));
#5743=CARTESIAN_POINT('Ctrl Pts',(-0.270728335181155,3.9253869263451,298.797139666749));
#5744=CARTESIAN_POINT('Ctrl Pts',(-0.38621637316139,3.91399104663029,298.803013830626));
#5745=CARTESIAN_POINT('Ctrl Pts',(-0.501589080330269,3.90260654728072,298.808882128336));
#5746=CARTESIAN_POINT('Ctrl Pts',(-0.61657610078503,3.88610481820368,298.814750426046));
#5747=CARTESIAN_POINT('Ctrl Pts',(-0.730690972785378,3.86452839325706,298.820618723756));
#5748=CARTESIAN_POINT('Ctrl Pts',(-0.84699754327141,3.84253756993226,298.826599728416));
#5749=CARTESIAN_POINT('Ctrl Pts',(-0.962397683703614,3.81527511216226,298.832580733076));
#5750=CARTESIAN_POINT('Ctrl Pts',(-1.07638251898232,3.78284148132449,298.838561737737));
#5751=CARTESIAN_POINT('Ctrl Pts',(-1.18809641723311,3.75105403059515,298.844423581941));
#5752=CARTESIAN_POINT('Ctrl Pts',(-1.2984504695073,3.71429967000211,298.850285426145));
#5753=CARTESIAN_POINT('Ctrl Pts',(-1.40697760964053,3.67272419410582,298.856147270349));
#5754=CARTESIAN_POINT('Ctrl Pts',(-1.51548975614759,3.63115446209205,298.862008304707));
#5755=CARTESIAN_POINT('Ctrl Pts',(-1.6221751080147,3.58476508665275,298.867869339065));
#5756=CARTESIAN_POINT('Ctrl Pts',(-1.72658462582728,3.53375077359127,298.873730373423));
#5757=CARTESIAN_POINT('Ctrl Pts',(-1.83100476525738,3.48273127082551,298.879592004027));
#5758=CARTESIAN_POINT('Ctrl Pts',(-1.93314824039184,3.42708607590499,298.88545363463));
#5759=CARTESIAN_POINT('Ctrl Pts',(-2.03258937874266,3.36705649156983,298.891315265233));
#5760=CARTESIAN_POINT('Ctrl Pts',(-2.13557615571801,3.3048865132653,298.897385896097));
#5761=CARTESIAN_POINT('Ctrl Pts',(-2.23566388252832,3.23801389735006,298.903456526961));
#5762=CARTESIAN_POINT('Ctrl Pts',(-2.33241234216944,3.1667557004126,298.909527157825));
#5763=CARTESIAN_POINT('Ctrl Pts',(-2.42596764758634,3.09784935913677,298.915397429318));
#5764=CARTESIAN_POINT('Ctrl Pts',(-2.5164003444594,3.02484266972502,298.92126770081));
#5765=CARTESIAN_POINT('Ctrl Pts',(-2.60334692919883,2.94806271409395,298.927137972303));
#5766=CARTESIAN_POINT('Ctrl Pts',(-2.69474489998909,2.86735187118878,298.933308782853));
#5767=CARTESIAN_POINT('Ctrl Pts',(-2.78228997575694,2.78247154699177,298.939479593403));
#5768=CARTESIAN_POINT('Ctrl Pts',(-2.86560565489064,2.6938435794713,298.945650403953));
#5769=CARTESIAN_POINT('Ctrl Pts',(-2.94892133402435,2.60521561195084,298.951821214503));
#5770=CARTESIAN_POINT('Ctrl Pts',(-3.0280073312464,2.51284044281146,298.957992025052));
#5771=CARTESIAN_POINT('Ctrl Pts',(-3.10253867309009,2.41717661373355,298.964162835602));
#5772=CARTESIAN_POINT('Ctrl Pts',(-3.17357549142453,2.32599813929206,298.970044317636));
#5773=CARTESIAN_POINT('Ctrl Pts',(-3.24070398890551,2.23153863094175,298.97592579967));
#5774=CARTESIAN_POINT('Ctrl Pts',(-3.30360706473768,2.13416713539856,298.981807281704));
#5775=CARTESIAN_POINT('Ctrl Pts',(-3.36643063552401,2.03691871054967,298.98768132996));
#5776=CARTESIAN_POINT('Ctrl Pts',(-3.42503918482522,1.9367659614758,298.993555378216));
#5777=CARTESIAN_POINT('Ctrl Pts',(-3.47915620275512,1.83411044292065,298.999429426472));
#5778=CARTESIAN_POINT('Ctrl Pts',(-3.53321915928189,1.73155747438737,299.005297606716));
#5779=CARTESIAN_POINT('Ctrl Pts',(-3.58279931910324,1.62650707216866,299.011165786961));
#5780=CARTESIAN_POINT('Ctrl Pts',(-3.62766415580198,1.51938861806633,299.017033967205));
#5781=CARTESIAN_POINT('Ctrl Pts',(-3.67339191646354,1.41020986267446,299.023015015203));
#5782=CARTESIAN_POINT('Ctrl Pts',(-3.71422085474296,1.29888304458287,299.028996063201));
#5783=CARTESIAN_POINT('Ctrl Pts',(-3.74995442141005,1.18588820609162,299.0349771112));
#5784=CARTESIAN_POINT('Ctrl Pts',(-3.78497508459818,1.07514767415239,299.04083883414));
#5785=CARTESIAN_POINT('Ctrl Pts',(-3.81510167315239,0.962805470956686,299.04670055708));
#5786=CARTESIAN_POINT('Ctrl Pts',(-3.84019852157032,0.84933168722775,299.05256228002));
#5787=CARTESIAN_POINT('Ctrl Pts',(-3.8652918974921,0.735873604166504,299.058423191909));
#5788=CARTESIAN_POINT('Ctrl Pts',(-3.88535682837333,0.621284653934497,299.064284103799));
#5789=CARTESIAN_POINT('Ctrl Pts',(-3.90030839852345,0.506046832227465,299.070145015688));
#5790=CARTESIAN_POINT('Ctrl Pts',(-3.91526148700582,0.390797308117357,299.076006522753));
#5791=CARTESIAN_POINT('Ctrl Pts',(-3.92510012951962,0.274899189935423,299.081868029819));
#5792=CARTESIAN_POINT('Ctrl Pts',(-3.92979117117279,0.158840646474369,299.087729536884));
#5793=CARTESIAN_POINT('Ctrl Pts',(-3.93464971154881,0.0386381070220402,
299.093800335407));
#5794=CARTESIAN_POINT('Ctrl Pts',(-3.93398615723645,-0.0817360519541535,
299.09987113393));
#5795=CARTESIAN_POINT('Ctrl Pts',(-3.92782256344909,-0.20173970868475,299.105941932454));
#5796=CARTESIAN_POINT('Ctrl Pts',(-3.9218626888408,-0.317777003049758,299.111812078868));
#5797=CARTESIAN_POINT('Ctrl Pts',(-3.91076070600483,-0.433467489394996,
299.117682225282));
#5798=CARTESIAN_POINT('Ctrl Pts',(-3.89458930067724,-0.548327620178241,
299.123552371697));
#5799=CARTESIAN_POINT('Ctrl Pts',(-3.87758874399137,-0.669076938173299,
299.129723496275));
#5800=CARTESIAN_POINT('Ctrl Pts',(-3.85498523900164,-0.78890797412956,299.135894620852));
#5801=CARTESIAN_POINT('Ctrl Pts',(-3.8269234206086,-0.90727401197069,299.14206574543));
#5802=CARTESIAN_POINT('Ctrl Pts',(-3.79886160221556,-1.02564004981182,299.148236870008));
#5803=CARTESIAN_POINT('Ctrl Pts',(-3.76534168195458,-1.14254060791152,299.154407994585));
#5804=CARTESIAN_POINT('Ctrl Pts',(-3.72656733161276,-1.25745175770545,299.160579119163));
#5805=CARTESIAN_POINT('Ctrl Pts',(-3.68961247851761,-1.36697066962001,299.166460661992));
#5806=CARTESIAN_POINT('Ctrl Pts',(-3.64776609054497,-1.47503554147972,299.172342204821));
#5807=CARTESIAN_POINT('Ctrl Pts',(-3.60116145735301,-1.58117840804735,299.17822374765));
#5808=CARTESIAN_POINT('Ctrl Pts',(-3.55461572231055,-1.68718713305017,299.184097857484));
#5809=CARTESIAN_POINT('Ctrl Pts',(-3.50332386589151,-1.79127830985841,299.189971967319));
#5810=CARTESIAN_POINT('Ctrl Pts',(-3.44746867013671,-1.89299993883407,299.195846077153));
#5811=CARTESIAN_POINT('Ctrl Pts',(-3.3916692649337,-1.9946199639082,299.201714319676));
#5812=CARTESIAN_POINT('Ctrl Pts',(-3.33131578465535,-2.09387479039293,299.207582562199));
#5813=CARTESIAN_POINT('Ctrl Pts',(-3.26663846632172,-2.19033379427595,299.213450804722));
#5814=CARTESIAN_POINT('Ctrl Pts',(-3.20071810754434,-2.28864665428782,299.219431829638));
#5815=CARTESIAN_POINT('Ctrl Pts',(-3.1303061674118,-2.38405471685387,299.225412854555));
#5816=CARTESIAN_POINT('Ctrl Pts',(-3.05569496974759,-2.4761294901235,299.231393879472));
#5817=CARTESIAN_POINT('Ctrl Pts',(-2.98257122919138,-2.56636865050586,299.237255666013));
#5818=CARTESIAN_POINT('Ctrl Pts',(-2.90541438526128,-2.65340586242024,299.243117452554));
#5819=CARTESIAN_POINT('Ctrl Pts',(-2.82454201203783,-2.73686890848525,299.248979239095));
#5820=CARTESIAN_POINT('Ctrl Pts',(-2.74368082326022,-2.82032041182091,299.254840214965));
#5821=CARTESIAN_POINT('Ctrl Pts',(-2.65910541356834,-2.90019843665227,299.260701190836));
#5822=CARTESIAN_POINT('Ctrl Pts',(-2.57117125235045,-2.97616655970169,299.266562166706));
#5823=CARTESIAN_POINT('Ctrl Pts',(-2.48322815688645,-3.05214240122933,299.272423738061));
#5824=CARTESIAN_POINT('Ctrl Pts',(-2.39192594313031,-3.1242072820544,299.278285309416));
#5825=CARTESIAN_POINT('Ctrl Pts',(-2.29765374936215,-3.19206457454138,299.284146880771));
#5826=CARTESIAN_POINT('Ctrl Pts',(-2.20001795681944,-3.26234299139951,299.290217590933));
#5827=CARTESIAN_POINT('Ctrl Pts',(-2.09919667553962,-3.32810768099155,299.296288301096));
#5828=CARTESIAN_POINT('Ctrl Pts',(-1.99565445230437,-3.38907838608046,299.302359011259));
#5829=CARTESIAN_POINT('Ctrl Pts',(-1.89553195112258,-3.44803539223291,299.308229222139));
#5830=CARTESIAN_POINT('Ctrl Pts',(-1.79286579947545,-3.5025099374884,299.31409943302));
#5831=CARTESIAN_POINT('Ctrl Pts',(-1.68809959077946,-3.55229626743185,299.319969643901));
#5832=CARTESIAN_POINT('Ctrl Pts',(-1.5779658876126,-3.60463330388669,299.326140603704));
#5833=CARTESIAN_POINT('Ctrl Pts',(-1.46551173200654,-3.65178881422318,299.332311563508));
#5834=CARTESIAN_POINT('Ctrl Pts',(-1.35127301478791,-3.69358230441749,299.338482523312));
#5835=CARTESIAN_POINT('Ctrl Pts',(-1.23703429756927,-3.73537579461179,299.344653483115));
#5836=CARTESIAN_POINT('Ctrl Pts',(-1.12101153710817,-3.77180717586096,299.350824442919));
#5837=CARTESIAN_POINT('Ctrl Pts',(-1.00375413201564,-3.80275776804959,299.356995402723));
#5838=CARTESIAN_POINT('Ctrl Pts',(-0.891996200935767,-3.83225675061678,
299.362876939159));
#5839=CARTESIAN_POINT('Ctrl Pts',(-0.778756740685876,-3.85687246497439,
299.368758475595));
#5840=CARTESIAN_POINT('Ctrl Pts',(-0.664499721401675,-3.876458321749,299.374640012031));
#5841=CARTESIAN_POINT('Ctrl Pts',(-0.55038709765623,-3.89601942634332,299.380514115509));
#5842=CARTESIAN_POINT('Ctrl Pts',(-0.435259874857216,-3.910563246732,299.386388218987));
#5843=CARTESIAN_POINT('Ctrl Pts',(-0.319595967014109,-3.91999329308971,
299.392262322465));
#5844=CARTESIAN_POINT('Ctrl Pts',(-0.204047588459498,-3.92941392037654,
299.398130558676));
#5845=CARTESIAN_POINT('Ctrl Pts',(-0.0879639993725192,-3.9337309011422,
299.403998794888));
#5846=CARTESIAN_POINT('Ctrl Pts',(0.0281685797596234,-3.93289912546894,
299.409867031099));
#5847=CARTESIAN_POINT('Ctrl Pts',(0.14653329806966,-3.93205136255866,299.415848058398));
#5848=CARTESIAN_POINT('Ctrl Pts',(0.264948480771353,-3.92585479993738,299.421829085698));
#5849=CARTESIAN_POINT('Ctrl Pts',(0.38289547787891,-3.91431731634264,299.427810112997));
#5850=CARTESIAN_POINT('Ctrl Pts',(0.4984909030979,-3.90300986168253,299.43367189338));
#5851=CARTESIAN_POINT('Ctrl Pts',(0.613636210696612,-3.88657252532392,299.439533673764));
#5852=CARTESIAN_POINT('Ctrl Pts',(0.727845804577129,-3.86506526267791,299.445395454147));
#5853=CARTESIAN_POINT('Ctrl Pts',(0.842039604886268,-3.84356097418211,299.451256423929));
#5854=CARTESIAN_POINT('Ctrl Pts',(0.955297544220685,-3.81698822986422,299.457117393711));
#5855=CARTESIAN_POINT('Ctrl Pts',(1.06714301972724,-3.78545833096171,299.462978363493));
#5856=CARTESIAN_POINT('Ctrl Pts',(1.17899986037524,-3.75392522815882,299.468839928835));
#5857=CARTESIAN_POINT('Ctrl Pts',(1.28944355551657,-3.71743408115245,299.474701494178));
#5858=CARTESIAN_POINT('Ctrl Pts',(1.39801216353395,-3.67614621453107,299.48056305952));
#5859=CARTESIAN_POINT('Ctrl Pts',(1.51045473847569,-3.63338510594234,299.486633778417));
#5860=CARTESIAN_POINT('Ctrl Pts',(1.62088546594619,-3.58547873579373,299.492704497314));
#5861=CARTESIAN_POINT('Ctrl Pts',(1.72881451645822,-3.53266038102778,299.498775216211));
#5862=CARTESIAN_POINT('Ctrl Pts',(1.83317870714832,-3.48158659855142,299.504645421328));
#5863=CARTESIAN_POINT('Ctrl Pts',(1.93520353290518,-3.42592044474168,299.510515626445));
#5864=CARTESIAN_POINT('Ctrl Pts',(2.03447288757065,-3.36591875566538,299.516385831562));
#5865=CARTESIAN_POINT('Ctrl Pts',(2.13882848874925,-3.30284277057018,299.522556807349));
#5866=CARTESIAN_POINT('Ctrl Pts',(2.24013833689055,-3.23497549954912,299.528727783136));
#5867=CARTESIAN_POINT('Ctrl Pts',(2.33795655109297,-3.16266472538609,299.534898758922));
#5868=CARTESIAN_POINT('Ctrl Pts',(2.43577476529539,-3.09035395122306,299.541069734709));
#5869=CARTESIAN_POINT('Ctrl Pts',(2.53010098584831,-3.01360005760153,299.547240710496));
#5870=CARTESIAN_POINT('Ctrl Pts',(2.6205334766521,-2.93279615686901,299.553411686283));
#5871=CARTESIAN_POINT('Ctrl Pts',(2.70548444373599,-2.85689014731022,299.559208611219));
#5872=CARTESIAN_POINT('Ctrl Pts',(2.78729091307262,-2.77715017311055,299.565005536155));
#5873=CARTESIAN_POINT('Ctrl Pts',(2.86558028352338,-2.69387056828683,299.57080246109));
#5874=CARTESIAN_POINT('Ctrl Pts',(2.94376982409076,-2.61069715659241,299.576591994137));
#5875=CARTESIAN_POINT('Ctrl Pts',(3.01845089177533,-2.52399339245083,299.582381527184));
#5876=CARTESIAN_POINT('Ctrl Pts',(3.08928452069845,-2.43409329118112,299.588171060231));
#5877=CARTESIAN_POINT('Ctrl Pts',(3.16004045061587,-2.3442918033608,299.593954242608));
#5878=CARTESIAN_POINT('Ctrl Pts',(3.22695707589869,-2.25130128503618,299.599737424985));
#5879=CARTESIAN_POINT('Ctrl Pts',(3.28973350510711,-2.15549123528157,299.605520607363));
#5880=CARTESIAN_POINT('Ctrl Pts',(3.35247197808269,-2.05973911473071,299.61130029308));
#5881=CARTESIAN_POINT('Ctrl Pts',(3.41107499672829,-1.96117120427352,299.617079978798));
#5882=CARTESIAN_POINT('Ctrl Pts',(3.46528339540584,-1.86018815970981,299.622859664515));
#5883=CARTESIAN_POINT('Ctrl Pts',(3.51947294369267,-1.75924023091954,299.628637340409));
#5884=CARTESIAN_POINT('Ctrl Pts',(3.56927070893024,-1.65587921137128,299.634415016302));
#5885=CARTESIAN_POINT('Ctrl Pts',(3.61446258141136,-1.55053192407546,299.640192692196));
#5886=CARTESIAN_POINT('Ctrl Pts',(3.65965034692724,-1.44519421057295,299.645969843024));
#5887=CARTESIAN_POINT('Ctrl Pts',(3.70023288587998,-1.33787097926437,299.651746993851));
#5888=CARTESIAN_POINT('Ctrl Pts',(3.73604386178533,-1.22900987091891,299.657524144679));
#5889=CARTESIAN_POINT('Ctrl Pts',(3.77187742242758,-1.12008010765892,299.663304938955));
#5890=CARTESIAN_POINT('Ctrl Pts',(3.80293327544379,-1.00961093401714,299.66908573323));
#5891=CARTESIAN_POINT('Ctrl Pts',(3.82909477244069,-0.898065823682953,299.674866527506));
#5892=CARTESIAN_POINT('Ctrl Pts',(3.85526493282691,-0.786483775144647,299.680649236094));
#5893=CARTESIAN_POINT('Ctrl Pts',(3.87653742847292,-0.673825497608828,299.686431944682));
#5894=CARTESIAN_POINT('Ctrl Pts',(3.89284694541333,-0.560563698063004,299.69221465327));
#5895=CARTESIAN_POINT('Ctrl Pts',(3.90917625425363,-0.447164453232653,299.698004379281));
#5896=CARTESIAN_POINT('Ctrl Pts',(3.92053051365403,-0.333160646533695,299.703794105293));
#5897=CARTESIAN_POINT('Ctrl Pts',(3.92689638714524,-0.219029141042092,299.709583831304));
#5898=CARTESIAN_POINT('Ctrl Pts',(3.93102052731456,-0.145088883348921,299.713334713512));
#5899=CARTESIAN_POINT('Ctrl Pts',(3.9330520506215,-0.071095061957422,299.717085595719));
#5900=CARTESIAN_POINT('Ctrl Pts',(3.93299898658193,0.00282339255091775,
299.720836477927));
#5901=CARTESIAN_POINT('',(3.93299856047831,-0.00336500750684849,300.970836478009));
#5902=CARTESIAN_POINT('Ctrl Pts',(3.93299898658139,0.00282339330360925,
299.720836477965));
#5903=CARTESIAN_POINT('Ctrl Pts',(3.93286227153703,0.193268036719428,299.730500308591));
#5904=CARTESIAN_POINT('Ctrl Pts',(3.91889056996141,0.383215183348325,299.740164139217));
#5905=CARTESIAN_POINT('Ctrl Pts',(3.89131247211491,0.571118415359679,299.749827969843));
#5906=CARTESIAN_POINT('Ctrl Pts',(3.87452808318749,0.685478765531458,299.755709502814));
#5907=CARTESIAN_POINT('Ctrl Pts',(3.85267105367365,0.799282807316514,299.761591035785));
#5908=CARTESIAN_POINT('Ctrl Pts',(3.82578888170836,0.912046288626114,299.767472568755));
#5909=CARTESIAN_POINT('Ctrl Pts',(3.79894068332811,1.02466725988382,299.773346668668));
#5910=CARTESIAN_POINT('Ctrl Pts',(3.76708006784964,1.13624988898569,299.77922076858));
#5911=CARTESIAN_POINT('Ctrl Pts',(3.73030608248496,1.24631678596404,299.785094868492));
#5912=CARTESIAN_POINT('Ctrl Pts',(3.69356882892567,1.35627374229275,299.790963101042));
#5913=CARTESIAN_POINT('Ctrl Pts',(3.65192809800505,1.46471758982599,299.796831333592));
#5914=CARTESIAN_POINT('Ctrl Pts',(3.60553344841376,1.57118348781088,299.802699566141));
#5915=CARTESIAN_POINT('Ctrl Pts',(3.55824702521909,1.67969581740632,299.808680594777));
#5916=CARTESIAN_POINT('Ctrl Pts',(3.50602214080958,1.78615295067061,299.814661623413));
#5917=CARTESIAN_POINT('Ctrl Pts',(3.44906982345746,1.89008104400714,299.820642652049));
#5918=CARTESIAN_POINT('Ctrl Pts',(3.39325304405572,1.99193697769186,299.826504428558));
#5919=CARTESIAN_POINT('Ctrl Pts',(3.33289580751339,2.09136341031837,299.832366205066));
#5920=CARTESIAN_POINT('Ctrl Pts',(3.26824404288429,2.18793735654185,299.838227981575));
#5921=CARTESIAN_POINT('Ctrl Pts',(3.20360121949022,2.28449794674394,299.844088947409));
#5922=CARTESIAN_POINT('Ctrl Pts',(3.13466527817958,2.37820649296099,299.849949913244));
#5923=CARTESIAN_POINT('Ctrl Pts',(3.06172583090244,2.46866845412356,299.855810879078));
#5924=CARTESIAN_POINT('Ctrl Pts',(2.98877897275775,2.55913960649385,299.861672440404));
#5925=CARTESIAN_POINT('Ctrl Pts',(2.9118280585073,2.64636319748854,299.86753400173));
#5926=CARTESIAN_POINT('Ctrl Pts',(2.83120293986401,2.72997782285963,299.873395563056));
#5927=CARTESIAN_POINT('Ctrl Pts',(2.74770080941029,2.81657613704588,299.879466287252));
#5928=CARTESIAN_POINT('Ctrl Pts',(2.66025768621864,2.89930276628044,299.885537011448));
#5929=CARTESIAN_POINT('Ctrl Pts',(2.56928054706066,2.97779893050147,299.891607735643));
#5930=CARTESIAN_POINT('Ctrl Pts',(2.48130849086831,3.05370227318346,299.897477936608));
#5931=CARTESIAN_POINT('Ctrl Pts',(2.39003256428525,3.12565000183945,299.903348137573));
#5932=CARTESIAN_POINT('Ctrl Pts',(2.29585243996787,3.19336038897798,299.909218338538));
#5933=CARTESIAN_POINT('Ctrl Pts',(2.19684659428728,3.26454020731649,299.915389324349));
#5934=CARTESIAN_POINT('Ctrl Pts',(2.09463149365931,3.33103665683795,299.92156031016));
#5935=CARTESIAN_POINT('Ctrl Pts',(1.98970214547334,3.39257636204387,299.92773129597));
#5936=CARTESIAN_POINT('Ctrl Pts',(1.88477279728737,3.45411606724978,299.933902281781));
#5937=CARTESIAN_POINT('Ctrl Pts',(1.77712969571039,3.5106988481097,299.940073267592));
#5938=CARTESIAN_POINT('Ctrl Pts',(1.66729218737897,3.56210973468043,299.946244253403));
#5939=CARTESIAN_POINT('Ctrl Pts',(1.56260667785026,3.61110916063007,299.952125785165));
#5940=CARTESIAN_POINT('Ctrl Pts',(1.45559066607768,3.65556877395938,299.958007316927));
#5941=CARTESIAN_POINT('Ctrl Pts',(1.34667444823225,3.69526141571586,299.963888848689));
#5942=CARTESIAN_POINT('Ctrl Pts',(1.23789587840074,3.73490389402181,299.969762947388));
#5943=CARTESIAN_POINT('Ctrl Pts',(1.12722226223994,3.76979124274595,299.975637046086));
#5944=CARTESIAN_POINT('Ctrl Pts',(1.01510657011407,3.79974310333097,299.981511144785));
#5945=CARTESIAN_POINT('Ctrl Pts',(0.90310286516894,3.82966504638739,299.987379376118));
#5946=CARTESIAN_POINT('Ctrl Pts',(0.789660345262875,3.85466120232658,299.993247607451));
#5947=CARTESIAN_POINT('Ctrl Pts',(0.675249337185439,3.87460028036837,299.999115838784));
#5948=CARTESIAN_POINT('Ctrl Pts',(0.558639147709174,3.8949226226631,300.005096867875));
#5949=CARTESIAN_POINT('Ctrl Pts',(0.441023261512045,3.90999131716783,300.011077896966));
#5950=CARTESIAN_POINT('Ctrl Pts',(0.322913385621832,3.91972141170597,300.017058926056));
#5951=CARTESIAN_POINT('Ctrl Pts',(0.207158464239176,3.92925750104498,300.022920701348));
#5952=CARTESIAN_POINT('Ctrl Pts',(0.0909294984046878,3.93366587279982,300.02878247664));
#5953=CARTESIAN_POINT('Ctrl Pts',(-0.0252850199421676,3.93291872122556,
300.034644251932));
#5954=CARTESIAN_POINT('Ctrl Pts',(-0.14148346604903,3.93217167298091,300.040505216551));
#5955=CARTESIAN_POINT('Ctrl Pts',(-0.257667056951934,3.92627052199484,300.046366181171));
#5956=CARTESIAN_POINT('Ctrl Pts',(-0.373346971543809,3.9152395889446,300.052227145791));
#5957=CARTESIAN_POINT('Ctrl Pts',(-0.489038639637707,3.90420753511125,300.058088705906));
#5958=CARTESIAN_POINT('Ctrl Pts',(-0.604226119740003,3.88804470219206,300.063950266021));
#5959=CARTESIAN_POINT('Ctrl Pts',(-0.718426074681787,3.86682724920798,300.069811826136));
#5960=CARTESIAN_POINT('Ctrl Pts',(-0.836701177368185,3.84485266584044,300.075882552038));
#5961=CARTESIAN_POINT('Ctrl Pts',(-0.953916490971856,3.81745606708775,300.081953277941));
#5962=CARTESIAN_POINT('Ctrl Pts',(-1.06954837563246,3.78477942186621,300.088024003843));
#5963=CARTESIAN_POINT('Ctrl Pts',(-1.18136074768559,3.75318214034061,300.093894203617));
#5964=CARTESIAN_POINT('Ctrl Pts',(-1.29169226784869,3.71664831158494,300.099764403391));
#5965=CARTESIAN_POINT('Ctrl Pts',(-1.40008762459992,3.67535626075108,300.105634603166));
#5966=CARTESIAN_POINT('Ctrl Pts',(-1.51403716230762,3.6319484041367,300.111805592132));
#5967=CARTESIAN_POINT('Ctrl Pts',(-1.62584637717475,3.58328199783452,300.117976581099));
#5968=CARTESIAN_POINT('Ctrl Pts',(-1.73501440219533,3.52961952966248,300.124147570065));
#5969=CARTESIAN_POINT('Ctrl Pts',(-1.84418242721591,3.47595706149044,300.130318559031));
#5970=CARTESIAN_POINT('Ctrl Pts',(-1.95070883988529,3.41729884466421,300.136489547998));
#5971=CARTESIAN_POINT('Ctrl Pts',(-2.05412810537226,3.35395985764883,300.142660536964));
#5972=CARTESIAN_POINT('Ctrl Pts',(-2.15269635935121,3.29359186596465,300.148542067885));
#5973=CARTESIAN_POINT('Ctrl Pts',(-2.24875994987839,3.22877777678703,300.154423598805));
#5974=CARTESIAN_POINT('Ctrl Pts',(-2.34189223289244,3.15975153604173,300.160305129726));
#5975=CARTESIAN_POINT('Ctrl Pts',(-2.4349068152897,3.09081253068729,300.166179227565));
#5976=CARTESIAN_POINT('Ctrl Pts',(-2.5249971300413,3.01767220412538,300.172053325405));
#5977=CARTESIAN_POINT('Ctrl Pts',(-2.61176309751935,2.94060920940477,300.177927423244));
#5978=CARTESIAN_POINT('Ctrl Pts',(-2.69844239822905,2.86362318957311,300.183795653702));
#5979=CARTESIAN_POINT('Ctrl Pts',(-2.7818036509193,2.78272256780388,300.189663884159));
#5980=CARTESIAN_POINT('Ctrl Pts',(-2.86147816243415,2.69822751559473,300.195532114616));
#5981=CARTESIAN_POINT('Ctrl Pts',(-2.94268417509544,2.61210830194591,300.201513144029));
#5982=CARTESIAN_POINT('Ctrl Pts',(-3.02005989979471,2.52225530447395,300.207494173442));
#5983=CARTESIAN_POINT('Ctrl Pts',(-3.09325251614972,2.42904875853356,300.213475202855));
#5984=CARTESIAN_POINT('Ctrl Pts',(-3.16498575366242,2.3377006467889,300.219336977236));
#5985=CARTESIAN_POINT('Ctrl Pts',(-3.23270088533774,2.24313181838456,300.225198751617));
#5986=CARTESIAN_POINT('Ctrl Pts',(-3.29610557226436,2.1457346193059,300.231060525998));
#5987=CARTESIAN_POINT('Ctrl Pts',(-3.35950149032172,2.04835089026149,300.236921489696));
#5988=CARTESIAN_POINT('Ctrl Pts',(-3.41858792455225,1.94813991347986,300.242782453394));
#5989=CARTESIAN_POINT('Ctrl Pts',(-3.47311585622691,1.84552302863584,300.248643417091));
#5990=CARTESIAN_POINT('Ctrl Pts',(-3.52764932804217,1.74289571772297,300.254504976274));
#5991=CARTESIAN_POINT('Ctrl Pts',(-3.57762318335449,1.63786237646624,300.260366535457));
#5992=CARTESIAN_POINT('Ctrl Pts',(-3.62283468592864,1.53086832824783,300.266228094639));
#5993=CARTESIAN_POINT('Ctrl Pts',(-3.6696595473584,1.420056229636,300.272298821796));
#5994=CARTESIAN_POINT('Ctrl Pts',(-3.71137563291121,1.30714131369295,300.278369548953));
#5995=CARTESIAN_POINT('Ctrl Pts',(-3.74781292239943,1.19263879640729,300.28444027611));
#5996=CARTESIAN_POINT('Ctrl Pts',(-3.7830466149001,1.081918527659,300.290310474934));
#5997=CARTESIAN_POINT('Ctrl Pts',(-3.81334469339374,0.969714304558971,300.296180673759));
#5998=CARTESIAN_POINT('Ctrl Pts',(-3.83860512399242,0.856504350286162,300.302050872583));
#5999=CARTESIAN_POINT('Ctrl Pts',(-3.86515991416635,0.737493450231623,300.308221863906));
#6000=CARTESIAN_POINT('Ctrl Pts',(-3.88614702618422,0.617371542083399,300.31439285523));
#6001=CARTESIAN_POINT('Ctrl Pts',(-3.90150956439982,0.496701237059789,300.320563846553));
#6002=CARTESIAN_POINT('Ctrl Pts',(-3.91687210261542,0.376030932036179,300.326734837877));
#6003=CARTESIAN_POINT('Ctrl Pts',(-3.92661009564127,0.254812755301197,300.3329058292));
#6004=CARTESIAN_POINT('Ctrl Pts',(-3.93072991968259,0.133608751629746,300.339076820524));
#6005=CARTESIAN_POINT('Ctrl Pts',(-3.93465649713345,0.0180900054416166,
300.344958352147));
#6006=CARTESIAN_POINT('Ctrl Pts',(-3.9334926897861,-0.0977880713029246,
300.35083988377));
#6007=CARTESIAN_POINT('Ctrl Pts',(-3.92719867588365,-0.213540535116148,
300.356721415393));
#6008=CARTESIAN_POINT('Ctrl Pts',(-3.92091261634664,-0.329146711137223,
300.362595513945));
#6009=CARTESIAN_POINT('Ctrl Pts',(-3.90950926720366,-0.44462718230248,300.368469612497));
#6010=CARTESIAN_POINT('Ctrl Pts',(-3.89300075218217,-0.559494542876913,
300.37434371105));
#6011=CARTESIAN_POINT('Ctrl Pts',(-3.87650872677365,-0.67424716761256,300.380211942229));
#6012=CARTESIAN_POINT('Ctrl Pts',(-3.85492173761455,-0.788387494658678,
300.386080173408));
#6013=CARTESIAN_POINT('Ctrl Pts',(-3.82830384953644,-0.901431437006986,
300.391948404588));
#6014=CARTESIAN_POINT('Ctrl Pts',(-3.80117431773606,-1.01664828741144,300.397929433733));
#6015=CARTESIAN_POINT('Ctrl Pts',(-3.76881850597314,-1.13072573458947,300.403910462879));
#6016=CARTESIAN_POINT('Ctrl Pts',(-3.73135934974289,-1.24315984615268,300.409891492025));
#6017=CARTESIAN_POINT('Ctrl Pts',(-3.69464708088346,-1.35335216621741,300.415753267146));
#6018=CARTESIAN_POINT('Ctrl Pts',(-3.65303322709672,-1.46196566771069,300.421615042267));
#6019=CARTESIAN_POINT('Ctrl Pts',(-3.60668415290106,-1.56854021982619,300.427476817388));
#6020=CARTESIAN_POINT('Ctrl Pts',(-3.56034148873928,-1.67510003278018,300.433337781831));
#6021=CARTESIAN_POINT('Ctrl Pts',(-3.50926507071346,-1.77962107959935,300.439198746275));
#6022=CARTESIAN_POINT('Ctrl Pts',(-3.45366932690097,-1.88166340784515,300.445059710718));
#6023=CARTESIAN_POINT('Ctrl Pts',(-3.39806793441307,-1.98371610386285,300.45092127065));
#6024=CARTESIAN_POINT('Ctrl Pts',(-3.33794650035513,-2.08328921904157,300.456782830583));
#6025=CARTESIAN_POINT('Ctrl Pts',(-3.27356496741808,-2.17996821171618,300.462644390516));
#6026=CARTESIAN_POINT('Ctrl Pts',(-3.206886018671,-2.2800971353902,300.468715116647));
#6027=CARTESIAN_POINT('Ctrl Pts',(-3.1356375157091,-2.37712113013852,300.474785842777));
#6028=CARTESIAN_POINT('Ctrl Pts',(-3.06015575390324,-2.47061445026392,300.480856568908));
#6029=CARTESIAN_POINT('Ctrl Pts',(-2.98716728484268,-2.56101952481547,300.486726768487));
#6030=CARTESIAN_POINT('Ctrl Pts',(-2.91022112759993,-2.64812321743505,300.492596968066));
#6031=CARTESIAN_POINT('Ctrl Pts',(-2.82966016283104,-2.73157690041613,300.498467167645));
#6032=CARTESIAN_POINT('Ctrl Pts',(-2.74497124323042,-2.81930676150501,300.504638157051));
#6033=CARTESIAN_POINT('Ctrl Pts',(-2.65628764242745,-2.90300228752162,300.510809146458));
#6034=CARTESIAN_POINT('Ctrl Pts',(-2.5640475344818,-2.98230602737509,300.516980135864));
#6035=CARTESIAN_POINT('Ctrl Pts',(-2.47180742653616,-3.06160976722855,300.523151125271));
#6036=CARTESIAN_POINT('Ctrl Pts',(-2.37601126548068,-3.13652145545942,300.529322114677));
#6037=CARTESIAN_POINT('Ctrl Pts',(-2.27713161213382,-3.20673675580345,300.535493104084));
#6038=CARTESIAN_POINT('Ctrl Pts',(-2.18289003236026,-3.27365851983395,300.541374635529));
#6039=CARTESIAN_POINT('Ctrl Pts',(-2.08554403724696,-3.33653013104263,300.547256166974));
#6040=CARTESIAN_POINT('Ctrl Pts',(-1.98547639138279,-3.39505117770875,300.553137698419));
#6041=CARTESIAN_POINT('Ctrl Pts',(-1.88553521088857,-3.45349826554679,300.559011796792));
#6042=CARTESIAN_POINT('Ctrl Pts',(-1.78287957293349,-3.50760551789886,300.564885895165));
#6043=CARTESIAN_POINT('Ctrl Pts',(-1.67792291623876,-3.55711451701528,300.570759993538));
#6044=CARTESIAN_POINT('Ctrl Pts',(-1.57307109605039,-3.60657406380857,300.576628224537));
#6045=CARTESIAN_POINT('Ctrl Pts',(-1.46592319957269,-3.65144431931033,300.582496455535));
#6046=CARTESIAN_POINT('Ctrl Pts',(-1.35691851279621,-3.69151204110605,300.588364686534));
#6047=CARTESIAN_POINT('Ctrl Pts',(-1.24581855506076,-3.73234993835341,300.594345715747));
#6048=CARTESIAN_POINT('Ctrl Pts',(-1.13279006261636,-3.7681985473478,300.60032674496));
#6049=CARTESIAN_POINT('Ctrl Pts',(-1.01832131796954,-3.79888282174757,300.606307774173));
#6050=CARTESIAN_POINT('Ctrl Pts',(-0.906134937533447,-3.82895528992951,
300.612169549112));
#6051=CARTESIAN_POINT('Ctrl Pts',(-0.792565622134735,-3.85406734576189,
300.618031324051));
#6052=CARTESIAN_POINT('Ctrl Pts',(-0.678089027239685,-3.8741043185667,300.62389309899));
#6053=CARTESIAN_POINT('Ctrl Pts',(-0.563628264357405,-3.89413852027572,
300.629754063251));
#6054=CARTESIAN_POINT('Ctrl Pts',(-0.448260877046215,-3.90909896380426,
300.635615027512));
#6055=CARTESIAN_POINT('Ctrl Pts',(-0.332472161681067,-3.9189222066414,300.641475991772));
#6056=CARTESIAN_POINT('Ctrl Pts',(-0.216671681875719,-3.92874644754604,
300.647337551523));
#6057=CARTESIAN_POINT('Ctrl Pts',(-0.100450199251126,-3.93343241534619,
300.653199111273));
#6058=CARTESIAN_POINT('Ctrl Pts',(0.0157031198949376,-3.93296865128945,
300.659060671023));
#6059=CARTESIAN_POINT('Ctrl Pts',(0.136001308312363,-3.93248833805958,300.665131397408));
#6060=CARTESIAN_POINT('Ctrl Pts',(0.256225900979215,-3.92648389608274,300.671202123793));
#6061=CARTESIAN_POINT('Ctrl Pts',(0.375836314881207,-3.91500141307976,300.677272850178));
#6062=CARTESIAN_POINT('Ctrl Pts',(0.491495782155133,-3.90389821709722,300.683143049576));
#6063=CARTESIAN_POINT('Ctrl Pts',(0.60658059924388,-3.88767328386297,300.689013248974));
#6064=CARTESIAN_POINT('Ctrl Pts',(0.720610913084401,-3.8664206848122,300.694883448372));
#6065=CARTESIAN_POINT('Ctrl Pts',(0.840484168638869,-3.84407909728687,300.701054438251));
#6066=CARTESIAN_POINT('Ctrl Pts',(0.959191476895999,-3.81618107976652,300.707225428129));
#6067=CARTESIAN_POINT('Ctrl Pts',(1.07619311940487,-3.78289536859607,300.713396418008));
#6068=CARTESIAN_POINT('Ctrl Pts',(1.19319476191375,-3.74960965742562,300.719567407887));
#6069=CARTESIAN_POINT('Ctrl Pts',(1.30849026698904,-3.71093648525897,300.725738397765));
#6070=CARTESIAN_POINT('Ctrl Pts',(1.4215652972654,-3.66710254909932,300.731909387644));
#6071=CARTESIAN_POINT('Ctrl Pts',(1.52933639269463,-3.62532470207726,300.737790919026));
#6072=CARTESIAN_POINT('Ctrl Pts',(1.63543784988561,-3.57872467304876,300.743672450408));
#6073=CARTESIAN_POINT('Ctrl Pts',(1.73940807989206,-3.52745638266531,300.74955398179));
#6074=CARTESIAN_POINT('Ctrl Pts',(1.84324691241889,-3.47625288509938,300.755428080099));
#6075=CARTESIAN_POINT('Ctrl Pts',(1.94495950844811,-3.42039304042143,300.761302178407));
#6076=CARTESIAN_POINT('Ctrl Pts',(2.04410242477976,-3.36007950456675,300.767176276715));
#6077=CARTESIAN_POINT('Ctrl Pts',(2.14314631166475,-3.29982621321871,300.773044507648));
#6078=CARTESIAN_POINT('Ctrl Pts',(2.23962527491145,-3.23512829293464,300.778912738581));
#6079=CARTESIAN_POINT('Ctrl Pts',(2.33311933139266,-3.16623485949509,300.784780969514));
#6080=CARTESIAN_POINT('Ctrl Pts',(2.42841051739046,-3.09601716623204,300.790761998751));
#6081=CARTESIAN_POINT('Ctrl Pts',(2.5206004700145,-3.02144119401526,300.796743027988));
#6082=CARTESIAN_POINT('Ctrl Pts',(2.60927408768007,-2.94281799222469,300.802724057225));
#6083=CARTESIAN_POINT('Ctrl Pts',(2.69617966246681,-2.86576244038114,300.808585832095));
#6084=CARTESIAN_POINT('Ctrl Pts',(2.77970750466545,-2.78481984323551,300.814447606965));
#6085=CARTESIAN_POINT('Ctrl Pts',(2.85949985541869,-2.70032397627776,300.820309381835));
#6086=CARTESIAN_POINT('Ctrl Pts',(2.93928117094525,-2.6158397950397,300.826170346026));
#6087=CARTESIAN_POINT('Ctrl Pts',(3.01532773975615,-2.52780362059282,300.832031310217));
#6088=CARTESIAN_POINT('Ctrl Pts',(3.08731924326377,-2.43658549822764,300.837892274407));
#6089=CARTESIAN_POINT('Ctrl Pts',(3.1593180612869,-2.34535810787473,300.843753834086));
#6090=CARTESIAN_POINT('Ctrl Pts',(3.22726073984971,-2.25094845018128,300.849615393766));
#6091=CARTESIAN_POINT('Ctrl Pts',(3.29086821072129,-2.1537584404162,300.855476953445));
#6092=CARTESIAN_POINT('Ctrl Pts',(3.35674548210995,-2.05310025417129,300.861547679925));
#6093=CARTESIAN_POINT('Ctrl Pts',(3.41797210376408,-1.94945997571898,300.867618406405));
#6094=CARTESIAN_POINT('Ctrl Pts',(3.47428870425617,-1.84331413477952,300.873689132885));
#6095=CARTESIAN_POINT('Ctrl Pts',(3.52874506483896,-1.740674484338,300.87955933221));
#6096=CARTESIAN_POINT('Ctrl Pts',(3.57861053221662,-1.63569258843833,300.885429531534));
#6097=CARTESIAN_POINT('Ctrl Pts',(3.62369923835292,-1.52882073179313,300.891299730859));
#6098=CARTESIAN_POINT('Ctrl Pts',(3.67109830299598,-1.41647272991574,300.897470720917));
#6099=CARTESIAN_POINT('Ctrl Pts',(3.71321793158873,-1.30203644970569,300.903641710975));
#6100=CARTESIAN_POINT('Ctrl Pts',(3.74990158412522,-1.18605527247898,300.909812701032));
#6101=CARTESIAN_POINT('Ctrl Pts',(3.7865852366617,-1.07007409525226,300.91598369109));
#6102=CARTESIAN_POINT('Ctrl Pts',(3.81783284742637,-0.952548542829235,300.922154681147));
#6103=CARTESIAN_POINT('Ctrl Pts',(3.8435502305382,-0.8340327483557,300.928325671204));
#6104=CARTESIAN_POINT('Ctrl Pts',(3.87699876730369,-0.679888763662496,300.93635178284));
#6105=CARTESIAN_POINT('Ctrl Pts',(3.90118402329849,-0.523669741101071,300.944377894475));
#6106=CARTESIAN_POINT('Ctrl Pts',(3.91590394367339,-0.366313122783201,300.95240400611));
#6107=CARTESIAN_POINT('Ctrl Pts',(3.92717235235256,-0.245853321478743,300.958548163395));
#6108=CARTESIAN_POINT('Ctrl Pts',(3.93289472509772,-0.124727083469295,300.96469232068));
#6109=CARTESIAN_POINT('Ctrl Pts',(3.93299856047757,-0.00336500837822571,
300.970836477965));
#6110=CARTESIAN_POINT('',(3.93299968132247,0.00158326162505113,302.220836477997));
#6111=CARTESIAN_POINT('Ctrl Pts',(3.93299856047831,-0.00336500750684587,
300.970836478009));
#6112=CARTESIAN_POINT('Ctrl Pts',(3.93309642351835,0.111016667666786,300.976627240917));
#6113=CARTESIAN_POINT('Ctrl Pts',(3.92820031008576,0.225544572613075,300.982418003824));
#6114=CARTESIAN_POINT('Ctrl Pts',(3.91829868241434,0.339741718648166,300.988208766731));
#6115=CARTESIAN_POINT('Ctrl Pts',(3.90840490488755,0.453848327637999,300.993994938643));
#6116=CARTESIAN_POINT('Ctrl Pts',(3.89351354081032,0.567624278283278,300.999781110555));
#6117=CARTESIAN_POINT('Ctrl Pts',(3.87366511651891,0.680593538806071,301.005567282468));
#6118=CARTESIAN_POINT('Ctrl Pts',(3.85382505019857,0.793515229113815,301.011351017881));
#6119=CARTESIAN_POINT('Ctrl Pts',(3.82903214430561,0.905630487192161,301.017134753294));
#6120=CARTESIAN_POINT('Ctrl Pts',(3.79937858655754,1.01647004678349,301.022918488708));
#6121=CARTESIAN_POINT('Ctrl Pts',(3.76972992619471,1.12729130084712,301.028701268918));
#6122=CARTESIAN_POINT('Ctrl Pts',(3.73522231925427,1.23683686558601,301.034484049128));
#6123=CARTESIAN_POINT('Ctrl Pts',(3.69599851630752,1.34465012826855,301.040266829338));
#6124=CARTESIAN_POINT('Ctrl Pts',(3.65677115228748,1.45247317916388,301.046050134559));
#6125=CARTESIAN_POINT('Ctrl Pts',(3.6128268872907,1.55856321718528,301.051833439779));
#6126=CARTESIAN_POINT('Ctrl Pts',(3.56435724870095,1.66248200099521,301.057616745));
#6127=CARTESIAN_POINT('Ctrl Pts',(3.51584124399944,1.76650019363266,301.063405582536));
#6128=CARTESIAN_POINT('Ctrl Pts',(3.46279139982919,1.86834259890711,301.069194420073));
#6129=CARTESIAN_POINT('Ctrl Pts',(3.40544602109028,1.96759406317471,301.07498325761));
#6130=CARTESIAN_POINT('Ctrl Pts',(3.34807292213555,2.06689350466508,301.080774893416));
#6131=CARTESIAN_POINT('Ctrl Pts',(3.28640038253629,2.16359915404018,301.086566529223));
#6132=CARTESIAN_POINT('Ctrl Pts',(3.2207099608377,2.2573250426469,301.092358165029));
#6133=CARTESIAN_POINT('Ctrl Pts',(3.15491554705315,2.35119930525416,301.098158969361));
#6134=CARTESIAN_POINT('Ctrl Pts',(3.08509080472275,2.44208404844958,301.103959773692));
#6135=CARTESIAN_POINT('Ctrl Pts',(3.01155767267647,2.52962633290838,301.109760578024));
#6136=CARTESIAN_POINT('Ctrl Pts',(2.94825452302332,2.60498967158115,301.114754370271));
#6137=CARTESIAN_POINT('Ctrl Pts',(2.88220378713752,2.67787633476089,301.119748162518));
#6138=CARTESIAN_POINT('Ctrl Pts',(2.81363138731921,2.74808431753689,301.124741954765));
#6139=CARTESIAN_POINT('Ctrl Pts',(2.73286897173146,2.83077307128557,301.130623486196));
#6140=CARTESIAN_POINT('Ctrl Pts',(2.64832821169398,2.91003177469155,301.136505017626));
#6141=CARTESIAN_POINT('Ctrl Pts',(2.56033201258128,2.98549643867674,301.142386549057));
#6142=CARTESIAN_POINT('Ctrl Pts',(2.47244702296896,3.06086573050196,301.148260647415));
#6143=CARTESIAN_POINT('Ctrl Pts',(2.38111558943806,3.13245025346527,301.154134745773));
#6144=CARTESIAN_POINT('Ctrl Pts',(2.28669830350379,3.19992185353844,301.16000884413));
#6145=CARTESIAN_POINT('Ctrl Pts',(2.19237532678064,3.26732605924295,301.165877075113));
#6146=CARTESIAN_POINT('Ctrl Pts',(2.0949729623651,3.33062527627382,301.171745306097));
#6147=CARTESIAN_POINT('Ctrl Pts',(1.99488530741401,3.38953117853542,301.17761353708));
#6148=CARTESIAN_POINT('Ctrl Pts',(1.89287378291923,3.4495693610104,301.183594566298));
#6149=CARTESIAN_POINT('Ctrl Pts',(1.78807299843527,3.5050433050812,301.189575595517));
#6150=CARTESIAN_POINT('Ctrl Pts',(1.68093208576008,3.55569350803219,301.195556624735));
#6151=CARTESIAN_POINT('Ctrl Pts',(1.57592742985903,3.60533380882289,301.201418399657));
#6152=CARTESIAN_POINT('Ctrl Pts',(1.46867548891698,3.65034076207192,301.207280174579));
#6153=CARTESIAN_POINT('Ctrl Pts',(1.35962376252546,3.69051652541702,301.213141949501));
#6154=CARTESIAN_POINT('Ctrl Pts',(1.25058711790202,3.73068673248561,301.219002913744));
#6155=CARTESIAN_POINT('Ctrl Pts',(1.1397515691501,3.76602693607731,301.224863877987));
#6156=CARTESIAN_POINT('Ctrl Pts',(1.02758325800001,3.79638797383488,301.23072484223));
#6157=CARTESIAN_POINT('Ctrl Pts',(0.915403550261956,3.82675209635171,301.236586401962));
#6158=CARTESIAN_POINT('Ctrl Pts',(0.801891208440969,3.85213593975959,301.242447961694));
#6159=CARTESIAN_POINT('Ctrl Pts',(0.687525473407211,3.87244079663152,301.248309521426));
#6160=CARTESIAN_POINT('Ctrl Pts',(0.569078657268208,3.89347022164181,301.254380247834));
#6161=CARTESIAN_POINT('Ctrl Pts',(0.449716873291618,3.90905132129816,301.260450974243));
#6162=CARTESIAN_POINT('Ctrl Pts',(0.329980236896991,3.91913281776178,301.266521700651));
#6163=CARTESIAN_POINT('Ctrl Pts',(0.214198717309004,3.92888130423532,301.272391900029));
#6164=CARTESIAN_POINT('Ctrl Pts',(0.0980671387338737,3.93348781893126,301.278262099408));
#6165=CARTESIAN_POINT('Ctrl Pts',(-0.0179255588339876,3.93295914984385,
301.284132298786));
#6166=CARTESIAN_POINT('Ctrl Pts',(-0.139861752426486,3.93240339161475,301.290303288709));
#6167=CARTESIAN_POINT('Ctrl Pts',(-0.261643926493478,3.92617228084719,301.296474278633));
#6168=CARTESIAN_POINT('Ctrl Pts',(-0.382710894131026,3.91433536778767,301.302645268556));
#6169=CARTESIAN_POINT('Ctrl Pts',(-0.503777861768569,3.90249845472815,301.308816258479));
#6170=CARTESIAN_POINT('Ctrl Pts',(-0.624129117302728,3.88505588397538,301.314987248402));
#6171=CARTESIAN_POINT('Ctrl Pts',(-0.74321808634839,3.86213876966178,301.321158238325));
#6172=CARTESIAN_POINT('Ctrl Pts',(-0.856721028788768,3.84029661309866,301.327039769752));
#6173=CARTESIAN_POINT('Ctrl Pts',(-0.96944313299157,3.81341149870345,301.332921301179));
#6174=CARTESIAN_POINT('Ctrl Pts',(-1.08090273155306,3.78155236442934,301.338802832606));
#6175=CARTESIAN_POINT('Ctrl Pts',(-1.19222146759307,3.74973349369506,301.34467693096));
#6176=CARTESIAN_POINT('Ctrl Pts',(-1.30228047876852,3.71295321749393,301.350551029313));
#6177=CARTESIAN_POINT('Ctrl Pts',(-1.41060724030656,3.67133166760982,301.356425127667));
#6178=CARTESIAN_POINT('Ctrl Pts',(-1.51882579907708,3.62975169163434,301.362293358646));
#6179=CARTESIAN_POINT('Ctrl Pts',(-1.62531516790214,3.58334020837589,301.368161589625));
#6180=CARTESIAN_POINT('Ctrl Pts',(-1.72961760009685,3.53226725453146,301.374029820604));
#6181=CARTESIAN_POINT('Ctrl Pts',(-1.83592491773613,3.48021258415732,301.380010849824));
#6182=CARTESIAN_POINT('Ctrl Pts',(-1.93995993808061,3.42331550647589,301.385991879044));
#6183=CARTESIAN_POINT('Ctrl Pts',(-2.04125864743069,3.36180786695038,301.391972908264));
#6184=CARTESIAN_POINT('Ctrl Pts',(-2.14053758618997,3.30152661344913,301.397834683182));
#6185=CARTESIAN_POINT('Ctrl Pts',(-2.23718795307223,3.23681717642505,301.4036964581));
#6186=CARTESIAN_POINT('Ctrl Pts',(-2.33079809162441,3.16794401088151,301.409558233017));
#6187=CARTESIAN_POINT('Ctrl Pts',(-2.4243952839665,3.09908037044373,301.415419197256));
#6188=CARTESIAN_POINT('Ctrl Pts',(-2.51495275253598,3.02605439064379,301.421280161494));
#6189=CARTESIAN_POINT('Ctrl Pts',(-2.60208919539452,2.94917290425826,301.427141125733));
#6190=CARTESIAN_POINT('Ctrl Pts',(-2.68923449153746,2.87228360651801,301.433002685461));
#6191=CARTESIAN_POINT('Ctrl Pts',(-2.77295776220296,2.79153829591929,301.438864245188));
#6192=CARTESIAN_POINT('Ctrl Pts',(-2.8529125951192,2.70728253505433,301.444725804916));
#6193=CARTESIAN_POINT('Ctrl Pts',(-2.93572057434046,2.62002015152481,301.45079653133));
#6194=CARTESIAN_POINT('Ctrl Pts',(-3.01448581251665,2.52899244459817,301.456867257744));
#6195=CARTESIAN_POINT('Ctrl Pts',(-3.08886794048257,2.43462191033001,301.462937984158));
#6196=CARTESIAN_POINT('Ctrl Pts',(-3.16079309263499,2.34336860497887,301.468808183532));
#6197=CARTESIAN_POINT('Ctrl Pts',(-3.22861993213213,2.24899019989031,301.474678382906));
#6198=CARTESIAN_POINT('Ctrl Pts',(-3.29208474305109,2.15189847450344,301.48054858228));
#6199=CARTESIAN_POINT('Ctrl Pts',(-3.35880150757953,2.0498317435623,301.486719572214));
#6200=CARTESIAN_POINT('Ctrl Pts',(-3.42069711094639,1.94476672081401,301.492890562148));
#6201=CARTESIAN_POINT('Ctrl Pts',(-3.47752041045979,1.83721005735207,301.499061552082));
#6202=CARTESIAN_POINT('Ctrl Pts',(-3.53434370997318,1.72965339389013,301.505232542016));
#6203=CARTESIAN_POINT('Ctrl Pts',(-3.58609454770608,1.61960559138573,301.511403531951));
#6204=CARTESIAN_POINT('Ctrl Pts',(-3.6325812091906,1.50759502474482,301.517574521885));
#6205=CARTESIAN_POINT('Ctrl Pts',(-3.67688735191643,1.40083846288577,301.523456053319));
#6206=CARTESIAN_POINT('Ctrl Pts',(-3.71655474682514,1.29195513096818,301.529337584753));
#6207=CARTESIAN_POINT('Ctrl Pts',(-3.75137555139626,1.18138498059965,301.535219116187));
#6208=CARTESIAN_POINT('Ctrl Pts',(-3.78615234947252,1.07095456866658,301.541093214548));
#6209=CARTESIAN_POINT('Ctrl Pts',(-3.81609461649755,0.958841967506965,301.546967312909));
#6210=CARTESIAN_POINT('Ctrl Pts',(-3.84104227032977,0.845507704009778,301.55284141127));
#6211=CARTESIAN_POINT('Ctrl Pts',(-3.86596500506448,0.732286645048134,301.558709642257));
#6212=CARTESIAN_POINT('Ctrl Pts',(-3.8859029627829,0.617846751099631,301.564577873243));
#6213=CARTESIAN_POINT('Ctrl Pts',(-3.90074585091687,0.502663711197483,301.57044610423));
#6214=CARTESIAN_POINT('Ctrl Pts',(-3.91587404675698,0.385266640669798,301.576427133447));
#6215=CARTESIAN_POINT('Ctrl Pts',(-3.92570914490651,0.267097974193734,301.582408162664));
#6216=CARTESIAN_POINT('Ctrl Pts',(-3.93018898183505,0.14867268431816,301.588389191882));
#6217=CARTESIAN_POINT('Ctrl Pts',(-3.93457949638071,0.032608647598457,301.594250966807));
#6218=CARTESIAN_POINT('Ctrl Pts',(-3.93382631025829,-0.0837014439737091,
301.600112741732));
#6219=CARTESIAN_POINT('Ctrl Pts',(-3.92792332002528,-0.19976834584481,301.605974516657));
#6220=CARTESIAN_POINT('Ctrl Pts',(-3.92202114617121,-0.315819195753972,
301.611835480903));
#6221=CARTESIAN_POINT('Ctrl Pts',(-3.9109706054979,-0.431626511680904,301.61769644515));
#6222=CARTESIAN_POINT('Ctrl Pts',(-3.89481768425206,-0.546703033133568,
301.623557409396));
#6223=CARTESIAN_POINT('Ctrl Pts',(-3.87866312182813,-0.661791246654964,
301.629418969131));
#6224=CARTESIAN_POINT('Ctrl Pts',(-3.85740520550711,-0.776148110288028,
301.635280528866));
#6225=CARTESIAN_POINT('Ctrl Pts',(-3.83114146549651,-0.889294142201137,
301.641142088602));
#6226=CARTESIAN_POINT('Ctrl Pts',(-3.80394051777232,-1.00647773060195,301.647212815005));
#6227=CARTESIAN_POINT('Ctrl Pts',(-3.77136991776805,-1.12236199240654,301.653283541409));
#6228=CARTESIAN_POINT('Ctrl Pts',(-3.73359472912333,-1.23643010261903,301.659354267813));
#6229=CARTESIAN_POINT('Ctrl Pts',(-3.69706732296464,-1.34673033779912,301.665224467194));
#6230=CARTESIAN_POINT('Ctrl Pts',(-3.65567393915433,-1.4553321394044,301.671094666576));
#6231=CARTESIAN_POINT('Ctrl Pts',(-3.60961292988756,-1.56178855687592,301.676964865958));
#6232=CARTESIAN_POINT('Ctrl Pts',(-3.56119174260528,-1.67369982868355,301.683135855872));
#6233=CARTESIAN_POINT('Ctrl Pts',(-3.50761215158859,-1.7832395568609,301.689306845787));
#6234=CARTESIAN_POINT('Ctrl Pts',(-3.44915861034888,-1.8899190143115,301.695477835701));
#6235=CARTESIAN_POINT('Ctrl Pts',(-3.39070506910917,-1.9965984717621,301.701648825616));
#6236=CARTESIAN_POINT('Ctrl Pts',(-3.32737790930106,-2.10041725029467,301.707819815531));
#6237=CARTESIAN_POINT('Ctrl Pts',(-3.25951245570123,-2.20092424929359,301.713990805445));
#6238=CARTESIAN_POINT('Ctrl Pts',(-3.19483032139855,-2.29671683392642,301.719872336876));
#6239=CARTESIAN_POINT('Ctrl Pts',(-3.12581760277878,-2.38980994238618,301.725753868308));
#6240=CARTESIAN_POINT('Ctrl Pts',(-3.05272694618447,-2.47978773124621,301.731635399739));
#6241=CARTESIAN_POINT('Ctrl Pts',(-2.97972866148265,-2.56965180627432,301.737509498097));
#6242=CARTESIAN_POINT('Ctrl Pts',(-2.90266294612174,-2.65640807518584,301.743383596455));
#6243=CARTESIAN_POINT('Ctrl Pts',(-2.82182593083418,-2.73966921654272,301.749257694813));
#6244=CARTESIAN_POINT('Ctrl Pts',(-2.74106966003229,-2.82284719206264,301.755125925797));
#6245=CARTESIAN_POINT('Ctrl Pts',(-2.65654986806582,-2.90253669097835,301.76099415678));
#6246=CARTESIAN_POINT('Ctrl Pts',(-2.56860277056359,-2.97838358964272,301.766862387764));
#6247=CARTESIAN_POINT('Ctrl Pts',(-2.47896516745751,-3.05568840574687,301.772843416982));
#6248=CARTESIAN_POINT('Ctrl Pts',(-2.38576741288062,-3.12900103385473,301.778824446201));
#6249=CARTESIAN_POINT('Ctrl Pts',(-2.28940502271977,-3.19798587269323,301.784805475419));
#6250=CARTESIAN_POINT('Ctrl Pts',(-2.19496397897023,-3.26559523950041,301.790667250341));
#6251=CARTESIAN_POINT('Ctrl Pts',(-2.09748367848344,-3.32904754989868,301.796529025264));
#6252=CARTESIAN_POINT('Ctrl Pts',(-1.99736905234712,-3.38806816175914,301.802390800186));
#6253=CARTESIAN_POINT('Ctrl Pts',(-1.89726827198561,-3.44708061111496,301.808251764429));
#6254=CARTESIAN_POINT('Ctrl Pts',(-1.79453424516427,-3.5016623717278,301.814112728672));
#6255=CARTESIAN_POINT('Ctrl Pts',(-1.68959894593133,-3.55158336547345,301.819973692915));
#6256=CARTESIAN_POINT('Ctrl Pts',(-1.58465298500382,-3.60150943131964,301.825835252648));
#6257=CARTESIAN_POINT('Ctrl Pts',(-1.4775056789278,-3.64677361201657,301.83169681238));
#6258=CARTESIAN_POINT('Ctrl Pts',(-1.36861090822361,-3.68719313053864,301.837558372112));
#6259=CARTESIAN_POINT('Ctrl Pts',(-1.25583028490971,-3.72905499831694,301.84362909852));
#6260=CARTESIAN_POINT('Ctrl Pts',(-1.14117559858218,-3.76571981855612,301.849699824928));
#6261=CARTESIAN_POINT('Ctrl Pts',(-1.02516910154362,-3.79704059936686,301.855770551336));
#6262=CARTESIAN_POINT('Ctrl Pts',(-0.912994508079964,-3.82732679836519,
301.861640750714));
#6263=CARTESIAN_POINT('Ctrl Pts',(-0.799556420831486,-3.85261639866851,
301.867510950093));
#6264=CARTESIAN_POINT('Ctrl Pts',(-0.685337119421168,-3.8728286862116,301.873381149471));
#6265=CARTESIAN_POINT('Ctrl Pts',(-0.56526519128116,-3.89407665662863,301.879552139394));
#6266=CARTESIAN_POINT('Ctrl Pts',(-0.444330394377407,-3.90971313830002,
301.885723129316));
#6267=CARTESIAN_POINT('Ctrl Pts',(-0.323097309888554,-3.9197062553644,301.891894119239));
#6268=CARTESIAN_POINT('Ctrl Pts',(-0.201864225399701,-3.92969937242878,
301.898065109161));
#6269=CARTESIAN_POINT('Ctrl Pts',(-0.080333376702017,-3.93404917677253,
301.904236099084));
#6270=CARTESIAN_POINT('Ctrl Pts',(0.0409340283513448,-3.93278697685534,
301.910407089006));
#6271=CARTESIAN_POINT('Ctrl Pts',(0.156513224452326,-3.93158398210432,301.916288620437));
#6272=CARTESIAN_POINT('Ctrl Pts',(0.27222553085449,-3.92527967244625,301.922170151868));
#6273=CARTESIAN_POINT('Ctrl Pts',(0.387584714775992,-3.91385578284024,301.928051683299));
#6274=CARTESIAN_POINT('Ctrl Pts',(0.502798107885911,-3.90244633073353,301.933925781657));
#6275=CARTESIAN_POINT('Ctrl Pts',(0.617658859821588,-3.88593020698826,301.939799880015));
#6276=CARTESIAN_POINT('Ctrl Pts',(0.731680582858796,-3.86434115014027,301.945673978373));
#6277=CARTESIAN_POINT('Ctrl Pts',(0.845588414687085,-3.84277365763737,301.951542209357));
#6278=CARTESIAN_POINT('Ctrl Pts',(0.958658482398417,-3.81614338804519,301.95741044034));
#6279=CARTESIAN_POINT('Ctrl Pts',(1.07041001841268,-3.78453582259195,301.963278671323));
#6280=CARTESIAN_POINT('Ctrl Pts',(1.18430962529593,-3.75232070136803,301.969259700542));
#6281=CARTESIAN_POINT('Ctrl Pts',(1.29683905491361,-3.71493500399106,301.97524072976));
#6282=CARTESIAN_POINT('Ctrl Pts',(1.40750032594332,-3.67252390495548,301.981221758979));
#6283=CARTESIAN_POINT('Ctrl Pts',(1.51595514862774,-3.63095843057627,301.987083533901));
#6284=CARTESIAN_POINT('Ctrl Pts',(1.62261521870239,-3.58456625312263,301.992945308823));
#6285=CARTESIAN_POINT('Ctrl Pts',(1.72702824035086,-3.53353398979416,301.998807083745));
#6286=CARTESIAN_POINT('Ctrl Pts',(1.83142682175967,-3.482508784188,302.004668047988));
#6287=CARTESIAN_POINT('Ctrl Pts',(1.93357860287773,-3.42684494967813,302.010529012231));
#6288=CARTESIAN_POINT('Ctrl Pts',(2.03305357901926,-3.3667762243483,302.016389976474));
#6289=CARTESIAN_POINT('Ctrl Pts',(2.13253866207282,-3.30670139588231,302.022251536206));
#6290=CARTESIAN_POINT('Ctrl Pts',(2.22934604697387,-3.24222099977867,302.028113095938));
#6291=CARTESIAN_POINT('Ctrl Pts',(2.32307313432031,-3.17361311640206,302.03397465567));
#6292=CARTESIAN_POINT('Ctrl Pts',(2.42014482348011,-3.10255699679354,302.040045382078));
#6293=CARTESIAN_POINT('Ctrl Pts',(2.51391188487007,-3.02707359239515,302.046116108486));
#6294=CARTESIAN_POINT('Ctrl Pts',(2.60396391385506,-2.94751775827401,302.052186834894));
#6295=CARTESIAN_POINT('Ctrl Pts',(2.69104136209466,-2.8705897966731,302.058057034272));
#6296=CARTESIAN_POINT('Ctrl Pts',(2.77464507276988,-2.78985453124993,302.063927233651));
#6297=CARTESIAN_POINT('Ctrl Pts',(2.8544419755787,-2.70566997397213,302.069797433029));
#6298=CARTESIAN_POINT('Ctrl Pts',(2.93832769246227,-2.61717177806229,302.075968422952));
#6299=CARTESIAN_POINT('Ctrl Pts',(3.0180057981482,-2.52486184285586,302.082139412875));
#6300=CARTESIAN_POINT('Ctrl Pts',(3.09313863581024,-2.42919377153367,302.088310402798));
#6301=CARTESIAN_POINT('Ctrl Pts',(3.16827147347228,-2.33352570021148,302.09448139272));
#6302=CARTESIAN_POINT('Ctrl Pts',(3.23885879805826,-2.23449995813827,302.100652382643));
#6303=CARTESIAN_POINT('Ctrl Pts',(3.30461754106501,-2.13260214463116,302.106823372566));
#6304=CARTESIAN_POINT('Ctrl Pts',(3.36854554677612,-2.03354118777613,302.112822560826));
#6305=CARTESIAN_POINT('Ctrl Pts',(3.42811017090977,-1.93145696754079,302.118821749086));
#6306=CARTESIAN_POINT('Ctrl Pts',(3.48302060674435,-1.82676119210864,302.124820937346));
#6307=CARTESIAN_POINT('Ctrl Pts',(3.5378536738083,-1.72221293296029,302.130811672753));
#6308=CARTESIAN_POINT('Ctrl Pts',(3.58804542311245,-1.6150607833623,302.13680240816));
#6309=CARTESIAN_POINT('Ctrl Pts',(3.63334843404784,-1.50574505039935,302.142793143567));
#6310=CARTESIAN_POINT('Ctrl Pts',(3.67859675921488,-1.39656127367341,302.148776647491));
#6311=CARTESIAN_POINT('Ctrl Pts',(3.71896794345594,-1.28521946973946,302.154760151415));
#6312=CARTESIAN_POINT('Ctrl Pts',(3.75426080001111,-1.17218379339589,302.160743655339));
#6313=CARTESIAN_POINT('Ctrl Pts',(3.78951057542934,-1.05928609697023,302.166719855345));
#6314=CARTESIAN_POINT('Ctrl Pts',(3.81969425795302,-0.944699018097502,302.17269605535));
#6315=CARTESIAN_POINT('Ctrl Pts',(3.84465930220239,-0.828905211703131,302.178672255355));
#6316=CARTESIAN_POINT('Ctrl Pts',(3.86960642744596,-0.71319451791486,302.18464416586));
#6317=CARTESIAN_POINT('Ctrl Pts',(3.88934228772551,-0.596279200328868,302.190616076365));
#6318=CARTESIAN_POINT('Ctrl Pts',(3.90376457098115,-0.478655590537035,302.19658798687));
#6319=CARTESIAN_POINT('Ctrl Pts',(3.91817850501867,-0.36110007434428,302.202556440171));
#6320=CARTESIAN_POINT('Ctrl Pts',(3.92728494152255,-0.242837468855173,302.208524893471));
#6321=CARTESIAN_POINT('Ctrl Pts',(3.93103301119697,-0.124372283406156,302.214493346772));
#6322=CARTESIAN_POINT('Ctrl Pts',(3.9323607978372,-0.0824049497558171,302.216607723836));
#6323=CARTESIAN_POINT('Ctrl Pts',(3.93301658695605,-0.0404122476420527,
302.218722100901));
#6324=CARTESIAN_POINT('Ctrl Pts',(3.93299968132272,0.00158326098779867,
302.220836477965));
#6325=CARTESIAN_POINT('',(3.93299980390471,0.00124196841146249,303.470836477931));
#6326=CARTESIAN_POINT('Ctrl Pts',(3.93299968132247,0.00158326162505384,
302.220836477997));
#6327=CARTESIAN_POINT('Ctrl Pts',(3.93294868380391,0.128266824884077,302.227214703415));
#6328=CARTESIAN_POINT('Ctrl Pts',(3.92677272985102,0.254761136096585,302.233592928833));
#6329=CARTESIAN_POINT('Ctrl Pts',(3.91455140815298,0.380494773850481,302.239971154252));
#6330=CARTESIAN_POINT('Ctrl Pts',(3.90227516682082,0.5067934278565,302.246378041856));
#6331=CARTESIAN_POINT('Ctrl Pts',(3.88389919273337,0.632324281556489,302.252784929461));
#6332=CARTESIAN_POINT('Ctrl Pts',(3.85955466376678,0.756522833360689,302.259191817066));
#6333=CARTESIAN_POINT('Ctrl Pts',(3.83515314991891,0.881012105093762,302.265613701705));
#6334=CARTESIAN_POINT('Ctrl Pts',(3.80475523229135,1.00416257072053,302.272035586344));
#6335=CARTESIAN_POINT('Ctrl Pts',(3.7685419950764,1.1254244671881,302.278457470983));
#6336=CARTESIAN_POINT('Ctrl Pts',(3.73221410263239,1.24707029261601,302.284899688039));
#6337=CARTESIAN_POINT('Ctrl Pts',(3.69003414469865,1.36681531903206,302.291341905096));
#6338=CARTESIAN_POINT('Ctrl Pts',(3.64223220348205,1.4841272101536,302.297784122152));
#6339=CARTESIAN_POINT('Ctrl Pts',(3.6287386544955,1.51724205254839,302.299602633477));
#6340=CARTESIAN_POINT('Ctrl Pts',(3.61479741450538,1.55016316822392,302.301421144801));
#6341=CARTESIAN_POINT('Ctrl Pts',(3.60041431324821,1.58287895082266,302.303239656125));
#6342=CARTESIAN_POINT('Ctrl Pts',(3.55389567958219,1.68869017182401,302.309121187556));
#6343=CARTESIAN_POINT('Ctrl Pts',(3.50263369698545,1.79261943292796,302.315002718987));
#6344=CARTESIAN_POINT('Ctrl Pts',(3.44680261578071,1.8942124294406,302.320884250418));
#6345=CARTESIAN_POINT('Ctrl Pts',(3.39104209383576,1.99567703283458,302.326758348776));
#6346=CARTESIAN_POINT('Ctrl Pts',(3.33072415434759,2.09481088605764,302.332632447134));
#6347=CARTESIAN_POINT('Ctrl Pts',(3.26607092977507,2.19117997473467,302.338506545492));
#6348=CARTESIAN_POINT('Ctrl Pts',(3.20148228442225,2.28745280463124,302.344374776475));
#6349=CARTESIAN_POINT('Ctrl Pts',(3.13256719626738,2.38096602345876,302.350243007459));
#6350=CARTESIAN_POINT('Ctrl Pts',(3.0595931709049,2.47131111528924,302.356111238442));
#6351=CARTESIAN_POINT('Ctrl Pts',(2.98521645002923,2.56339280660589,302.362092267661));
#6352=CARTESIAN_POINT('Ctrl Pts',(2.90662334810156,2.65218293684626,302.368073296879));
#6353=CARTESIAN_POINT('Ctrl Pts',(2.82414302670637,2.73728061489972,302.374054326098));
#6354=CARTESIAN_POINT('Ctrl Pts',(2.74330726051104,2.82068155091131,302.37991610102));
#6355=CARTESIAN_POINT('Ctrl Pts',(2.65873815131185,2.90053560808156,302.385777875942));
#6356=CARTESIAN_POINT('Ctrl Pts',(2.57078502006563,2.97650018992207,302.391639650864));
#6357=CARTESIAN_POINT('Ctrl Pts',(2.48284405266891,3.05245426592013,302.397500615107));
#6358=CARTESIAN_POINT('Ctrl Pts',(2.39152030552604,3.12451966722851,302.40336157935));
#6359=CARTESIAN_POINT('Ctrl Pts',(2.29719767240265,3.19239281008898,302.409222543593));
#6360=CARTESIAN_POINT('Ctrl Pts',(2.20286545585876,3.26027284903418,302.415084103325));
#6361=CARTESIAN_POINT('Ctrl Pts',(2.10553408188791,3.32395954225861,302.420945663057));
#6362=CARTESIAN_POINT('Ctrl Pts',(2.00561745251773,3.38319192984322,302.426807222789));
#6363=CARTESIAN_POINT('Ctrl Pts',(1.90213535078178,3.44453799402423,302.432877949197));
#6364=CARTESIAN_POINT('Ctrl Pts',(1.79588044885773,3.50110566993879,302.438948675605));
#6365=CARTESIAN_POINT('Ctrl Pts',(1.68734031573658,3.5526569858192,302.445019402014));
#6366=CARTESIAN_POINT('Ctrl Pts',(1.58238545874658,3.60250546886682,302.450889601392));
#6367=CARTESIAN_POINT('Ctrl Pts',(1.47529436655552,3.64766365189985,302.45675980077));
#6368=CARTESIAN_POINT('Ctrl Pts',(1.36652712562125,3.68796591835409,302.462630000149));
#6369=CARTESIAN_POINT('Ctrl Pts',(1.25218662294444,3.73033328343396,302.468800990072));
#6370=CARTESIAN_POINT('Ctrl Pts',(1.13599415365427,3.76733375293837,302.474971979995));
#6371=CARTESIAN_POINT('Ctrl Pts',(1.01849950972216,3.7988350515251,302.481142969918));
#6372=CARTESIAN_POINT('Ctrl Pts',(0.901004865790038,3.83033635011184,302.487313959841));
#6373=CARTESIAN_POINT('Ctrl Pts',(0.782208571438175,3.85633843528387,302.493484949763));
#6374=CARTESIAN_POINT('Ctrl Pts',(0.662668393150532,3.87677180147598,302.499655939686));
#6375=CARTESIAN_POINT('Ctrl Pts',(0.548735405950958,3.89624671344413,302.505537471118));
#6376=CARTESIAN_POINT('Ctrl Pts',(0.433759646994256,3.91072625163266,302.511419002549));
#6377=CARTESIAN_POINT('Ctrl Pts',(0.318216254326758,3.92010553626841,302.51730053398));
#6378=CARTESIAN_POINT('Ctrl Pts',(0.202818885273631,3.92947296737441,302.523174632338));
#6379=CARTESIAN_POINT('Ctrl Pts',(0.0868557161750379,3.93375293139621,302.529048730696));
#6380=CARTESIAN_POINT('Ctrl Pts',(-0.0291886673971811,3.93289168700278,
302.534922829054));
#6381=CARTESIAN_POINT('Ctrl Pts',(-0.145117139415065,3.93203130286793,302.540791060038));
#6382=CARTESIAN_POINT('Ctrl Pts',(-0.261126255042839,3.92603992884984,302.546659291022));
#6383=CARTESIAN_POINT('Ctrl Pts',(-0.376727709900703,3.91491573761083,302.552527522005));
#6384=CARTESIAN_POINT('Ctrl Pts',(-0.494551238172591,3.90357771887601,302.558508551223));
#6385=CARTESIAN_POINT('Ctrl Pts',(-0.611950838548064,3.88690748403242,302.564489580442));
#6386=CARTESIAN_POINT('Ctrl Pts',(-0.728410600579572,3.86495886096648,302.57047060966));
#6387=CARTESIAN_POINT('Ctrl Pts',(-0.84254829955899,3.84344786619186,302.576332384582));
#6388=CARTESIAN_POINT('Ctrl Pts',(-0.955782868850262,3.81686710255979,302.582194159504));
#6389=CARTESIAN_POINT('Ctrl Pts',(-1.06763594037816,3.78531933907997,302.588055934427));
#6390=CARTESIAN_POINT('Ctrl Pts',(-1.17947354271327,3.75377593863131,302.59391689867));
#6391=CARTESIAN_POINT('Ctrl Pts',(-1.2899296310067,3.71726701619518,302.599777862913));
#6392=CARTESIAN_POINT('Ctrl Pts',(-1.39853934699871,3.67594568715268,302.605638827156));
#6393=CARTESIAN_POINT('Ctrl Pts',(-1.50716009801522,3.63462015975763,302.611500386888));
#6394=CARTESIAN_POINT('Ctrl Pts',(-1.61393371891148,3.58848140019214,302.617361946621));
#6395=CARTESIAN_POINT('Ctrl Pts',(-1.71841438968569,3.53773105045044,302.623223506353));
#6396=CARTESIAN_POINT('Ctrl Pts',(-1.8266233982354,3.48516970117496,302.62929423276));
#6397=CARTESIAN_POINT('Ctrl Pts',(-1.93237232452447,3.42766169539494,302.635364959168));
#6398=CARTESIAN_POINT('Ctrl Pts',(-2.03519394636018,3.36548281836334,302.641435685576));
#6399=CARTESIAN_POINT('Ctrl Pts',(-2.13461918480063,3.30535782165104,302.647305884955));
#6400=CARTESIAN_POINT('Ctrl Pts',(-2.23130713953885,3.24086593897765,302.653176084333));
#6401=CARTESIAN_POINT('Ctrl Pts',(-2.32486611309871,3.17229988433712,302.659046283712));
#6402=CARTESIAN_POINT('Ctrl Pts',(-2.42321907281232,3.10022048721262,302.665217273634));
#6403=CARTESIAN_POINT('Ctrl Pts',(-2.5181134859288,3.02363866808636,302.671388263556));
#6404=CARTESIAN_POINT('Ctrl Pts',(-2.60913605640904,2.94294037301918,302.677559253479));
#6405=CARTESIAN_POINT('Ctrl Pts',(-2.70015862688927,2.86224207795201,302.683730243401));
#6406=CARTESIAN_POINT('Ctrl Pts',(-2.78730903044837,2.77742772101423,302.689901233324));
#6407=CARTESIAN_POINT('Ctrl Pts',(-2.87022196134231,2.68892448622647,302.696072223246));
#6408=CARTESIAN_POINT('Ctrl Pts',(-2.94924575095883,2.60457261335401,302.70195375468));
#6409=CARTESIAN_POINT('Ctrl Pts',(-3.02467521876955,2.51659831271189,302.707835286115));
#6410=CARTESIAN_POINT('Ctrl Pts',(-3.09616106188238,2.42534032228126,302.713716817549));
#6411=CARTESIAN_POINT('Ctrl Pts',(-3.16755656126438,2.33419766359975,302.71959091591));
#6412=CARTESIAN_POINT('Ctrl Pts',(-3.23501809650283,2.23977989008139,302.725465014271));
#6413=CARTESIAN_POINT('Ctrl Pts',(-3.29823383664126,2.14246179868736,302.731339112632));
#6414=CARTESIAN_POINT('Ctrl Pts',(-3.36138643339906,2.04524091399017,302.737207343619));
#6415=CARTESIAN_POINT('Ctrl Pts',(-3.42030144830607,1.94512581771063,302.743075574605));
#6416=CARTESIAN_POINT('Ctrl Pts',(-3.47470832579785,1.84252301223922,302.748943805592));
#6417=CARTESIAN_POINT('Ctrl Pts',(-3.53016100389512,1.73794799147018,302.754924834809));
#6418=CARTESIAN_POINT('Ctrl Pts',(-3.58093017604073,1.63078897854424,302.760905864027));
#6419=CARTESIAN_POINT('Ctrl Pts',(-3.62677652361598,1.5215061773611,302.766886893244));
#6420=CARTESIAN_POINT('Ctrl Pts',(-3.6717087519777,1.41440233946629,302.772748668169));
#6421=CARTESIAN_POINT('Ctrl Pts',(-3.71191248138543,1.30525901703019,302.778610443094));
#6422=CARTESIAN_POINT('Ctrl Pts',(-3.74720992042188,1.19453204741096,302.78447221802));
#6423=CARTESIAN_POINT('Ctrl Pts',(-3.78250247784995,1.08382039124556,302.790333182266));
#6424=CARTESIAN_POINT('Ctrl Pts',(-3.81288996927061,0.97152591570686,302.796194146512));
#6425=CARTESIAN_POINT('Ctrl Pts',(-3.83824406250132,0.858120921941285,302.802055110759));
#6426=CARTESIAN_POINT('Ctrl Pts',(-3.86360073177262,0.744704405938851,302.807916670494));
#6427=CARTESIAN_POINT('Ctrl Pts',(-3.88392289636919,0.630177549295771,302.813778230229));
#6428=CARTESIAN_POINT('Ctrl Pts',(-3.89913321057087,0.515023500651496,302.819639789964));
#6429=CARTESIAN_POINT('Ctrl Pts',(-3.91488629681441,0.395760240502265,302.825710516368));
#6430=CARTESIAN_POINT('Ctrl Pts',(-3.92515582547606,0.275824662378546,302.831781242771));
#6431=CARTESIAN_POINT('Ctrl Pts',(-3.92991453478782,0.155758625004988,302.837851969175));
#6432=CARTESIAN_POINT('Ctrl Pts',(-3.93451605536408,0.0396585849962591,
302.843722168557));
#6433=CARTESIAN_POINT('Ctrl Pts',(-3.9339651358796,-0.0765630137847103,
302.849592367938));
#6434=CARTESIAN_POINT('Ctrl Pts',(-3.92829025249607,-0.192418014084886,
302.85546256732));
#6435=CARTESIAN_POINT('Ctrl Pts',(-3.92232458662173,-0.314209454534326,
302.861633557234));
#6436=CARTESIAN_POINT('Ctrl Pts',(-3.9106959918333,-0.435595204961309,302.867804547149));
#6437=CARTESIAN_POINT('Ctrl Pts',(-3.89349885041236,-0.55601771719759,302.873975537064));
#6438=CARTESIAN_POINT('Ctrl Pts',(-3.87630170899142,-0.676440229433871,
302.880146526978));
#6439=CARTESIAN_POINT('Ctrl Pts',(-3.8535361878316,-0.795899004719565,302.886317516893));
#6440=CARTESIAN_POINT('Ctrl Pts',(-3.82535752409154,-0.913853824676704,
302.892488506807));
#6441=CARTESIAN_POINT('Ctrl Pts',(-3.7985006180461,-1.02627581694782,302.898370038234));
#6442=CARTESIAN_POINT('Ctrl Pts',(-3.76664036763767,-1.13769397793619,302.90425156966));
#6443=CARTESIAN_POINT('Ctrl Pts',(-3.7298670150836,-1.24763017348545,302.910133101087));
#6444=CARTESIAN_POINT('Ctrl Pts',(-3.69314013665257,-1.35742743179014,302.91600719944));
#6445=CARTESIAN_POINT('Ctrl Pts',(-3.65151263467761,-1.46574606241026,302.921881297793));
#6446=CARTESIAN_POINT('Ctrl Pts',(-3.60512548911715,-1.57211933634754,302.927755396147));
#6447=CARTESIAN_POINT('Ctrl Pts',(-3.55878467760544,-1.67838635877052,302.933623627126));
#6448=CARTESIAN_POINT('Ctrl Pts',(-3.50769384352709,-1.78271151453597,302.939491858104));
#6449=CARTESIAN_POINT('Ctrl Pts',(-3.45204316688148,-1.88464505251968,302.945360089083));
#6450=CARTESIAN_POINT('Ctrl Pts',(-3.39532278141245,-1.98853794143234,302.951341118303));
#6451=CARTESIAN_POINT('Ctrl Pts',(-3.33386558241127,-2.08994590758986,302.957322147524));
#6452=CARTESIAN_POINT('Ctrl Pts',(-3.26792377584389,-2.18841568155463,302.963303176744));
#6453=CARTESIAN_POINT('Ctrl Pts',(-3.20329676709277,-2.28492209038707,302.969164951661));
#6454=CARTESIAN_POINT('Ctrl Pts',(-3.13436256896134,-2.37860603237821,302.975026726579));
#6455=CARTESIAN_POINT('Ctrl Pts',(-3.06140364168512,-2.46906799069549,302.980888501496));
#6456=CARTESIAN_POINT('Ctrl Pts',(-2.98845480457132,-2.5595174381949,302.986749465735));
#6457=CARTESIAN_POINT('Ctrl Pts',(-2.91148260371394,-2.64674546771949,302.992610429974));
#6458=CARTESIAN_POINT('Ctrl Pts',(-2.83081048851824,-2.73038476740827,302.998471394212));
#6459=CARTESIAN_POINT('Ctrl Pts',(-2.75013017682898,-2.81403256506416,303.00433295394));
#6460=CARTESIAN_POINT('Ctrl Pts',(-2.66574948938785,-2.89409061163836,303.010194513667));
#6461=CARTESIAN_POINT('Ctrl Pts',(-2.57802901917495,-2.97022816906241,303.016056073395));
#6462=CARTESIAN_POINT('Ctrl Pts',(-2.48717828995853,-3.04908265531795,303.022126799809));
#6463=CARTESIAN_POINT('Ctrl Pts',(-2.39274532702639,-3.12373131025878,303.028197526224));
#6464=CARTESIAN_POINT('Ctrl Pts',(-2.29516731291136,-3.1938528466013,303.034268252638));
#6465=CARTESIAN_POINT('Ctrl Pts',(-2.20081247655511,-3.26165814215536,303.040138452012));
#6466=CARTESIAN_POINT('Ctrl Pts',(-2.10351746537417,-3.32523049700737,303.046008651386));
#6467=CARTESIAN_POINT('Ctrl Pts',(-2.00370535464323,-3.38432472611214,303.05187885076));
#6468=CARTESIAN_POINT('Ctrl Pts',(-1.89877884509945,-3.44644695906301,303.058049840695));
#6469=CARTESIAN_POINT('Ctrl Pts',(-1.79107091742452,-3.50361974134971,303.064220830629));
#6470=CARTESIAN_POINT('Ctrl Pts',(-1.68109886722032,-3.55561465834398,303.070391820564));
#6471=CARTESIAN_POINT('Ctrl Pts',(-1.57112681701613,-3.60760957533824,303.076562810498));
#6472=CARTESIAN_POINT('Ctrl Pts',(-1.45889115246716,-3.65442649152831,303.082733800432));
#6473=CARTESIAN_POINT('Ctrl Pts',(-1.34492823469066,-3.69589732589149,303.088904790367));
#6474=CARTESIAN_POINT('Ctrl Pts',(-1.23631089938228,-3.73542291552563,303.094786321798));
#6475=CARTESIAN_POINT('Ctrl Pts',(-1.12577471544002,-3.77021995865531,303.100667853229));
#6476=CARTESIAN_POINT('Ctrl Pts',(-1.01376842338987,-3.80010033864076,303.106549384661));
#6477=CARTESIAN_POINT('Ctrl Pts',(-0.9019036847711,-3.82994295583413,303.112423483019));
#6478=CARTESIAN_POINT('Ctrl Pts',(-0.788572927624629,-3.85488116269695,
303.118297581377));
#6479=CARTESIAN_POINT('Ctrl Pts',(-0.674243328308384,-3.87477546887967,
303.124171679735));
#6480=CARTESIAN_POINT('Ctrl Pts',(-0.560027927725882,-3.8946499035279,303.130039910718));
#6481=CARTESIAN_POINT('Ctrl Pts',(-0.444816073096787,-3.90949038943808,
303.135908141702));
#6482=CARTESIAN_POINT('Ctrl Pts',(-0.32908787876733,-3.91920784955945,303.141776372685));
#6483=CARTESIAN_POINT('Ctrl Pts',(-0.211135174855228,-3.92911209720727,
303.147757401904));
#6484=CARTESIAN_POINT('Ctrl Pts',(-0.0926464960115012,-3.93369422362778,
303.153738431122));
#6485=CARTESIAN_POINT('Ctrl Pts',(0.0258609341336898,-3.93291497646284,
303.15971946034));
#6486=CARTESIAN_POINT('Ctrl Pts',(0.142005473262988,-3.93215126651885,303.165581235262));
#6487=CARTESIAN_POINT('Ctrl Pts',(0.258167592750564,-3.9262380041259,303.171443010184));
#6488=CARTESIAN_POINT('Ctrl Pts',(0.373858259076704,-3.91519080021908,303.177304785106));
#6489=CARTESIAN_POINT('Ctrl Pts',(0.489532925472927,-3.90414512413204,303.183165749349));
#6490=CARTESIAN_POINT('Ctrl Pts',(0.604735858539977,-3.88796695768318,303.189026713592));
#6491=CARTESIAN_POINT('Ctrl Pts',(0.718982318147405,-3.8667238621592,303.194887677835));
#6492=CARTESIAN_POINT('Ctrl Pts',(0.833240385486079,-3.84547860828262,303.200749237567));
#6493=CARTESIAN_POINT('Ctrl Pts',(0.946541381310529,-3.81916747760947,303.206610797299));
#6494=CARTESIAN_POINT('Ctrl Pts',(1.05841062355686,-3.78790917947381,303.212472357031));
#6495=CARTESIAN_POINT('Ctrl Pts',(1.17427186087416,-3.75553544540976,303.218543083439));
#6496=CARTESIAN_POINT('Ctrl Pts',(1.28859679338039,-3.71785500023293,303.224613809847));
#6497=CARTESIAN_POINT('Ctrl Pts',(1.4008764291635,-3.67505567715839,303.230684536255));
#6498=CARTESIAN_POINT('Ctrl Pts',(1.50944726630239,-3.63367009282895,303.236554735633));
#6499=CARTESIAN_POINT('Ctrl Pts',(1.61610543337687,-3.58749868482086,303.242424935011));
#6500=CARTESIAN_POINT('Ctrl Pts',(1.72041322114842,-3.53675944170617,303.24829513439));
#6501=CARTESIAN_POINT('Ctrl Pts',(1.83006576712664,-3.48342030656202,303.254466124313));
#6502=CARTESIAN_POINT('Ctrl Pts',(1.9371202206171,-3.42503307634299,303.260637114235));
#6503=CARTESIAN_POINT('Ctrl Pts',(2.04110095740479,-3.36190360981413,303.266808104158));
#6504=CARTESIAN_POINT('Ctrl Pts',(2.14508169419248,-3.29877414328527,303.272979094081));
#6505=CARTESIAN_POINT('Ctrl Pts',(2.24598832120404,-3.23090278988649,303.279150084004));
#6506=CARTESIAN_POINT('Ctrl Pts',(2.34338506086676,-3.15864456001407,303.285321073927));
#6507=CARTESIAN_POINT('Ctrl Pts',(2.43545879049995,-3.09033544880476,303.291154801624));
#6508=CARTESIAN_POINT('Ctrl Pts',(2.52470367385015,-3.01787791041709,303.29698852932));
#6509=CARTESIAN_POINT('Ctrl Pts',(2.61071910442475,-2.94153612212932,303.302822257017));
#6510=CARTESIAN_POINT('Ctrl Pts',(2.69662537708536,-2.86529121541622,303.308648581419));
#6511=CARTESIAN_POINT('Ctrl Pts',(2.77931003431553,-2.78517213482679,303.314474905821));
#6512=CARTESIAN_POINT('Ctrl Pts',(2.85840257146368,-2.70148546904288,303.320301230224));
#6513=CARTESIAN_POINT('Ctrl Pts',(2.93741660425641,-2.61788186757821,303.32612177163));
#6514=CARTESIAN_POINT('Ctrl Pts',(3.01284532077852,-2.53071802572051,303.331942313036));
#6515=CARTESIAN_POINT('Ctrl Pts',(3.08435294146453,-2.44033930683401,303.337762854442));
#6516=CARTESIAN_POINT('Ctrl Pts',(3.15581096158886,-2.35002327826189,303.343579358487));
#6517=CARTESIAN_POINT('Ctrl Pts',(3.22335303577711,-2.25649713550921,303.349395862531));
#6518=CARTESIAN_POINT('Ctrl Pts',(3.28668226398882,-2.16014089715956,303.355212366576));
#6519=CARTESIAN_POINT('Ctrl Pts',(3.34998888490214,-2.06381905610629,303.361026794242));
#6520=CARTESIAN_POINT('Ctrl Pts',(3.40908541899942,-1.96466947753097,303.366841221908));
#6521=CARTESIAN_POINT('Ctrl Pts',(3.46371747678195,-1.86310231630882,303.372655649574));
#6522=CARTESIAN_POINT('Ctrl Pts',(3.51834370030402,-1.76154600163531,303.378469456306));
#6523=CARTESIAN_POINT('Ctrl Pts',(3.56850619716011,-1.65757298708004,303.384283263039));
#6524=CARTESIAN_POINT('Ctrl Pts',(3.6139962460256,-1.55161855290302,303.390097069771));
#6525=CARTESIAN_POINT('Ctrl Pts',(3.65949281823104,-1.44564892470421,303.395911710212));
#6526=CARTESIAN_POINT('Ctrl Pts',(3.70031544598483,-1.33769769774431,303.401726350653));
#6527=CARTESIAN_POINT('Ctrl Pts',(3.73630362763664,-1.22821993230418,303.407540991094));
#6528=CARTESIAN_POINT('Ctrl Pts',(3.7723264008866,-1.11863693757223,303.413361220528));
#6529=CARTESIAN_POINT('Ctrl Pts',(3.80350531868779,-1.00752487358253,303.419181449962));
#6530=CARTESIAN_POINT('Ctrl Pts',(3.82972983561874,-0.895353777102462,303.425001679396));
#6531=CARTESIAN_POINT('Ctrl Pts',(3.85596803231133,-0.783124167671821,303.430824944896));
#6532=CARTESIAN_POINT('Ctrl Pts',(3.87724660440776,-0.669834837519033,303.436648210396));
#6533=CARTESIAN_POINT('Ctrl Pts',(3.89350651409067,-0.555964049857084,303.442471475895));
#6534=CARTESIAN_POINT('Ctrl Pts',(3.90979039676959,-0.4419253754116,303.448303326997));
#6535=CARTESIAN_POINT('Ctrl Pts',(3.9210408005791,-0.327303948478049,303.454135178099));
#6536=CARTESIAN_POINT('Ctrl Pts',(3.92725071313894,-0.212581363599228,303.459967029201));
#6537=CARTESIAN_POINT('Ctrl Pts',(3.93110874066186,-0.141307752948724,303.463590178778));
#6538=CARTESIAN_POINT('Ctrl Pts',(3.93302229924915,-0.06999509726729,303.467213328355));
#6539=CARTESIAN_POINT('Ctrl Pts',(3.93299980390471,0.00124196841145939,
303.470836477931));
#6540=CARTESIAN_POINT('',(3.93299876362378,-0.00311854674718142,304.720836477934));
#6541=CARTESIAN_POINT('Ctrl Pts',(3.9329998039045,0.00124196907699985,303.470836477965));
#6542=CARTESIAN_POINT('Ctrl Pts',(3.93297724349898,0.0726850284083443,303.474470104473));
#6543=CARTESIAN_POINT('Ctrl Pts',(3.93100814933993,0.144094335620644,303.47810373098));
#6544=CARTESIAN_POINT('Ctrl Pts',(3.92709733580092,0.215396181826265,303.481737357488));
#6545=CARTESIAN_POINT('Ctrl Pts',(3.92076713854636,0.330808166210949,303.487618888865));
#6546=CARTESIAN_POINT('Ctrl Pts',(3.90933474442503,0.446126778365148,303.493500420243));
#6547=CARTESIAN_POINT('Ctrl Pts',(3.89280348111204,0.560865453956625,303.49938195162));
#6548=CARTESIAN_POINT('Ctrl Pts',(3.87629310999173,0.675459122934113,303.505256049925));
#6549=CARTESIAN_POINT('Ctrl Pts',(3.85469674391957,0.789473908938345,303.51113014823));
#6550=CARTESIAN_POINT('Ctrl Pts',(3.82806966980477,0.902425400307849,303.517004246534));
#6551=CARTESIAN_POINT('Ctrl Pts',(3.80146919228528,1.01526406947644,303.522872477464));
#6552=CARTESIAN_POINT('Ctrl Pts',(3.76984809661393,1.12704115818054,303.528740708395));
#6553=CARTESIAN_POINT('Ctrl Pts',(3.73331311205916,1.23728016525246,303.534608939325));
#6554=CARTESIAN_POINT('Ctrl Pts',(3.69607585717752,1.34963817099025,303.540589968563));
#6555=CARTESIAN_POINT('Ctrl Pts',(3.65373391493134,1.46039792427612,303.546570997802));
#6556=CARTESIAN_POINT('Ctrl Pts',(3.60645441286487,1.56906837579739,303.55255202704));
#6557=CARTESIAN_POINT('Ctrl Pts',(3.56011760593738,1.67557207213044,303.55841380191));
#6558=CARTESIAN_POINT('Ctrl Pts',(3.50903848508585,1.78006861692458,303.564275576779));
#6559=CARTESIAN_POINT('Ctrl Pts',(3.45342355261713,1.88211444025843,303.570137351648));
#6560=CARTESIAN_POINT('Ctrl Pts',(3.39781631164719,1.98414615074,303.575998315839));
#6561=CARTESIAN_POINT('Ctrl Pts',(3.33767470358564,2.08372745229958,303.58185928003));
#6562=CARTESIAN_POINT('Ctrl Pts',(3.27325131613053,2.18043913500234,303.587720244221));
#6563=CARTESIAN_POINT('Ctrl Pts',(3.2088213830904,2.27716064386555,303.593581803901));
#6564=CARTESIAN_POINT('Ctrl Pts',(3.14010903413636,2.37101161154408,303.599443363581));
#6565=CARTESIAN_POINT('Ctrl Pts',(3.06740993956996,2.46160217391589,303.605304923261));
#6566=CARTESIAN_POINT('Ctrl Pts',(2.99211661446502,2.55542541483493,303.611375649743));
#6567=CARTESIAN_POINT('Ctrl Pts',(2.91254699512177,2.64575083865355,303.617446376226));
#6568=CARTESIAN_POINT('Ctrl Pts',(2.82907379728069,2.73218419026606,303.623517102708));
#6569=CARTESIAN_POINT('Ctrl Pts',(2.74835787122056,2.81576249082629,303.629387302036));
#6570=CARTESIAN_POINT('Ctrl Pts',(2.66399252506124,2.89570154048497,303.635257501364));
#6571=CARTESIAN_POINT('Ctrl Pts',(2.5763501968945,2.97168448240416,303.641127700692));
#6572=CARTESIAN_POINT('Ctrl Pts',(2.4842170501855,3.05156081250237,303.647298690751));
#6573=CARTESIAN_POINT('Ctrl Pts',(2.38846261490447,3.1270645437864,303.653469680811));
#6574=CARTESIAN_POINT('Ctrl Pts',(2.28955502976185,3.19787847888131,303.65964067087));
#6575=CARTESIAN_POINT('Ctrl Pts',(2.19064744461922,3.26869241397621,303.665811660929));
#6576=CARTESIAN_POINT('Ctrl Pts',(2.08858718539478,3.33481632871994,303.671982650989));
#6577=CARTESIAN_POINT('Ctrl Pts',(1.98387193327577,3.39598898001166,303.678153641048));
#6578=CARTESIAN_POINT('Ctrl Pts',(1.88406849122884,3.45429224562489,303.684035172499));
#6579=CARTESIAN_POINT('Ctrl Pts',(1.78153192407126,3.5082860844213,303.689916703951));
#6580=CARTESIAN_POINT('Ctrl Pts',(1.67667012221104,3.55770520157092,303.695798235402));
#6581=CARTESIAN_POINT('Ctrl Pts',(1.5719408445903,3.60706186289011,303.701672333779));
#6582=CARTESIAN_POINT('Ctrl Pts',(1.46489254604909,3.65185512709515,303.707546432157));
#6583=CARTESIAN_POINT('Ctrl Pts',(1.35595994737052,3.69186424738599,303.713420530535));
#6584=CARTESIAN_POINT('Ctrl Pts',(1.24713615661049,3.73183340434947,303.719288761537));
#6585=CARTESIAN_POINT('Ctrl Pts',(1.13643219418166,3.76702778222905,303.72515699254));
#6586=CARTESIAN_POINT('Ctrl Pts',(1.02430452134174,3.79727392316631,303.731025223543));
#6587=CARTESIAN_POINT('Ctrl Pts',(0.910021548103897,3.8281014506422,303.737006252754));
#6588=CARTESIAN_POINT('Ctrl Pts',(0.794259959271355,3.85378836150459,303.742987281965));
#6589=CARTESIAN_POINT('Ctrl Pts',(0.677521633415707,3.87420358735234,303.748968311176));
#6590=CARTESIAN_POINT('Ctrl Pts',(0.563110924342039,3.89421175903048,303.754830086116));
#6591=CARTESIAN_POINT('Ctrl Pts',(0.447762491066853,3.90915644642796,303.760691861056));
#6592=CARTESIAN_POINT('Ctrl Pts',(0.33196028223957,3.91896559962134,303.766553635996));
#6593=CARTESIAN_POINT('Ctrl Pts',(0.216174088777913,3.92877339621559,303.772414600256));
#6594=CARTESIAN_POINT('Ctrl Pts',(0.0999346547980537,3.93344703631303,303.778275564516));
#6595=CARTESIAN_POINT('Ctrl Pts',(-0.0162690097360618,3.9329663511556,303.784136528777));
#6596=CARTESIAN_POINT('Ctrl Pts',(-0.132484480848625,3.93248561715938,303.789998088526));
#6597=CARTESIAN_POINT('Ctrl Pts',(-0.248663763486618,3.92684951855352,303.795859648275));
#6598=CARTESIAN_POINT('Ctrl Pts',(-0.364318601620493,3.9160900087349,303.801721208024));
#6599=CARTESIAN_POINT('Ctrl Pts',(-0.484100520964409,3.90494655154738,303.807791934406));
#6600=CARTESIAN_POINT('Ctrl Pts',(-0.603319392770055,3.88830724208517,303.813862660788));
#6601=CARTESIAN_POINT('Ctrl Pts',(-0.721440848531566,3.86626591197114,303.81993338717));
#6602=CARTESIAN_POINT('Ctrl Pts',(-0.835660540602558,3.844952646551,303.825803586563));
#6603=CARTESIAN_POINT('Ctrl Pts',(-0.948853777669127,3.81858875686602,303.831673785957));
#6604=CARTESIAN_POINT('Ctrl Pts',(-1.06055093604124,3.78731048529983,303.837543985351));
#6605=CARTESIAN_POINT('Ctrl Pts',(-1.17797148469267,3.75442950729021,303.843714975227));
#6606=CARTESIAN_POINT('Ctrl Pts',(-1.29373807183921,3.71611734535315,303.849885965103));
#6607=CARTESIAN_POINT('Ctrl Pts',(-1.40732806354444,3.67258992014631,303.85605695498));
#6608=CARTESIAN_POINT('Ctrl Pts',(-1.52091805524966,3.62906249493948,303.862227944856));
#6609=CARTESIAN_POINT('Ctrl Pts',(-1.63233100231149,3.58032008001792,303.868398934732));
#6610=CARTESIAN_POINT('Ctrl Pts',(-1.74107469043908,3.52663407831213,303.874569924608));
#6611=CARTESIAN_POINT('Ctrl Pts',(-1.84471761548938,3.47546628782378,303.880451456237));
#6612=CARTESIAN_POINT('Ctrl Pts',(-1.9462699658564,3.41964332459861,303.886332987867));
#6613=CARTESIAN_POINT('Ctrl Pts',(-2.04528561596243,3.35935942541687,303.892214519496));
#6614=CARTESIAN_POINT('Ctrl Pts',(-2.14417613021617,3.29915171295002,303.898088618054));
#6615=CARTESIAN_POINT('Ctrl Pts',(-2.24053597150076,3.23449448940438,303.903962716611));
#6616=CARTESIAN_POINT('Ctrl Pts',(-2.33394140916372,3.16562892623107,303.909836815168));
#6617=CARTESIAN_POINT('Ctrl Pts',(-2.42725354831772,3.09683214978498,303.915705046351));
#6618=CARTESIAN_POINT('Ctrl Pts',(-2.51761682459389,3.02383563861823,303.921573277534));
#6619=CARTESIAN_POINT('Ctrl Pts',(-2.60463499393594,2.94692476123235,303.927441508718));
#6620=CARTESIAN_POINT('Ctrl Pts',(-2.69332580904191,2.86853551841737,303.933422537861));
#6621=CARTESIAN_POINT('Ctrl Pts',(-2.77854121904429,2.78608009789253,303.939403567005));
#6622=CARTESIAN_POINT('Ctrl Pts',(-2.85989533299847,2.69990512505413,303.945384596149));
#6623=CARTESIAN_POINT('Ctrl Pts',(-2.93962735064849,2.6154483702401,303.951246371271));
#6624=CARTESIAN_POINT('Ctrl Pts',(-3.01565032955656,2.52741932842187,303.957108146393));
#6625=CARTESIAN_POINT('Ctrl Pts',(-3.08763751042896,2.43618217795634,303.962969921515));
#6626=CARTESIAN_POINT('Ctrl Pts',(-3.15961473552719,2.3449576455216,303.968830885958));
#6627=CARTESIAN_POINT('Ctrl Pts',(-3.22755701756412,2.25052620999185,303.974691850401));
#6628=CARTESIAN_POINT('Ctrl Pts',(-3.2911781055904,2.15328485744047,303.980552814844));
#6629=CARTESIAN_POINT('Ctrl Pts',(-3.35480565767605,2.05603362492796,303.986414374775));
#6630=CARTESIAN_POINT('Ctrl Pts',(-3.41411091750535,1.95597225245877,303.992275934707));
#6631=CARTESIAN_POINT('Ctrl Pts',(-3.4688515474911,1.85352581354256,303.998137494638));
#6632=CARTESIAN_POINT('Ctrl Pts',(-3.5255455635182,1.74742363584846,304.004208220765));
#6633=CARTESIAN_POINT('Ctrl Pts',(-3.57734286543658,1.63876341196607,304.010278946893));
#6634=CARTESIAN_POINT('Ctrl Pts',(-3.62402734990921,1.52804278968556,304.01634967302));
#6635=CARTESIAN_POINT('Ctrl Pts',(-3.66916976535286,1.42097946049541,304.022219872595));
#6636=CARTESIAN_POINT('Ctrl Pts',(-3.70953171257518,1.31199011416512,304.02809007217));
#6637=CARTESIAN_POINT('Ctrl Pts',(-3.74496815269547,1.20154173264879,304.033960271744));
#6638=CARTESIAN_POINT('Ctrl Pts',(-3.78222036085575,1.0854339609526,304.040131261148));
#6639=CARTESIAN_POINT('Ctrl Pts',(-3.81402878617087,0.967714182480075,304.046302250552));
#6640=CARTESIAN_POINT('Ctrl Pts',(-3.84028567851689,0.848937516769068,304.052473239956));
#6641=CARTESIAN_POINT('Ctrl Pts',(-3.86654257086292,0.730160851058062,304.05864422936));
#6642=CARTESIAN_POINT('Ctrl Pts',(-3.88724791104503,0.610327823699778,304.064815218764));
#6643=CARTESIAN_POINT('Ctrl Pts',(-3.90235701070404,0.489998735721905,304.070986208168));
#6644=CARTESIAN_POINT('Ctrl Pts',(-3.91675739780014,0.375313844834309,304.076867739046));
#6645=CARTESIAN_POINT('Ctrl Pts',(-3.92612106289952,0.259808859864661,304.082749269924));
#6646=CARTESIAN_POINT('Ctrl Pts',(-3.93036431193775,0.143963104461184,304.088630800802));
#6647=CARTESIAN_POINT('Ctrl Pts',(-3.93460219836204,0.0282637548089151,
304.094504898607));
#6648=CARTESIAN_POINT('Ctrl Pts',(-3.93373252396109,-0.0877751007682438,
304.100378996412));
#6649=CARTESIAN_POINT('Ctrl Pts',(-3.92772310194429,-0.203666969470105,
304.106253094217));
#6650=CARTESIAN_POINT('Ctrl Pts',(-3.9217196824706,-0.319443078962975,304.112121324648));
#6651=CARTESIAN_POINT('Ctrl Pts',(-3.91058674917664,-0.43507208468703,304.11798955508));
#6652=CARTESIAN_POINT('Ctrl Pts',(-3.89434414314356,-0.550066082178732,
304.123857785511));
#6653=CARTESIAN_POINT('Ctrl Pts',(-3.87778932209959,-0.667270491725312,
304.129838814937));
#6654=CARTESIAN_POINT('Ctrl Pts',(-3.8559263462702,-0.783814794207662,304.135819844362));
#6655=CARTESIAN_POINT('Ctrl Pts',(-3.82883188209237,-0.899185975576223,
304.141800873788));
#6656=CARTESIAN_POINT('Ctrl Pts',(-3.80227765128556,-1.01225678437351,304.147662648163));
#6657=CARTESIAN_POINT('Ctrl Pts',(-3.77069871852815,-1.12420040153827,304.153524422539));
#6658=CARTESIAN_POINT('Ctrl Pts',(-3.73421897735477,-1.23454349018715,304.159386196914));
#6659=CARTESIAN_POINT('Ctrl Pts',(-3.69774428128287,-1.34487131852822,304.165247160614));
#6660=CARTESIAN_POINT('Ctrl Pts',(-3.65637025391693,-1.45359866766378,304.171108124313));
#6661=CARTESIAN_POINT('Ctrl Pts',(-3.61027048613083,-1.56026793114922,304.176969088013));
#6662=CARTESIAN_POINT('Ctrl Pts',(-3.56416603446161,-1.66694803257131,304.182830647205));
#6663=CARTESIAN_POINT('Ctrl Pts',(-3.51333505124083,-1.77156925463698,304.188692206397));
#6664=CARTESIAN_POINT('Ctrl Pts',(-3.4579987614115,-1.87369516359425,304.194553765589));
#6665=CARTESIAN_POINT('Ctrl Pts',(-3.4006878126345,-1.9794654050598,304.200624492767));
#6666=CARTESIAN_POINT('Ctrl Pts',(-3.33854423471032,-2.08255849745215,304.206695219946));
#6667=CARTESIAN_POINT('Ctrl Pts',(-3.27186427265409,-2.1825199154486,304.212765947124));
#6668=CARTESIAN_POINT('Ctrl Pts',(-3.20738688382552,-2.27917940680487,304.218636145976));
#6669=CARTESIAN_POINT('Ctrl Pts',(-3.13866836723035,-2.37291054688362,304.224506344829));
#6670=CARTESIAN_POINT('Ctrl Pts',(-3.06601852864048,-2.4633350121397,304.230376543681));
#6671=CARTESIAN_POINT('Ctrl Pts',(-2.98964606901135,-2.55839288090167,304.236547535022));
#6672=CARTESIAN_POINT('Ctrl Pts',(-2.90892907964158,-2.64979582975975,304.242718526363));
#6673=CARTESIAN_POINT('Ctrl Pts',(-2.8242714652856,-2.73714809434446,304.248889517705));
#6674=CARTESIAN_POINT('Ctrl Pts',(-2.73961385092963,-2.82450035892918,304.255060509046));
#6675=CARTESIAN_POINT('Ctrl Pts',(-2.65101603963972,-2.90780163364738,304.261231500387));
#6676=CARTESIAN_POINT('Ctrl Pts',(-2.55892100416771,-2.98670592700877,304.267402491728));
#6677=CARTESIAN_POINT('Ctrl Pts',(-2.47114582302524,-3.06190909737749,304.273284023561));
#6678=CARTESIAN_POINT('Ctrl Pts',(-2.37991126582219,-3.13336075402604,304.279165555394));
#6679=CARTESIAN_POINT('Ctrl Pts',(-2.28557123594851,-3.20072696826905,304.285047087227));
#6680=CARTESIAN_POINT('Ctrl Pts',(-2.19135043296191,-3.26800804512098,304.290921185983));
#6681=CARTESIAN_POINT('Ctrl Pts',(-2.09403229516527,-3.33121371109447,304.296795284739));
#6682=CARTESIAN_POINT('Ctrl Pts',(-1.99400508673938,-3.39004907251466,304.302669383495));
#6683=CARTESIAN_POINT('Ctrl Pts',(-1.89407779109888,-3.44882566587631,304.308537614871));
#6684=CARTESIAN_POINT('Ctrl Pts',(-1.79144716068113,-3.50324043079569,304.314405846248));
#6685=CARTESIAN_POINT('Ctrl Pts',(-1.68653130243143,-3.55304111514614,304.320274077624));
#6686=CARTESIAN_POINT('Ctrl Pts',(-1.57959877749203,-3.60379905593932,304.326255106694));
#6687=CARTESIAN_POINT('Ctrl Pts',(-1.4702926183206,-3.64976344900962,304.332236135763));
#6688=CARTESIAN_POINT('Ctrl Pts',(-1.35908319433564,-3.69071563126644,304.338217164832));
#6689=CARTESIAN_POINT('Ctrl Pts',(-1.25009113841468,-3.730851281454,304.344078940134));
#6690=CARTESIAN_POINT('Ctrl Pts',(-1.13927141557552,-3.76617259484159,304.349940715435));
#6691=CARTESIAN_POINT('Ctrl Pts',(-1.02708730308535,-3.79652218113379,304.355802490736));
#6692=CARTESIAN_POINT('Ctrl Pts',(-0.914918705681009,-3.82686757007196,
304.361663455353));
#6693=CARTESIAN_POINT('Ctrl Pts',(-0.801386491296358,-3.85224249181356,
304.367524419969));
#6694=CARTESIAN_POINT('Ctrl Pts',(-0.686968190209235,-3.87253969710327,
304.373385384586));
#6695=CARTESIAN_POINT('Ctrl Pts',(-0.572538264052435,-3.89283896461923,
304.379246944685));
#6696=CARTESIAN_POINT('Ctrl Pts',(-0.457222477702342,-3.90805941817867,
304.385108504785));
#6697=CARTESIAN_POINT('Ctrl Pts',(-0.341506935919518,-3.91814522608834,
304.390970064884));
#6698=CARTESIAN_POINT('Ctrl Pts',(-0.221662164081661,-3.92859093916294,
304.397040790751));
#6699=CARTESIAN_POINT('Ctrl Pts',(-0.101389048498594,-3.93352866481337,
304.403111516618));
#6700=CARTESIAN_POINT('Ctrl Pts',(0.0187698763244972,-3.93295521100136,
304.409182242485));
#6701=CARTESIAN_POINT('Ctrl Pts',(0.134959752648127,-3.9324006993195,304.415052442212));
#6702=CARTESIAN_POINT('Ctrl Pts',(0.251042448178382,-3.9266934278433,304.420922641939));
#6703=CARTESIAN_POINT('Ctrl Pts',(0.36653154990781,-3.91588350476903,304.426792841666));
#6704=CARTESIAN_POINT('Ctrl Pts',(0.487938316675192,-3.90451968091208,304.432963830603));
#6705=CARTESIAN_POINT('Ctrl Pts',(0.608688522367494,-3.88751650818532,304.43913481954));
#6706=CARTESIAN_POINT('Ctrl Pts',(0.728229356076895,-3.86499301486404,304.445305808477));
#6707=CARTESIAN_POINT('Ctrl Pts',(0.847770189786295,-3.84246952154276,304.451476797414));
#6708=CARTESIAN_POINT('Ctrl Pts',(0.966101160649947,-3.81442589648643,304.457647786351));
#6709=CARTESIAN_POINT('Ctrl Pts',(1.08268947065621,-3.78104119392135,304.463818775288));
#6710=CARTESIAN_POINT('Ctrl Pts',(1.19380909821671,-3.74922243168823,304.469700308285));
#6711=CARTESIAN_POINT('Ctrl Pts',(1.30370387732472,-3.71244979145023,304.475581841282));
#6712=CARTESIAN_POINT('Ctrl Pts',(1.41190014870259,-3.67083464216159,304.481463374279));
#6713=CARTESIAN_POINT('Ctrl Pts',(1.51995968195813,-3.62927208597345,304.487337474213));
#6714=CARTESIAN_POINT('Ctrl Pts',(1.62632459563915,-3.58287933893364,304.493211574146));
#6715=CARTESIAN_POINT('Ctrl Pts',(1.73053487570909,-3.53181795170059,304.499085674079));
#6716=CARTESIAN_POINT('Ctrl Pts',(1.83464106493965,-3.48080756733071,304.504953906645));
#6717=CARTESIAN_POINT('Ctrl Pts',(1.93659653404071,-3.4251379994445,304.510822139211));
#6718=CARTESIAN_POINT('Ctrl Pts',(2.03596041321068,-3.36501919694955,304.516690371777));
#6719=CARTESIAN_POINT('Ctrl Pts',(2.13723421230144,-3.30374482263658,304.522671400405));
#6720=CARTESIAN_POINT('Ctrl Pts',(2.23581535788513,-3.23784856044379,304.528652429033));
#6721=CARTESIAN_POINT('Ctrl Pts',(2.33126221796963,-3.16760247996293,304.534633457661));
#6722=CARTESIAN_POINT('Ctrl Pts',(2.42480602078419,-3.09875699363494,304.540495234173));
#6723=CARTESIAN_POINT('Ctrl Pts',(2.51533901948406,-3.02573379443896,304.546357010686));
#6724=CARTESIAN_POINT('Ctrl Pts',(2.6024746236808,-2.94883279164782,304.552218787198));
#6725=CARTESIAN_POINT('Ctrl Pts',(2.68959817709415,-2.871942424203,304.558079753031));
#6726=CARTESIAN_POINT('Ctrl Pts',(2.77332496173136,-2.79117559211882,304.563940718864));
#6727=CARTESIAN_POINT('Ctrl Pts',(2.85330237920067,-2.7068717244908,304.569801684697));
#6728=CARTESIAN_POINT('Ctrl Pts',(2.93328792255268,-2.62255929140316,304.575663246018));
#6729=CARTESIAN_POINT('Ctrl Pts',(3.00952305802561,-2.53470940712846,304.581524807338));
#6730=CARTESIAN_POINT('Ctrl Pts',(3.08169337310605,-2.44369698492965,304.587386368659));
#6731=CARTESIAN_POINT('Ctrl Pts',(3.15643900026495,-2.34943689241214,304.593457092841));
#6732=CARTESIAN_POINT('Ctrl Pts',(3.22682399347094,-2.25178471503604,304.599527817024));
#6733=CARTESIAN_POINT('Ctrl Pts',(3.29254678060488,-2.15119145998872,304.605598541206));
#6734=CARTESIAN_POINT('Ctrl Pts',(3.35609866596458,-2.05392091971635,304.611468742154));
#6735=CARTESIAN_POINT('Ctrl Pts',(3.41529131825077,-1.95390091967525,304.617338943101));
#6736=CARTESIAN_POINT('Ctrl Pts',(3.46989856609507,-1.85156499778198,304.623209144048));
#6737=CARTESIAN_POINT('Ctrl Pts',(3.52730384984093,-1.74398545723404,304.629380129848));
#6738=CARTESIAN_POINT('Ctrl Pts',(3.57964114955997,-1.6338468545087,304.635551115649));
#6739=CARTESIAN_POINT('Ctrl Pts',(3.62670522896991,-1.52167610948004,304.641722101449));
#6740=CARTESIAN_POINT('Ctrl Pts',(3.67376930837985,-1.40950536445138,304.647893087249));
#6741=CARTESIAN_POINT('Ctrl Pts',(3.7155600546515,-1.29530299081345,304.654064073049));
#6742=CARTESIAN_POINT('Ctrl Pts',(3.75193335141045,-1.17961227807018,304.660235058849));
#6743=CARTESIAN_POINT('Ctrl Pts',(3.79353038241778,-1.04730669694197,304.66729228793));
#6744=CARTESIAN_POINT('Ctrl Pts',(3.82815265954103,-0.912711690282679,304.674349517011));
#6745=CARTESIAN_POINT('Ctrl Pts',(3.85558531402917,-0.776499121855645,304.681406746093));
#6746=CARTESIAN_POINT('Ctrl Pts',(3.88272233690686,-0.641754466093948,304.688387922016));
#6747=CARTESIAN_POINT('Ctrl Pts',(3.90282382882847,-0.505426965597625,304.69536909794));
#6748=CARTESIAN_POINT('Ctrl Pts',(3.91572817428225,-0.368187269106653,304.702350273864));
#6749=CARTESIAN_POINT('Ctrl Pts',(3.92711844081548,-0.247050034554848,304.708512341887));
#6750=CARTESIAN_POINT('Ctrl Pts',(3.93290196110154,-0.12520239898195,304.714674409911));
#6751=CARTESIAN_POINT('Ctrl Pts',(3.93299876362378,-0.00311854674718404,
304.720836477935));
#6752=CARTESIAN_POINT('',(3.93299889167903,0.00295263467253422,305.970836478001));
#6753=CARTESIAN_POINT('Ctrl Pts',(3.93299876362426,-0.00311854614236361,
304.720836477965));
#6754=CARTESIAN_POINT('Ctrl Pts',(3.93309044288826,0.112504059879749,304.726672420641));
#6755=CARTESIAN_POINT('Ctrl Pts',(3.92807921482838,0.228206433372478,304.732508363318));
#6756=CARTESIAN_POINT('Ctrl Pts',(3.9179707306054,0.343503062751093,304.738344305994));
#6757=CARTESIAN_POINT('Ctrl Pts',(3.90786516887247,0.45876635842263,304.744178561426));
#6758=CARTESIAN_POINT('Ctrl Pts',(3.89266531672084,0.573623729284123,304.750012816858));
#6759=CARTESIAN_POINT('Ctrl Pts',(3.87242885259085,0.68759274401486,304.75584707229));
#6760=CARTESIAN_POINT('Ctrl Pts',(3.85219326980367,0.801556795142779,304.761681073628));
#6761=CARTESIAN_POINT('Ctrl Pts',(3.82692158407276,0.914632157675829,304.767515074965));
#6762=CARTESIAN_POINT('Ctrl Pts',(3.79672283545177,1.02634531750238,304.773349076302));
#6763=CARTESIAN_POINT('Ctrl Pts',(3.76651798635264,1.13808104461139,304.779184256172));
#6764=CARTESIAN_POINT('Ctrl Pts',(3.73138420430134,1.24845362061568,304.785019436041));
#6765=CARTESIAN_POINT('Ctrl Pts',(3.69148055445412,1.3570041695172,304.79085461591));
#6766=CARTESIAN_POINT('Ctrl Pts',(3.65153425451423,1.46567074016081,304.796696032577));
#6767=CARTESIAN_POINT('Ctrl Pts',(3.6068080497739,1.57251100390095,304.802537449243));
#6768=CARTESIAN_POINT('Ctrl Pts',(3.55750944186126,1.67708543940611,304.80837886591));
#6769=CARTESIAN_POINT('Ctrl Pts',(3.50818307740112,1.78171875335448,304.814223571463));
#6770=CARTESIAN_POINT('Ctrl Pts',(3.45427937636074,1.88408333071874,304.820068277017));
#6771=CARTESIAN_POINT('Ctrl Pts',(3.39605127137777,1.98376529916557,304.825912982571));
#6772=CARTESIAN_POINT('Ctrl Pts',(3.33772955186372,2.08360752837884,304.831767084779));
#6773=CARTESIAN_POINT('Ctrl Pts',(3.27506976679879,2.18075818474117,304.837621186986));
#6774=CARTESIAN_POINT('Ctrl Pts',(3.2083677514685,2.27483304251915,304.843475289194));
#6775=CARTESIAN_POINT('Ctrl Pts',(3.15832482018389,2.3454123439103,304.847867306933));
#6776=CARTESIAN_POINT('Ctrl Pts',(3.10600752986126,2.41426100054013,304.852259324671));
#6777=CARTESIAN_POINT('Ctrl Pts',(3.05155477118755,2.48123003335896,304.85665134241));
#6778=CARTESIAN_POINT('Ctrl Pts',(2.97863477273715,2.57091110532514,304.862532879626));
#6779=CARTESIAN_POINT('Ctrl Pts',(2.90164055801538,2.65751939625126,304.868414416843));
#6780=CARTESIAN_POINT('Ctrl Pts',(2.82086064578117,2.74066309806277,304.874295954059));
#6781=CARTESIAN_POINT('Ctrl Pts',(2.74018282350456,2.8237017225505,304.880170058167));
#6782=CARTESIAN_POINT('Ctrl Pts',(2.65572910359967,2.90328417339925,304.886044162274));
#6783=CARTESIAN_POINT('Ctrl Pts',(2.56782878935635,2.97905090734494,304.891918266382));
#6784=CARTESIAN_POINT('Ctrl Pts',(2.48001627536094,3.05474196081006,304.897786503072));
#6785=CARTESIAN_POINT('Ctrl Pts',(2.38876432557151,3.12662461182242,304.903654739763));
#6786=CARTESIAN_POINT('Ctrl Pts',(2.29443922717336,3.19437593792717,304.909522976454));
#6787=CARTESIAN_POINT('Ctrl Pts',(2.19830115435824,3.2634294775788,304.915504003517));
#6788=CARTESIAN_POINT('Ctrl Pts',(2.09897088014991,3.32819092729918,304.92148503058));
#6789=CARTESIAN_POINT('Ctrl Pts',(1.99687211471548,3.38836107247615,304.927466057643));
#6790=CARTESIAN_POINT('Ctrl Pts',(1.89680894080443,3.44733157692327,304.933327838132));
#6791=CARTESIAN_POINT('Ctrl Pts',(1.79408701740145,3.50189194113393,304.939189618621));
#6792=CARTESIAN_POINT('Ctrl Pts',(1.68913403009981,3.55180450311652,304.94505139911));
#6793=CARTESIAN_POINT('Ctrl Pts',(1.58419555880846,3.60171016171043,304.950912368859));
#6794=CARTESIAN_POINT('Ctrl Pts',(1.47702700908186,3.64696911966955,304.956773338607));
#6795=CARTESIAN_POINT('Ctrl Pts',(1.36807905218987,3.68739050101278,304.962634308355));
#6796=CARTESIAN_POINT('Ctrl Pts',(1.25912002717839,3.72781598879995,304.968495873525));
#6797=CARTESIAN_POINT('Ctrl Pts',(1.14838162173231,3.76340277975507,304.974357438694));
#6798=CARTESIAN_POINT('Ctrl Pts',(1.0363321338903,3.79400905484771,304.980219003864));
#6799=CARTESIAN_POINT('Ctrl Pts',(0.920284477662538,3.82570742811801,304.986289722372));
#6800=CARTESIAN_POINT('Ctrl Pts',(0.802830885987274,3.85206308735008,304.992360440881));
#6801=CARTESIAN_POINT('Ctrl Pts',(0.684504583500926,3.87297591977619,304.99843115939));
#6802=CARTESIAN_POINT('Ctrl Pts',(0.5700865613404,3.89319800796529,305.004301363987));
#6803=CARTESIAN_POINT('Ctrl Pts',(0.454852991523888,3.90833114846625,305.010171568585));
#6804=CARTESIAN_POINT('Ctrl Pts',(0.339291411066153,3.91833770091052,305.016041773183));
#6805=CARTESIAN_POINT('Ctrl Pts',(0.217808817780249,3.92885695770821,305.022212748647));
#6806=CARTESIAN_POINT('Ctrl Pts',(0.0959642402970337,3.93371035043805,305.028383724111));
#6807=CARTESIAN_POINT('Ctrl Pts',(-0.0256771418625223,3.93291618069668,
305.034554699576));
#6808=CARTESIAN_POINT('Ctrl Pts',(-0.147318524022069,3.93212201095531,305.04072567504));
#6809=CARTESIAN_POINT('Ctrl Pts',(-0.268756194151563,3.92568037682122,305.046896650504));
#6810=CARTESIAN_POINT('Ctrl Pts',(-0.389433934093832,3.91367221557659,305.053067625969));
#6811=CARTESIAN_POINT('Ctrl Pts',(-0.50445161464586,3.90222726429798,305.058949168704));
#6812=CARTESIAN_POINT('Ctrl Pts',(-0.619149616709469,3.88568926349385,305.064830711439));
#6813=CARTESIAN_POINT('Ctrl Pts',(-0.733042001163635,3.86408312857397,305.070712254175));
#6814=CARTESIAN_POINT('Ctrl Pts',(-0.846790450691664,3.8425042990569,305.076586363933));
#6815=CARTESIAN_POINT('Ctrl Pts',(-0.959734906402532,3.81587015009463,305.082460473692));
#6816=CARTESIAN_POINT('Ctrl Pts',(-1.07139388540056,3.78425740962825,305.088334583451));
#6817=CARTESIAN_POINT('Ctrl Pts',(-1.18294133498977,3.7526762452186,305.094202825916));
#6818=CARTESIAN_POINT('Ctrl Pts',(-1.29320546803174,3.71612649307839,305.100071068381));
#6819=CARTESIAN_POINT('Ctrl Pts',(-1.40171498704683,3.67473592181647,305.105939310847));
#6820=CARTESIAN_POINT('Ctrl Pts',(-1.51230996396627,3.6325498600318,305.111920335792));
#6821=CARTESIAN_POINT('Ctrl Pts',(-1.62108175866984,3.58533506478871,305.117901360737));
#6822=CARTESIAN_POINT('Ctrl Pts',(-1.72754722374054,3.533280287459,305.123882385682));
#6823=CARTESIAN_POINT('Ctrl Pts',(-1.83189018077566,3.48226328029353,305.12974417221));
#6824=CARTESIAN_POINT('Ctrl Pts',(-1.93401752879696,3.42659767395453,305.135605958738));
#6825=CARTESIAN_POINT('Ctrl Pts',(-2.03349529634568,3.36650945041597,305.141467745267));
#6826=CARTESIAN_POINT('Ctrl Pts',(-2.13295930665367,3.30642953675584,305.147328721141));
#6827=CARTESIAN_POINT('Ctrl Pts',(-2.22977411279647,3.24192843509472,305.153189697016));
#6828=CARTESIAN_POINT('Ctrl Pts',(-2.32353212423129,3.17327708649358,305.159050672891));
#6829=CARTESIAN_POINT('Ctrl Pts',(-2.4172996618925,3.10461876261345,305.164912244266));
#6830=CARTESIAN_POINT('Ctrl Pts',(-2.50800945517101,3.03180959680641,305.170773815642));
#6831=CARTESIAN_POINT('Ctrl Pts',(-2.59528514209377,2.95516226817197,305.176635387017));
#6832=CARTESIAN_POINT('Ctrl Pts',(-2.68567479525653,2.87578018943508,305.182706097227));
#6833=CARTESIAN_POINT('Ctrl Pts',(-2.77238034983704,2.7922812563357,305.188776807436));
#6834=CARTESIAN_POINT('Ctrl Pts',(-2.85502448088432,2.7050553069302,305.194847517645));
#6835=CARTESIAN_POINT('Ctrl Pts',(-2.93493909807435,2.62071019654613,305.200717728588));
#6836=CARTESIAN_POINT('Ctrl Pts',(-3.01105610450854,2.53288072603806,305.206587939531));
#6837=CARTESIAN_POINT('Ctrl Pts',(-3.08307547968066,2.44195302710594,305.212458150474));
#6838=CARTESIAN_POINT('Ctrl Pts',(-3.15878462819027,2.34636682345398,305.218629110317));
#6839=CARTESIAN_POINT('Ctrl Pts',(-3.22996484790023,2.24735695006518,305.224800070159));
#6840=CARTESIAN_POINT('Ctrl Pts',(-3.29632003011824,2.14540515032506,305.230971030002));
#6841=CARTESIAN_POINT('Ctrl Pts',(-3.36267521233624,2.04345335058495,305.237141989844));
#6842=CARTESIAN_POINT('Ctrl Pts',(-3.42420515423831,1.93856010973155,305.243312949687));
#6843=CARTESIAN_POINT('Ctrl Pts',(-3.48067095548873,1.83123420119251,305.249483909529));
#6844=CARTESIAN_POINT('Ctrl Pts',(-3.53448793321464,1.72894297532923,305.255365388248));
#6845=CARTESIAN_POINT('Ctrl Pts',(-3.58387854436078,1.62411255661549,305.261246866967));
#6846=CARTESIAN_POINT('Ctrl Pts',(-3.62859585370637,1.51716219649217,305.267128345686));
#6847=CARTESIAN_POINT('Ctrl Pts',(-3.67325664837305,1.41034700249021,305.273002391267));
#6848=CARTESIAN_POINT('Ctrl Pts',(-3.71325573030816,1.30141757231233,305.278876436849));
#6849=CARTESIAN_POINT('Ctrl Pts',(-3.7483918586729,1.19081798518276,305.284750482431));
#6850=CARTESIAN_POINT('Ctrl Pts',(-3.78349289082057,1.08032887200973,305.29061866064));
#6851=CARTESIAN_POINT('Ctrl Pts',(-3.81374050809356,0.968173310775371,305.296486838848));
#6852=CARTESIAN_POINT('Ctrl Pts',(-3.83898167650097,0.854815001909668,305.302355017057));
#6853=CARTESIAN_POINT('Ctrl Pts',(-3.86470834323288,0.739276315807282,305.308336066058));
#6854=CARTESIAN_POINT('Ctrl Pts',(-3.88523380992108,0.622488536375575,305.31431711506));
#6855=CARTESIAN_POINT('Ctrl Pts',(-3.90044940169039,0.504958874417568,305.320298164061));
#6856=CARTESIAN_POINT('Ctrl Pts',(-3.91536143074368,0.389774019282671,305.326159886552));
#6857=CARTESIAN_POINT('Ctrl Pts',(-3.92517343842528,0.273877036136198,305.332021609042));
#6858=CARTESIAN_POINT('Ctrl Pts',(-3.92983491896867,0.157754586793943,305.337883331532));
#6859=CARTESIAN_POINT('Ctrl Pts',(-3.93449575500278,0.0416481928647091,
305.343744243564));
#6860=CARTESIAN_POINT('Ctrl Pts',(-3.93400746358965,-0.0746831938899506,
305.349605155597));
#6861=CARTESIAN_POINT('Ctrl Pts',(-3.9283715936104,-0.190750157312963,305.355466067629));
#6862=CARTESIAN_POINT('Ctrl Pts',(-3.92273515073891,-0.306828919067288,
305.361327575429));
#6863=CARTESIAN_POINT('Ctrl Pts',(-3.91195010908134,-0.4226427927254,305.367189083229));
#6864=CARTESIAN_POINT('Ctrl Pts',(-3.89607005488542,-0.537705428115716,
305.37305059103));
#6865=CARTESIAN_POINT('Ctrl Pts',(-3.87962298375207,-0.65687651693619,305.379121391201));
#6866=CARTESIAN_POINT('Ctrl Pts',(-3.85771031474405,-0.77524124443046,305.385192191373));
#6867=CARTESIAN_POINT('Ctrl Pts',(-3.83044950539371,-0.892269906826998,
305.391262991545));
#6868=CARTESIAN_POINT('Ctrl Pts',(-3.80408971790723,-1.00543054820616,305.397133140165));
#6869=CARTESIAN_POINT('Ctrl Pts',(-3.77272990870503,-1.11734166185968,305.403003288786));
#6870=CARTESIAN_POINT('Ctrl Pts',(-3.73652702454398,-1.22754013981316,305.408873437406));
#6871=CARTESIAN_POINT('Ctrl Pts',(-3.69846792719186,-1.34338877170195,305.415044563353));
#6872=CARTESIAN_POINT('Ctrl Pts',(-3.65505614719676,-1.4573439958255,305.421215689301));
#6873=CARTESIAN_POINT('Ctrl Pts',(-3.60653060591148,-1.56889323684684,305.427386815248));
#6874=CARTESIAN_POINT('Ctrl Pts',(-3.5580050646262,-1.68044247786819,305.433557941195));
#6875=CARTESIAN_POINT('Ctrl Pts',(-3.50436605532843,-1.78958529909671,305.439729067143));
#6876=CARTESIAN_POINT('Ctrl Pts',(-3.44590658322787,-1.89584198172391,305.44590019309));
#6877=CARTESIAN_POINT('Ctrl Pts',(-3.39018977251935,-1.99711356799945,305.451781796942));
#6878=CARTESIAN_POINT('Ctrl Pts',(-3.32991504359332,-2.09609001318154,305.457663400793));
#6879=CARTESIAN_POINT('Ctrl Pts',(-3.2652962449239,-2.19233424296704,305.463545004645));
#6880=CARTESIAN_POINT('Ctrl Pts',(-3.20075911357354,-2.28845683619503,305.469419175136));
#6881=CARTESIAN_POINT('Ctrl Pts',(-3.13188905916723,-2.38185374270415,305.475293345627));
#6882=CARTESIAN_POINT('Ctrl Pts',(-3.05894582471176,-2.47211234402453,305.481167516118));
#6883=CARTESIAN_POINT('Ctrl Pts',(-2.98607545371347,-2.56228078545853,305.487035818863));
#6884=CARTESIAN_POINT('Ctrl Pts',(-2.90914025381092,-2.64931683929501,305.492904121609));
#6885=CARTESIAN_POINT('Ctrl Pts',(-2.82844290172965,-2.73283730793752,305.498772424354));
#6886=CARTESIAN_POINT('Ctrl Pts',(-2.74619577515903,-2.81796176838771,305.504753426533));
#6887=CARTESIAN_POINT('Ctrl Pts',(-2.6600407439559,-2.89943385647308,305.510734428712));
#6888=CARTESIAN_POINT('Ctrl Pts',(-2.57034120387822,-2.9768834534872,305.516715430891));
#6889=CARTESIAN_POINT('Ctrl Pts',(-2.48242870808692,-3.05279005641566,305.522577276207));
#6890=CARTESIAN_POINT('Ctrl Pts',(-2.39111195352829,-3.12483268079289,305.528439121524));
#6891=CARTESIAN_POINT('Ctrl Pts',(-2.29676926524284,-3.19270104178826,305.53430096684));
#6892=CARTESIAN_POINT('Ctrl Pts',(-2.20243963450449,-3.26056000942909,305.540162000845));
#6893=CARTESIAN_POINT('Ctrl Pts',(-2.10508523711594,-3.32424562222826,305.54602303485));
#6894=CARTESIAN_POINT('Ctrl Pts',(-2.00511537627614,-3.38348951938986,305.551884068855));
#6895=CARTESIAN_POINT('Ctrl Pts',(-1.90513537045563,-3.44273942864538,305.557745697639));
#6896=CARTESIAN_POINT('Ctrl Pts',(-1.80253972781519,-3.49754651627313,305.563607326424));
#6897=CARTESIAN_POINT('Ctrl Pts',(-1.69776386313948,-3.54768753768109,305.569468955209));
#6898=CARTESIAN_POINT('Ctrl Pts',(-1.58925218591523,-3.5996163511302,305.575539581996));
#6899=CARTESIAN_POINT('Ctrl Pts',(-1.4784023406849,-3.64653993997509,305.581610208782));
#6900=CARTESIAN_POINT('Ctrl Pts',(-1.36572103949845,-3.68826450275347,305.587680835569));
#6901=CARTESIAN_POINT('Ctrl Pts',(-1.25675877934779,-3.72861194830352,305.593551101605));
#6902=CARTESIAN_POINT('Ctrl Pts',(-1.14608446715669,-3.76409807133267,305.599421367641));
#6903=CARTESIAN_POINT('Ctrl Pts',(-1.03417106821957,-3.79459868782689,305.605291633676));
#6904=CARTESIAN_POINT('Ctrl Pts',(-0.916528017715103,-3.82666085018391,
305.611462440839));
#6905=CARTESIAN_POINT('Ctrl Pts',(-0.797516163788637,-3.85321339208828,
305.617633248001));
#6906=CARTESIAN_POINT('Ctrl Pts',(-0.677694801964336,-3.87417329960735,
305.623804055163));
#6907=CARTESIAN_POINT('Ctrl Pts',(-0.557873440140036,-3.89513320712642,
305.629974862325));
#6908=CARTESIAN_POINT('Ctrl Pts',(-0.437243096222677,-3.91050048438429,
305.636145669488));
#6909=CARTESIAN_POINT('Ctrl Pts',(-0.31636544559735,-3.92025533668816,305.64231647665));
#6910=CARTESIAN_POINT('Ctrl Pts',(-0.201152959526222,-3.92955300899872,
305.648198077017));
#6911=CARTESIAN_POINT('Ctrl Pts',(-0.0853447024464972,-3.93378238806566,
305.654079677383));
#6912=CARTESIAN_POINT('Ctrl Pts',(0.0305767478697531,-3.93288114014264,
305.65996127775));
#6913=CARTESIAN_POINT('Ctrl Pts',(0.146351717495847,-3.93198103105474,305.665835446007));
#6914=CARTESIAN_POINT('Ctrl Pts',(0.262239187654835,-3.92596319218012,305.671709614265));
#6915=CARTESIAN_POINT('Ctrl Pts',(0.377751705307836,-3.91481706458131,305.677583782522));
#6916=CARTESIAN_POINT('Ctrl Pts',(0.493148861045902,-3.90368206857802,305.68345208427));
#6917=CARTESIAN_POINT('Ctrl Pts',(0.6081714015849,-3.88742901138595,305.689320386017));
#6918=CARTESIAN_POINT('Ctrl Pts',(0.722332773385868,-3.86609937333389,305.695188687765));
#6919=CARTESIAN_POINT('Ctrl Pts',(0.838686624754658,-3.84436009763574,305.701169690784));
#6920=CARTESIAN_POINT('Ctrl Pts',(0.954145453613655,-3.81734723856571,305.707150693802));
#6921=CARTESIAN_POINT('Ctrl Pts',(1.06820016894353,-3.78516015500917,305.713131696821));
#6922=CARTESIAN_POINT('Ctrl Pts',(1.17998264550101,-3.75361431402656,305.718993544161));
#6923=CARTESIAN_POINT('Ctrl Pts',(1.29041602344907,-3.71709862327207,305.724855391501));
#6924=CARTESIAN_POINT('Ctrl Pts',(1.39903292108217,-3.67575786549227,305.730717238842));
#6925=CARTESIAN_POINT('Ctrl Pts',(1.50763480623193,-3.63442282162486,305.736578275987));
#6926=CARTESIAN_POINT('Ctrl Pts',(1.61442032559998,-3.5882641834342,305.742439313132));
#6927=CARTESIAN_POINT('Ctrl Pts',(1.71894001818385,-3.53747568385793,305.748300350277));
#6928=CARTESIAN_POINT('Ctrl Pts',(1.82347033721226,-3.48668202065018,305.75416198331));
#6929=CARTESIAN_POINT('Ctrl Pts',(1.92573400112539,-3.43125774028996,305.760023616343));
#6930=CARTESIAN_POINT('Ctrl Pts',(2.02530481479121,-3.37144322318848,305.765885249376));
#6931=CARTESIAN_POINT('Ctrl Pts',(2.12842576372008,-3.30949605678359,305.771955875278));
#6932=CARTESIAN_POINT('Ctrl Pts',(2.22865784474234,-3.24283999139748,305.778026501181));
#6933=CARTESIAN_POINT('Ctrl Pts',(2.3255601554877,-3.17179112855939,305.784097127084));
#6934=CARTESIAN_POINT('Ctrl Pts',(2.41926433453014,-3.10308713880998,305.789967400065));
#6935=CARTESIAN_POINT('Ctrl Pts',(2.50985477757929,-3.0302760439035,305.795837673045));
#6936=CARTESIAN_POINT('Ctrl Pts',(2.59696727228205,-2.9536841379362,305.801707946025));
#6937=CARTESIAN_POINT('Ctrl Pts',(2.68853950240764,-2.87317109944583,305.807878748389));
#6938=CARTESIAN_POINT('Ctrl Pts',(2.77626787070472,-2.78848025421607,305.814049550754));
#6939=CARTESIAN_POINT('Ctrl Pts',(2.85977496296949,-2.70003262224234,305.820220353118));
#6940=CARTESIAN_POINT('Ctrl Pts',(2.94328205523427,-2.6115849902686,305.826391155482));
#6941=CARTESIAN_POINT('Ctrl Pts',(3.02256758523281,-2.51938101262983,305.832561957846));
#6942=CARTESIAN_POINT('Ctrl Pts',(3.09730558680027,-2.42387852459149,305.83873276021));
#6943=CARTESIAN_POINT('Ctrl Pts',(3.16841691842985,-2.33301030553409,305.844604123695));
#6944=CARTESIAN_POINT('Ctrl Pts',(3.23564594367985,-2.23885685477851,305.85047548718));
#6945=CARTESIAN_POINT('Ctrl Pts',(3.29867404781631,-2.14178395882105,305.856346850665));
#6946=CARTESIAN_POINT('Ctrl Pts',(3.36162482580041,-2.04483015693512,305.862211010856));
#6947=CARTESIAN_POINT('Ctrl Pts',(3.42038470572425,-1.9449643728561,305.868075171047));
#6948=CARTESIAN_POINT('Ctrl Pts',(3.47467530420241,-1.84258528442129,305.873939331238));
#6949=CARTESIAN_POINT('Ctrl Pts',(3.52891241516199,-1.74030706065825,305.879797714013));
#6950=CARTESIAN_POINT('Ctrl Pts',(3.57868880782915,-1.63552081851714,305.885656096788));
#6951=CARTESIAN_POINT('Ctrl Pts',(3.62376980907873,-1.52865345020038,305.891514479563));
#6952=CARTESIAN_POINT('Ctrl Pts',(3.66881728756418,-1.42186554971887,305.897368505976));
#6953=CARTESIAN_POINT('Ctrl Pts',(3.70917615958446,-1.31299998020192,305.903222532388));
#6954=CARTESIAN_POINT('Ctrl Pts',(3.74465838158372,-1.20250680049421,305.909076558801));
#6955=CARTESIAN_POINT('Ctrl Pts',(3.78012564973577,-1.09206018771589,305.914928118057));
#6956=CARTESIAN_POINT('Ctrl Pts',(3.81072022758069,-0.979987720829308,305.920779677312));
#6957=CARTESIAN_POINT('Ctrl Pts',(3.83630298977896,-0.866757388554042,305.926631236567));
#6958=CARTESIAN_POINT('Ctrl Pts',(3.86187930737916,-0.753555580328454,305.932481321746));
#6959=CARTESIAN_POINT('Ctrl Pts',(3.88244623339217,-0.639196890247835,305.938331406925));
#6960=CARTESIAN_POINT('Ctrl Pts',(3.89791529686582,-0.524161557594061,305.944181492104));
#6961=CARTESIAN_POINT('Ctrl Pts',(3.91338784716017,-0.409100295278861,305.950032895928));
#6962=CARTESIAN_POINT('Ctrl Pts',(3.92376018391224,-0.293362494978405,305.955884299752));
#6963=CARTESIAN_POINT('Ctrl Pts',(3.92899551174811,-0.177435252030728,305.961735703575));
#6964=CARTESIAN_POINT('Ctrl Pts',(3.93170970586436,-0.117334136955256,305.964769295039));
#6965=CARTESIAN_POINT('Ctrl Pts',(3.93304403689269,-0.0571821728465312,
305.967802886502));
#6966=CARTESIAN_POINT('Ctrl Pts',(3.93299889167956,0.00295263396733381,
305.970836477965));
#6967=CARTESIAN_POINT('',(1.74869860048799,-3.52285994678348,306.999909416517));
#6968=CARTESIAN_POINT('Ctrl Pts',(3.93299889167903,0.0029526346725509,305.970836478001));
#6969=CARTESIAN_POINT('Ctrl Pts',(3.93289712360706,0.138510791597115,305.977674914663));
#6970=CARTESIAN_POINT('Ctrl Pts',(3.92578303440299,0.273785134511518,305.984513351326));
#6971=CARTESIAN_POINT('Ctrl Pts',(3.91176797889345,0.408117972287244,305.991351787988));
#6972=CARTESIAN_POINT('Ctrl Pts',(3.89766593117476,0.543284621267804,305.998232671198));
#6973=CARTESIAN_POINT('Ctrl Pts',(3.87657709023588,0.677497944107449,306.005113554408));
#6974=CARTESIAN_POINT('Ctrl Pts',(3.84866405746424,0.810107383488669,306.011994437617));
#6975=CARTESIAN_POINT('Ctrl Pts',(3.82056658327726,0.943593068489225,306.018920787754));
#6976=CARTESIAN_POINT('Ctrl Pts',(3.78555451165409,1.07545351169804,306.025847137892));
#6977=CARTESIAN_POINT('Ctrl Pts',(3.74384194762071,1.20504625273704,306.032773488029));
#6978=CARTESIAN_POINT('Ctrl Pts',(3.73907317719976,1.21986188549801,306.033565339942));
#6979=CARTESIAN_POINT('Ctrl Pts',(3.73421688150865,1.23464790254472,306.034357191856));
#6980=CARTESIAN_POINT('Ctrl Pts',(3.72927341967739,1.24940336212437,306.03514904377));
#6981=CARTESIAN_POINT('Ctrl Pts',(3.69255031001881,1.35901609480088,306.041031412373));
#6982=CARTESIAN_POINT('Ctrl Pts',(3.65093134138518,1.46718473829337,306.046913780975));
#6983=CARTESIAN_POINT('Ctrl Pts',(3.60454887307558,1.57344094951465,306.052796149578));
#6984=CARTESIAN_POINT('Ctrl Pts',(3.55822503132245,1.67956285490887,306.058671082978));
#6985=CARTESIAN_POINT('Ctrl Pts',(3.50714982803897,1.78377676160783,306.064546016379));
#6986=CARTESIAN_POINT('Ctrl Pts',(3.45150514742175,1.88563019102929,306.07042094978));
#6987=CARTESIAN_POINT('Ctrl Pts',(3.39591606944379,1.9873818439749,306.076290012685));
#6988=CARTESIAN_POINT('Ctrl Pts',(3.33576679346814,2.08677735246546,306.082159075591));
#6989=CARTESIAN_POINT('Ctrl Pts',(3.27128670288703,2.18338551509221,306.088028138497));
#6990=CARTESIAN_POINT('Ctrl Pts',(3.20557994039594,2.2818315554003,306.094008854699));
#6991=CARTESIAN_POINT('Ctrl Pts',(3.13537607156481,2.37738271336941,306.0999895709));
#6992=CARTESIAN_POINT('Ctrl Pts',(3.06096640292507,2.46961002592797,306.105970287102));
#6993=CARTESIAN_POINT('Ctrl Pts',(2.98802636484449,2.56001579997679,306.111832880975));
#6994=CARTESIAN_POINT('Ctrl Pts',(2.91104540726783,2.64722748579805,306.117695474848));
#6995=CARTESIAN_POINT('Ctrl Pts',(2.83034036601032,2.73087209743199,306.123558068721));
#6996=CARTESIAN_POINT('Ctrl Pts',(2.74964657103553,2.81450505315279,306.12941984564));
#6997=CARTESIAN_POINT('Ctrl Pts',(2.66523001020445,2.8945716270458,306.135281622558));
#6998=CARTESIAN_POINT('Ctrl Pts',(2.57744549293198,2.97073454400837,306.141143399476));
#6999=CARTESIAN_POINT('Ctrl Pts',(2.48965216515674,3.04690510507051,306.147005764712));
#7000=CARTESIAN_POINT('Ctrl Pts',(2.39849051993202,3.11917096056775,306.152868129949));
#7001=CARTESIAN_POINT('Ctrl Pts',(2.30434912397615,3.18723455597958,306.158730495185));
#7002=CARTESIAN_POINT('Ctrl Pts',(2.20688031948798,3.25770384535646,306.16480006453));
#7003=CARTESIAN_POINT('Ctrl Pts',(2.10621761237537,3.32366803967249,306.170869633876));
#7004=CARTESIAN_POINT('Ctrl Pts',(2.00282457289611,3.38484604231913,306.176939203221));
#7005=CARTESIAN_POINT('Ctrl Pts',(1.9028144410297,3.44402236736799,306.18281018287));
#7006=CARTESIAN_POINT('Ctrl Pts',(1.8002502481252,3.49872065916166,306.188681162519));
#7007=CARTESIAN_POINT('Ctrl Pts',(1.69557521418941,3.54873409725588,306.194552142168));
#7008=CARTESIAN_POINT('Ctrl Pts',(1.58558912882462,3.60128514085041,306.200721006362));
#7009=CARTESIAN_POINT('Ctrl Pts',(1.47327286760583,3.64866324838575,306.206889870556));
#7010=CARTESIAN_POINT('Ctrl Pts',(1.35916126896394,3.69068687982987,306.21305873475));
#7011=CARTESIAN_POINT('Ctrl Pts',(1.24504967032204,3.73271051127399,306.219227598944));
#7012=CARTESIAN_POINT('Ctrl Pts',(1.12914325102822,3.76937957672615,306.225396463137));
#7013=CARTESIAN_POINT('Ctrl Pts',(1.01199048658119,3.80057420070562,306.231565327331));
#7014=CARTESIAN_POINT('Ctrl Pts',(0.900289528946039,3.83031715545383,306.237447118011));
#7015=CARTESIAN_POINT('Ctrl Pts',(0.787096575424546,3.85517935422195,306.24332890869));
#7016=CARTESIAN_POINT('Ctrl Pts',(0.672875349500288,3.87501325985278,306.249210699369));
#7017=CARTESIAN_POINT('Ctrl Pts',(0.558798290772029,3.89482213162027,306.255085066198));
#7018=CARTESIAN_POINT('Ctrl Pts',(0.443695943088427,3.90961526284367,306.260959433027));
#7019=CARTESIAN_POINT('Ctrl Pts',(0.328046073160477,3.91929518840875,306.266833799856));
#7020=CARTESIAN_POINT('Ctrl Pts',(0.212511542925758,3.92896546001014,306.272702308074));
#7021=CARTESIAN_POINT('Ctrl Pts',(0.0964309847241987,3.93353263604942,306.278570816291));
#7022=CARTESIAN_POINT('Ctrl Pts',(-0.0197094256938501,3.93295061481057,
306.284439324509));
#7023=CARTESIAN_POINT('Ctrl Pts',(-0.138074685903231,3.93235744405169,306.290420253108));
#7024=CARTESIAN_POINT('Ctrl Pts',(-0.256501686965844,3.9264156878078,306.296401181707));
#7025=CARTESIAN_POINT('Ctrl Pts',(-0.374471814396688,3.91513216382569,306.302382110306));
#7026=CARTESIAN_POINT('Ctrl Pts',(-0.490097563316956,3.90407287331458,306.308244182032));
#7027=CARTESIAN_POINT('Ctrl Pts',(-0.605284001584659,3.88788220695453,306.314106253758));
#7028=CARTESIAN_POINT('Ctrl Pts',(-0.719545364824838,3.86661912631165,306.319968325485));
#7029=CARTESIAN_POINT('Ctrl Pts',(-0.83379105761463,3.84535896180807,306.325829593253));
#7030=CARTESIAN_POINT('Ctrl Pts',(-0.94711152298397,3.81902784179355,306.331690861021));
#7031=CARTESIAN_POINT('Ctrl Pts',(-1.05902988500892,3.78773609200245,306.337552128789));
#7032=CARTESIAN_POINT('Ctrl Pts',(-1.1709597387215,3.75644112919958,306.343413998388));
#7033=CARTESIAN_POINT('Ctrl Pts',(-1.28148680634442,3.72018463492664,306.349275867987));
#7034=CARTESIAN_POINT('Ctrl Pts',(-1.39014877040593,3.67912698831379,306.355137737585));
#7035=CARTESIAN_POINT('Ctrl Pts',(-1.50267484833663,3.63660929610832,306.361208060361));
#7036=CARTESIAN_POINT('Ctrl Pts',(-1.61320025723283,3.58894279412773,306.367278383136));
#7037=CARTESIAN_POINT('Ctrl Pts',(-1.72123481044774,3.5363596716543,306.373348705912));
#7038=CARTESIAN_POINT('Ctrl Pts',(-1.82571347588474,3.48550728880967,306.37921922792));
#7039=CARTESIAN_POINT('Ctrl Pts',(-1.92786233770892,3.43005710205278,306.385089749929));
#7040=CARTESIAN_POINT('Ctrl Pts',(-2.02726471187947,3.37026509164609,306.390960271938));
#7041=CARTESIAN_POINT('Ctrl Pts',(-2.13174176353459,3.30742058705604,306.397130495097));
#7042=CARTESIAN_POINT('Ctrl Pts',(-2.23318405934418,3.23977953541925,306.403300718256));
#7043=CARTESIAN_POINT('Ctrl Pts',(-2.33114517600648,3.16768861607035,306.409470941414));
#7044=CARTESIAN_POINT('Ctrl Pts',(-2.4291062926688,3.09559769672145,306.415641164573));
#7045=CARTESIAN_POINT('Ctrl Pts',(-2.52358587003434,3.01905729220659,306.421811387732));
#7046=CARTESIAN_POINT('Ctrl Pts',(-2.61418150222925,2.93845947281946,306.427981610891));
#7047=CARTESIAN_POINT('Ctrl Pts',(-2.70047380925804,2.86169007888839,306.433858746227));
#7048=CARTESIAN_POINT('Ctrl Pts',(-2.78352190916399,2.78099146830398,306.439735881563));
#7049=CARTESIAN_POINT('Ctrl Pts',(-2.86294739944237,2.69666853506807,306.445613016899));
#7050=CARTESIAN_POINT('Ctrl Pts',(-2.94227227116643,2.61245242461171,306.451482706906));
#7051=CARTESIAN_POINT('Ctrl Pts',(-3.01798337984358,2.5246214204154,306.457352396914));
#7052=CARTESIAN_POINT('Ctrl Pts',(-3.08973632633246,2.43351976234868,306.463222086922));
#7053=CARTESIAN_POINT('Ctrl Pts',(-3.16141746537064,2.34250927514171,306.46908590278));
#7054=CARTESIAN_POINT('Ctrl Pts',(-3.22914806794749,2.24823496718569,306.474949718639));
#7055=CARTESIAN_POINT('Ctrl Pts',(-3.29262193170535,2.15107643166227,306.480813534498));
#7056=CARTESIAN_POINT('Ctrl Pts',(-3.35738247842609,2.05194838892828,306.486796216163));
#7057=CARTESIAN_POINT('Ctrl Pts',(-3.41771153372696,1.94981823222956,306.492778897828));
#7058=CARTESIAN_POINT('Ctrl Pts',(-3.47332827271481,1.8451232235165,306.498761579492));
#7059=CARTESIAN_POINT('Ctrl Pts',(-3.52778009104181,1.74262110458731,306.504618950871));
#7060=CARTESIAN_POINT('Ctrl Pts',(-3.5777148678531,1.63766091082651,306.510476322249));
#7061=CARTESIAN_POINT('Ctrl Pts',(-3.6229143175292,1.53067986458368,306.516333693628));
#7062=CARTESIAN_POINT('Ctrl Pts',(-3.66810760446552,1.42371340472087,306.52219026638));
#7063=CARTESIAN_POINT('Ctrl Pts',(-3.70856668768278,1.31472702018849,306.528046839133));
#7064=CARTESIAN_POINT('Ctrl Pts',(-3.74412103833895,1.20417882819275,306.533903411886));
#7065=CARTESIAN_POINT('Ctrl Pts',(-3.77967910680249,1.09361907651796,306.539760597042));
#7066=CARTESIAN_POINT('Ctrl Pts',(-3.81033129686339,0.981497585426619,306.545617782198));
#7067=CARTESIAN_POINT('Ctrl Pts',(-3.83595687098442,0.868287903835731,306.551474967354));
#7068=CARTESIAN_POINT('Ctrl Pts',(-3.86254375848059,0.750831293743016,306.557551877945));
#7069=CARTESIAN_POINT('Ctrl Pts',(-3.88371939351089,0.632203717114054,306.563628788537));
#7070=CARTESIAN_POINT('Ctrl Pts',(-3.89940725364546,0.512944509881105,306.569705699128));
#7071=CARTESIAN_POINT('Ctrl Pts',(-3.91455039755654,0.397826238659985,306.575571606322));
#7072=CARTESIAN_POINT('Ctrl Pts',(-3.92458054935207,0.282119893340267,306.581437513516));
#7073=CARTESIAN_POINT('Ctrl Pts',(-3.92948199990403,0.166313596648635,306.58730342071));
#7074=CARTESIAN_POINT('Ctrl Pts',(-3.93438684269401,0.0504271517399519,
306.593173387631));
#7075=CARTESIAN_POINT('Ctrl Pts',(-3.93415591723505,-0.0655589709785255,
306.599043354553));
#7076=CARTESIAN_POINT('Ctrl Pts',(-3.9288255811531,-0.181158916084803,306.604913321474));
#7077=CARTESIAN_POINT('Ctrl Pts',(-3.92348777435322,-0.296920879977343,
306.610791515432));
#7078=CARTESIAN_POINT('Ctrl Pts',(-3.91303633391891,-0.412295177475449,
306.616669709389));
#7079=CARTESIAN_POINT('Ctrl Pts',(-3.89755913823653,-0.526803344663774,
306.622547903347));
#7080=CARTESIAN_POINT('Ctrl Pts',(-3.89593547204797,-0.538816053115138,
306.623164567048));
#7081=CARTESIAN_POINT('Ctrl Pts',(-3.89425654079538,-0.550819241196603,
306.62378123075));
#7082=CARTESIAN_POINT('Ctrl Pts',(-3.8925224779634,-0.562812365313372,306.624397894451));
#7083=CARTESIAN_POINT('Ctrl Pts',(-3.87595825681001,-0.677373819793196,
306.630288427217));
#7084=CARTESIAN_POINT('Ctrl Pts',(-3.85430596616859,-0.791385236060905,
306.636178959982));
#7085=CARTESIAN_POINT('Ctrl Pts',(-3.82761282970756,-0.904361114742364,
306.642069492747));
#7086=CARTESIAN_POINT('Ctrl Pts',(-3.80095342830771,-1.01719421334313,306.647952580997));
#7087=CARTESIAN_POINT('Ctrl Pts',(-3.76926594581306,-1.12899398134805,306.653835669246));
#7088=CARTESIAN_POINT('Ctrl Pts',(-3.73264916008286,-1.23928174671165,306.659718757496));
#7089=CARTESIAN_POINT('Ctrl Pts',(-3.69606903310955,-1.34945909789509,306.665595955913));
#7090=CARTESIAN_POINT('Ctrl Pts',(-3.65456954905768,-1.45812707048796,306.671473154331));
#7091=CARTESIAN_POINT('Ctrl Pts',(-3.60830001024323,-1.56481948993444,306.677350352749));
#7092=CARTESIAN_POINT('Ctrl Pts',(-3.56123957033372,-1.67333563949662,306.683328012135));
#7093=CARTESIAN_POINT('Ctrl Pts',(-3.50924459489837,-1.77980765438534,306.689305671521));
#7094=CARTESIAN_POINT('Ctrl Pts',(-3.45252449845199,-1.88376314529955,306.695283330907));
#7095=CARTESIAN_POINT('Ctrl Pts',(-3.39681997791561,-1.98585730841461,306.701153960029));
#7096=CARTESIAN_POINT('Ctrl Pts',(-3.3365583500657,-2.08552394555246,306.707024589151));
#7097=CARTESIAN_POINT('Ctrl Pts',(-3.27198525238109,-2.18233854115274,306.712895218274));
#7098=CARTESIAN_POINT('Ctrl Pts',(-3.20742171169672,-2.27913880792032,306.718764978527));
#7099=CARTESIAN_POINT('Ctrl Pts',(-3.13854819798794,-2.37308753135952,306.724634738779));
#7100=CARTESIAN_POINT('Ctrl Pts',(-3.06565409669719,-2.46378853788301,306.730504499032));
#7101=CARTESIAN_POINT('Ctrl Pts',(-2.99275344601327,-2.55449769371547,306.736374786671));
#7102=CARTESIAN_POINT('Ctrl Pts',(-2.91583174676212,-2.6419582326833,306.742245074311));
#7103=CARTESIAN_POINT('Ctrl Pts',(-2.83521871242445,-2.7258070094411,306.74811536195));
#7104=CARTESIAN_POINT('Ctrl Pts',(-2.75202471757622,-2.81234034439038,306.754173596622));
#7105=CARTESIAN_POINT('Ctrl Pts',(-2.66489936305495,-2.89502641257054,306.760231831293));
#7106=CARTESIAN_POINT('Ctrl Pts',(-2.57424524384319,-2.97350810063647,306.766290065965));
#7107=CARTESIAN_POINT('Ctrl Pts',(-2.48627798136556,-3.04966370518938,306.77216874334));
#7108=CARTESIAN_POINT('Ctrl Pts',(-2.3949885424225,-3.12186042568071,306.778047420714));
#7109=CARTESIAN_POINT('Ctrl Pts',(-2.30077659906905,-3.18981442111861,306.783926098089));
#7110=CARTESIAN_POINT('Ctrl Pts',(-2.20224826594791,-3.26088177904689,306.790074111409));
#7111=CARTESIAN_POINT('Ctrl Pts',(-2.10052370290793,-3.32730812825324,306.79622212473));
#7112=CARTESIAN_POINT('Ctrl Pts',(-1.9960904717941,-3.38882159878811,306.80237013805));
#7113=CARTESIAN_POINT('Ctrl Pts',(-1.89165724068026,-3.45033506932299,306.80851815137));
#7114=CARTESIAN_POINT('Ctrl Pts',(-1.78451582035214,-3.50693548322745,306.814666164691));
#7115=CARTESIAN_POINT('Ctrl Pts',(-1.67517794328877,-3.55840805112607,306.820814178011));
#7116=CARTESIAN_POINT('Ctrl Pts',(-1.57185477980409,-3.60704909566439,306.82662398704));
#7117=CARTESIAN_POINT('Ctrl Pts',(-1.46622651812633,-3.65127302112401,306.832433796069));
#7118=CARTESIAN_POINT('Ctrl Pts',(-1.35871205605211,-3.69085227945236,306.838243605099));
#7119=CARTESIAN_POINT('Ctrl Pts',(-1.25133244258961,-3.73038189601218,306.844046127251));
#7120=CARTESIAN_POINT('Ctrl Pts',(-1.14207172465273,-3.76527828081848,306.849848649403));
#7121=CARTESIAN_POINT('Ctrl Pts',(-1.03137203581375,-3.79536042079555,306.855651171555));
#7122=CARTESIAN_POINT('Ctrl Pts',(-0.916699611110698,-3.82652213378325,
306.861661931762));
#7123=CARTESIAN_POINT('Ctrl Pts',(-0.800483396006691,-3.8525173513266,306.867672691969));
#7124=CARTESIAN_POINT('Ctrl Pts',(-0.683236457770158,-3.87319983253817,
306.873683452175));
#7125=CARTESIAN_POINT('Ctrl Pts',(-0.570238634224967,-3.89313276552194,
306.879476378041));
#7126=CARTESIAN_POINT('Ctrl Pts',(-0.456283954458853,-3.90813126031801,
306.885269303907));
#7127=CARTESIAN_POINT('Ctrl Pts',(-0.341844866762429,-3.91811575723181,
306.891062229773));
#7128=CARTESIAN_POINT('Ctrl Pts',(-0.227442596936768,-3.92809704188724,
306.896853291912));
#7129=CARTESIAN_POINT('Ctrl Pts',(-0.112556649794527,-3.93306749798193,
306.902644354051));
#7130=CARTESIAN_POINT('Ctrl Pts',(0.0023343352513748,-3.93299930725635,
306.908435416191));
#7131=CARTESIAN_POINT('Ctrl Pts',(0.117217598358397,-3.93293112111394,306.914226089107));
#7132=CARTESIAN_POINT('Ctrl Pts',(0.232105475818189,-3.92782496247348,306.920016762023));
#7133=CARTESIAN_POINT('Ctrl Pts',(0.346519097391488,-3.91770513376683,306.925807434939));
#7134=CARTESIAN_POINT('Ctrl Pts',(0.46095415010996,-3.90758340948591,306.931599192522));
#7135=CARTESIAN_POINT('Ctrl Pts',(0.574914349355133,-3.89244618727576,306.937390950106));
#7136=CARTESIAN_POINT('Ctrl Pts',(0.687926557494139,-3.87236956545915,306.94318270769));
#7137=CARTESIAN_POINT('Ctrl Pts',(0.801046495301565,-3.85227380546404,306.948979986306));
#7138=CARTESIAN_POINT('Ctrl Pts',(0.913216221904416,-3.82722932348057,306.954777264923));
#7139=CARTESIAN_POINT('Ctrl Pts',(1.02397351037318,-3.79736319701632,306.96057454354));
#7140=CARTESIAN_POINT('Ctrl Pts',(1.13479391769831,-3.76748005031103,306.966375125935));
#7141=CARTESIAN_POINT('Ctrl Pts',(1.24419988250263,-3.73276991765602,306.972175708331));
#7142=CARTESIAN_POINT('Ctrl Pts',(1.35174671657435,-3.69340896926274,306.977976290726));
#7143=CARTESIAN_POINT('Ctrl Pts',(1.45943800980113,-3.65399515042101,306.983784664585));
#7144=CARTESIAN_POINT('Ctrl Pts',(1.56526480094117,-3.60991821374187,306.989593038445));
#7145=CARTESIAN_POINT('Ctrl Pts',(1.66880475645938,-3.56140136530812,306.995401412304));
#7146=CARTESIAN_POINT('Ctrl Pts',(1.69559128725737,-3.54884970785098,306.996904080375));
#7147=CARTESIAN_POINT('Ctrl Pts',(1.72222490323772,-3.53600112129244,306.998406748446));
#7148=CARTESIAN_POINT('Ctrl Pts',(1.74869860048799,-3.52285994678348,306.999909416517));
#7149=CARTESIAN_POINT('',(-1.74869447533106,-3.52286199445091,307.));
#7150=CARTESIAN_POINT('Origin',(0.,0.,307.));
#7151=CARTESIAN_POINT('',(3.93127820247977,0.00326437435658078,306.154164236595));
#7152=CARTESIAN_POINT('Ctrl Pts',(-1.74869447533129,-3.5228619944508,307.));
#7153=CARTESIAN_POINT('Ctrl Pts',(-2.90806357314774,-2.94736901759987,306.93452790548));
#7154=CARTESIAN_POINT('Ctrl Pts',(-4.59459704467384,-0.57010578582661,306.80358371644));
#7155=CARTESIAN_POINT('Ctrl Pts',(-3.00810365225817,3.52651283114026,306.60716743288));
#7156=CARTESIAN_POINT('Ctrl Pts',(1.28568539453312,4.45038130233524,306.410751149319));
#7157=CARTESIAN_POINT('Ctrl Pts',(3.69704862595707,2.09019977571459,306.259750186429));
#7158=CARTESIAN_POINT('Ctrl Pts',(3.93358950080438,0.400386139161716,306.174221318059));
#7159=CARTESIAN_POINT('Ctrl Pts',(3.93053755798013,0.00326985260832528,
306.154164544208));
#7160=CARTESIAN_POINT('',(3.932998918852,-0.0029162148394918,304.904163521999));
#7161=CARTESIAN_POINT('Ctrl Pts',(3.93299865583244,0.00325164884982929,
306.154163522035));
#7162=CARTESIAN_POINT('Ctrl Pts',(3.93309417218823,-0.11227918374711,306.148332127252));
#7163=CARTESIAN_POINT('Ctrl Pts',(3.9280948765027,-0.227892259450327,306.142500732469));
#7164=CARTESIAN_POINT('Ctrl Pts',(3.91800580906771,-0.34310272530493,306.136669337686));
#7165=CARTESIAN_POINT('Ctrl Pts',(3.9079197792971,-0.458278503044824,306.130839698647));
#7166=CARTESIAN_POINT('Ctrl Pts',(3.89274706022665,-0.573051497308586,306.125010059608));
#7167=CARTESIAN_POINT('Ctrl Pts',(3.87254472272492,-0.686939859445751,306.119180420569));
#7168=CARTESIAN_POINT('Ctrl Pts',(3.85234348722245,-0.800822009188452,306.113351099526));
#7169=CARTESIAN_POINT('Ctrl Pts',(3.82711325170791,-0.913819212630393,306.107521778483));
#7170=CARTESIAN_POINT('Ctrl Pts',(3.79696245960987,-1.02545847322716,306.101692457439));
#7171=CARTESIAN_POINT('Ctrl Pts',(3.76680587879097,-1.13711916770582,306.095862017211));
#7172=CARTESIAN_POINT('Ctrl Pts',(3.73172697215613,-1.24742099899279,306.090031576983));
#7173=CARTESIAN_POINT('Ctrl Pts',(3.69188422433854,-1.35590555500013,306.084201136755));
#7174=CARTESIAN_POINT('Ctrl Pts',(3.65199908332218,-1.46450553997756,306.078364492863));
#7175=CARTESIAN_POINT('Ctrl Pts',(3.6073401226729,-1.57128399664453,306.072527848971));
#7176=CARTESIAN_POINT('Ctrl Pts',(3.55811428393509,-1.67580182075837,306.06669120508));
#7177=CARTESIAN_POINT('Ctrl Pts',(3.50886108750736,-1.78037773156605,306.060851317422));
#7178=CARTESIAN_POINT('Ctrl Pts',(3.45503615222371,-1.88269013933472,306.055011429764));
#7179=CARTESIAN_POINT('Ctrl Pts',(3.39689187124467,-1.98232555728666,306.049171542107));
#7180=CARTESIAN_POINT('Ctrl Pts',(3.3386534669034,-2.08212226402534,306.043322200899));
#7181=CARTESIAN_POINT('Ctrl Pts',(3.27608197580863,-2.17923297481225,306.037472859691));
#7182=CARTESIAN_POINT('Ctrl Pts',(3.20947272689476,-2.27327381001909,306.031623518484));
#7183=CARTESIAN_POINT('Ctrl Pts',(3.15745116982446,-2.34671932630132,306.027055206389));
#7184=CARTESIAN_POINT('Ctrl Pts',(3.10296764191761,-2.4182929457685,306.022486894294));
#7185=CARTESIAN_POINT('Ctrl Pts',(3.04617884903102,-2.48782704779011,306.017918582199));
#7186=CARTESIAN_POINT('Ctrl Pts',(2.97306129458837,-2.57735463293069,306.012036720808));
#7187=CARTESIAN_POINT('Ctrl Pts',(2.89587579309586,-2.66380029440954,306.006154859417));
#7188=CARTESIAN_POINT('Ctrl Pts',(2.81491173847977,-2.74677281633717,306.000272998026));
#7189=CARTESIAN_POINT('Ctrl Pts',(2.73405006001075,-2.82964042248275,305.994398574038));
#7190=CARTESIAN_POINT('Ctrl Pts',(2.64941961592671,-2.90904333128066,305.98852415005));
#7191=CARTESIAN_POINT('Ctrl Pts',(2.56135051466587,-2.98462267984093,305.982649726062));
#7192=CARTESIAN_POINT('Ctrl Pts',(2.47336944781431,-3.0601264788247,305.976781174184));
#7193=CARTESIAN_POINT('Ctrl Pts',(2.38195687220633,-3.13181405399361,305.970912622306));
#7194=CARTESIAN_POINT('Ctrl Pts',(2.28747980121963,-3.19936324274256,305.965044070428));
#7195=CARTESIAN_POINT('Ctrl Pts',(2.19119393685813,-3.2682056820528,305.95906316327));
#7196=CARTESIAN_POINT('Ctrl Pts',(2.09172533096063,-3.33274933108614,305.953082256113));
#7197=CARTESIAN_POINT('Ctrl Pts',(1.98949827718364,-3.39269591992612,305.947101348955));
#7198=CARTESIAN_POINT('Ctrl Pts',(1.88930221312591,-3.45145152359006,305.941239267103));
#7199=CARTESIAN_POINT('Ctrl Pts',(1.78645666748683,-3.50579082792641,305.935377185251));
#7200=CARTESIAN_POINT('Ctrl Pts',(1.68138986744675,-3.55547705851794,305.929515103399));
#7201=CARTESIAN_POINT('Ctrl Pts',(1.57633770137118,-3.60515636868805,305.923653838033));
#7202=CARTESIAN_POINT('Ctrl Pts',(1.46906526829634,-3.65018371799922,305.917792572666));
#7203=CARTESIAN_POINT('Ctrl Pts',(1.36002368258499,-3.6903691661957,305.911931307299));
#7204=CARTESIAN_POINT('Ctrl Pts',(1.25097113359423,-3.730558654725,305.906069452629));
#7205=CARTESIAN_POINT('Ctrl Pts',(1.14014946472176,-3.76590513201227,305.900207597958));
#7206=CARTESIAN_POINT('Ctrl Pts',(1.02802731453032,-3.79626775143424,305.894345743287));
#7207=CARTESIAN_POINT('Ctrl Pts',(0.911918390824577,-3.82770998703133,305.888275456233));
#7208=CARTESIAN_POINT('Ctrl Pts',(0.794415239715369,-3.8538072136957,305.882205169179));
#7209=CARTESIAN_POINT('Ctrl Pts',(0.676051153361322,-3.87446045766876,305.876134882125));
#7210=CARTESIAN_POINT('Ctrl Pts',(0.561583168810041,-3.89443387430944,305.870264406154));
#7211=CARTESIAN_POINT('Ctrl Pts',(0.446310457463014,-3.90931606797126,305.864393930184));
#7212=CARTESIAN_POINT('Ctrl Pts',(0.330720679943943,-3.91907040404449,305.858523454213));
#7213=CARTESIAN_POINT('Ctrl Pts',(0.209229476681172,-3.92932274687273,305.852353261617));
#7214=CARTESIAN_POINT('Ctrl Pts',(0.0873885057713353,-3.93390978712592,
305.846183069022));
#7215=CARTESIAN_POINT('Ctrl Pts',(-0.0342373266273185,-3.93285097676805,
305.840012876426));
#7216=CARTESIAN_POINT('Ctrl Pts',(-0.155863159025963,-3.93179216641018,
305.83384268383));
#7217=CARTESIAN_POINT('Ctrl Pts',(-0.277273336903729,-3.92508760441031,
305.827672491235));
#7218=CARTESIAN_POINT('Ctrl Pts',(-0.397912032186795,-3.912819317914,305.821502298639));
#7219=CARTESIAN_POINT('Ctrl Pts',(-0.512921609468159,-3.90112348151096,
305.815620013187));
#7220=CARTESIAN_POINT('Ctrl Pts',(-0.627599793355764,-3.88433385812013,
305.809737727736));
#7221=CARTESIAN_POINT('Ctrl Pts',(-0.741460588139995,-3.86247656254832,
305.803855442284));
#7222=CARTESIAN_POINT('Ctrl Pts',(-0.855177774889915,-3.84064683470304,
305.797980575922));
#7223=CARTESIAN_POINT('Ctrl Pts',(-0.968079222106158,-3.81376222373203,
305.79210570956));
#7224=CARTESIAN_POINT('Ctrl Pts',(-1.07968351999496,-3.78190064605765,305.786230843198));
#7225=CARTESIAN_POINT('Ctrl Pts',(-1.19117660146453,-3.75007081922663,305.780361831284));
#7226=CARTESIAN_POINT('Ctrl Pts',(-1.30137471136452,-3.71327400422141,305.774492819371));
#7227=CARTESIAN_POINT('Ctrl Pts',(-1.40980675142425,-3.6716391330901,305.768623807457));
#7228=CARTESIAN_POINT('Ctrl Pts',(-1.52030303173504,-3.62921165142789,305.762643066108));
#7229=CARTESIAN_POINT('Ctrl Pts',(-1.62896488516239,-3.58176010348318,305.756662324759));
#7230=CARTESIAN_POINT('Ctrl Pts',(-1.73530976509467,-3.52947432618047,305.75068158341));
#7231=CARTESIAN_POINT('Ctrl Pts',(-1.83955364071031,-3.47822153367103,305.744819000673));
#7232=CARTESIAN_POINT('Ctrl Pts',(-1.9415708682392,-3.42232396481679,305.738956417935));
#7233=CARTESIAN_POINT('Ctrl Pts',(-2.04092790802344,-3.36200866659369,305.733093835198));
#7234=CARTESIAN_POINT('Ctrl Pts',(-2.14027135466279,-3.30170162017227,305.727232054527));
#7235=CARTESIAN_POINT('Ctrl Pts',(-2.23695498551482,-3.23697825992387,305.721370273856));
#7236=CARTESIAN_POINT('Ctrl Pts',(-2.33057174777083,-3.16811052971521,305.715508493186));
#7237=CARTESIAN_POINT('Ctrl Pts',(-2.42419814361127,-3.09923571270845,305.709646109311));
#7238=CARTESIAN_POINT('Ctrl Pts',(-2.51475671185153,-3.02621592187917,305.703783725437));
#7239=CARTESIAN_POINT('Ctrl Pts',(-2.60187172518877,-2.94936476646468,305.697921341562));
#7240=CARTESIAN_POINT('Ctrl Pts',(-2.69206612639077,-2.86979703549896,305.691851731022));
#7241=CARTESIAN_POINT('Ctrl Pts',(-2.7785686586941,-2.78612237288855,305.685782120482));
#7242=CARTESIAN_POINT('Ctrl Pts',(-2.86100315466831,-2.69873117389969,305.679712509941));
#7243=CARTESIAN_POINT('Ctrl Pts',(-2.94074069765388,-2.61419909295975,305.673841474695));
#7244=CARTESIAN_POINT('Ctrl Pts',(-3.01667199864521,-2.52619021322746,305.667970439449));
#7245=CARTESIAN_POINT('Ctrl Pts',(-3.08849782474958,-2.43509141235337,305.662099404203));
#7246=CARTESIAN_POINT('Ctrl Pts',(-3.16396768481436,-2.3393707763798,305.655930506016));
#7247=CARTESIAN_POINT('Ctrl Pts',(-3.23490425767385,-2.24023889389887,305.649761607828));
#7248=CARTESIAN_POINT('Ctrl Pts',(-3.30101282934007,-2.13817756524857,305.643592709641));
#7249=CARTESIAN_POINT('Ctrl Pts',(-3.36712140100628,-2.03611623659827,305.637423811454));
#7250=CARTESIAN_POINT('Ctrl Pts',(-3.42840177023318,-1.93112594615363,305.631254913266));
#7251=CARTESIAN_POINT('Ctrl Pts',(-3.48461637982025,-1.82371535210087,305.625086015079));
#7252=CARTESIAN_POINT('Ctrl Pts',(-3.53820812030988,-1.72131633653185,305.619204946204));
#7253=CARTESIAN_POINT('Ctrl Pts',(-3.58736886382915,-1.61638783416557,305.613323877329));
#7254=CARTESIAN_POINT('Ctrl Pts',(-3.63185255390124,-1.50934953762243,305.607442808454));
#7255=CARTESIAN_POINT('Ctrl Pts',(-3.67627997401797,-1.4024466399223,305.601569178878));
#7256=CARTESIAN_POINT('Ctrl Pts',(-3.71604195049381,-1.29343963291238,305.595695549302));
#7257=CARTESIAN_POINT('Ctrl Pts',(-3.75093817048656,-1.18277294574526,305.589821919726));
#7258=CARTESIAN_POINT('Ctrl Pts',(-3.78579949819037,-1.07221691279875,305.583954163119));
#7259=CARTESIAN_POINT('Ctrl Pts',(-3.81580462436139,-0.960004891458814,
305.578086406511));
#7260=CARTESIAN_POINT('Ctrl Pts',(-3.84080148226255,-0.846600835016009,
305.572218649903));
#7261=CARTESIAN_POINT('Ctrl Pts',(-3.86628163417958,-0.731004202927437,
305.56623744497));
#7262=CARTESIAN_POINT('Ctrl Pts',(-3.88655767673246,-0.614169364116873,
305.560256240037));
#7263=CARTESIAN_POINT('Ctrl Pts',(-3.90152196282265,-0.496603839707777,
305.554275035105));
#7264=CARTESIAN_POINT('Ctrl Pts',(-3.91618623511738,-0.381395345829929,
305.548413745281));
#7265=CARTESIAN_POINT('Ctrl Pts',(-3.92574969970113,-0.265485618831752,
305.542552455457));
#7266=CARTESIAN_POINT('Ctrl Pts',(-3.93016286975356,-0.149361364517402,
305.536691165633));
#7267=CARTESIAN_POINT('Ctrl Pts',(-3.93457542705394,-0.0332532336183861,
305.530830689627));
#7268=CARTESIAN_POINT('Ctrl Pts',(-3.93383909629661,0.0830689538829383,
305.524970213621));
#7269=CARTESIAN_POINT('Ctrl Pts',(-3.92795645087036,0.199115845843437,305.519109737615));
#7270=CARTESIAN_POINT('Ctrl Pts',(-3.92207321030637,0.315174478080568,305.513248668714));
#7271=CARTESIAN_POINT('Ctrl Pts',(-3.91104264093404,0.430957348054308,305.507387599813));
#7272=CARTESIAN_POINT('Ctrl Pts',(-3.89491934697215,0.545978278489179,305.501526530912));
#7273=CARTESIAN_POINT('Ctrl Pts',(-3.87821745047479,0.665126864361013,305.495455130963));
#7274=CARTESIAN_POINT('Ctrl Pts',(-3.8560505118387,0.783457324639823,305.489383731013));
#7275=CARTESIAN_POINT('Ctrl Pts',(-3.82853716399658,0.900439994612101,305.483312331064));
#7276=CARTESIAN_POINT('Ctrl Pts',(-3.80193781613805,1.01353647236053,305.47744262447));
#7277=CARTESIAN_POINT('Ctrl Pts',(-3.77034180769444,1.12537289937087,305.471572917876));
#7278=CARTESIAN_POINT('Ctrl Pts',(-3.73390706277148,1.23548656268909,305.465703211282));
#7279=CARTESIAN_POINT('Ctrl Pts',(-3.69559437577795,1.35127577228398,305.459530964655));
#7280=CARTESIAN_POINT('Ctrl Pts',(-3.65193105163972,1.46515940023407,305.453358718027));
#7281=CARTESIAN_POINT('Ctrl Pts',(-3.60315728430097,1.57662506151235,305.4471864714));
#7282=CARTESIAN_POINT('Ctrl Pts',(-3.55438351696223,1.68809072279065,305.441014224773));
#7283=CARTESIAN_POINT('Ctrl Pts',(-3.50049960109066,1.79713798072305,305.434841978145));
#7284=CARTESIAN_POINT('Ctrl Pts',(-3.44179979713586,1.90328746027381,305.428669731518));
#7285=CARTESIAN_POINT('Ctrl Pts',(-3.38586408005447,2.00443851796832,305.422788126847));
#7286=CARTESIAN_POINT('Ctrl Pts',(-3.32537540815491,2.10328456815501,305.416906522177));
#7287=CARTESIAN_POINT('Ctrl Pts',(-3.26054857752851,2.19938900005815,305.411024917506));
#7288=CARTESIAN_POINT('Ctrl Pts',(-3.19580367231638,2.29537197923376,305.405150745759));
#7289=CARTESIAN_POINT('Ctrl Pts',(-3.12673174029815,2.38861989252677,305.399276574013));
#7290=CARTESIAN_POINT('Ctrl Pts',(-3.05359341895139,2.47872068449367,305.393402402266));
#7291=CARTESIAN_POINT('Ctrl Pts',(-2.98052815062925,2.56873148074762,305.38753409784));
#7292=CARTESIAN_POINT('Ctrl Pts',(-2.90340483073116,2.6556010908894,305.381665793415));
#7293=CARTESIAN_POINT('Ctrl Pts',(-2.82252696655011,2.73894697340008,305.375797488989));
#7294=CARTESIAN_POINT('Ctrl Pts',(-2.74009589125975,2.82389346383904,305.369816487279));
#7295=CARTESIAN_POINT('Ctrl Pts',(-2.6537648180976,2.90517912670088,305.36383548557));
#7296=CARTESIAN_POINT('Ctrl Pts',(-2.56389794442153,2.98243463140285,305.35785448386));
#7297=CARTESIAN_POINT('Ctrl Pts',(-2.47582140148219,3.05815104946487,305.351992635858));
#7298=CARTESIAN_POINT('Ctrl Pts',(-2.38434896132091,3.12999612110749,305.346130787856));
#7299=CARTESIAN_POINT('Ctrl Pts',(-2.28985962129222,3.19766038140004,305.340268939854));
#7300=CARTESIAN_POINT('Ctrl Pts',(-2.19538335324821,3.26531528078296,305.334407902801));
#7301=CARTESIAN_POINT('Ctrl Pts',(-2.09789135007304,3.32879027936651,305.328546865747));
#7302=CARTESIAN_POINT('Ctrl Pts',(-1.99779349631778,3.38781790332219,305.322685828694));
#7303=CARTESIAN_POINT('Ctrl Pts',(-1.89768547854856,3.44685152098875,305.316824196506));
#7304=CARTESIAN_POINT('Ctrl Pts',(-1.79497143890895,3.50143665712838,305.310962564319));
#7305=CARTESIAN_POINT('Ctrl Pts',(-1.6900872756754,3.55135101061555,305.305100932131));
#7306=CARTESIAN_POINT('Ctrl Pts',(-1.58146355710944,3.60304501777962,305.29903030845));
#7307=CARTESIAN_POINT('Ctrl Pts',(-1.47051250808343,3.64972875318375,305.292959684769));
#7308=CARTESIAN_POINT('Ctrl Pts',(-1.35774125846145,3.69120951384116,305.286889061088));
#7309=CARTESIAN_POINT('Ctrl Pts',(-1.24869188428673,3.7313212533594,305.281018790824));
#7310=CARTESIAN_POINT('Ctrl Pts',(-1.13794097813819,3.76656796712536,305.27514852056));
#7311=CARTESIAN_POINT('Ctrl Pts',(-1.02596177403602,3.79682649566936,305.269278250296));
#7312=CARTESIAN_POINT('Ctrl Pts',(-0.908249763301447,3.82863411803407,305.263107449907));
#7313=CARTESIAN_POINT('Ctrl Pts',(-0.789180877071169,3.85492918090016,305.256936649517));
#7314=CARTESIAN_POINT('Ctrl Pts',(-0.669314587155635,3.87562988215086,305.250765849127));
#7315=CARTESIAN_POINT('Ctrl Pts',(-0.54944829724011,3.89633058340156,305.244595048737));
#7316=CARTESIAN_POINT('Ctrl Pts',(-0.428785129427652,3.91143692830187,305.238424248348));
#7317=CARTESIAN_POINT('Ctrl Pts',(-0.307886798320349,3.92093033850642,305.232253447958));
#7318=CARTESIAN_POINT('Ctrl Pts',(-0.192654566553249,3.92997882441132,305.226371852289));
#7319=CARTESIAN_POINT('Ctrl Pts',(-0.0768375312944448,3.9339577482393,305.220490256619));
#7320=CARTESIAN_POINT('Ctrl Pts',(0.0390815966009194,3.93280582139611,305.21460866095));
#7321=CARTESIAN_POINT('Ctrl Pts',(0.154854253226902,3.93165535008653,305.208734497054));
#7322=CARTESIAN_POINT('Ctrl Pts',(0.270728337701162,3.92538692618264,305.202860333159));
#7323=CARTESIAN_POINT('Ctrl Pts',(0.386216376054573,3.9139910463448,305.196986169264));
#7324=CARTESIAN_POINT('Ctrl Pts',(0.501589083605886,3.90260654687138,305.191117871535));
#7325=CARTESIAN_POINT('Ctrl Pts',(0.616576104422988,3.88610481763749,305.185249573805));
#7326=CARTESIAN_POINT('Ctrl Pts',(0.730690976763123,3.86452839250496,305.179381276076));
#7327=CARTESIAN_POINT('Ctrl Pts',(0.846997547081014,3.84253756908796,305.173400271423));
#7328=CARTESIAN_POINT('Ctrl Pts',(0.962397687329678,3.81527511124227,305.16741926677));
#7329=CARTESIAN_POINT('Ctrl Pts',(1.07638252241415,3.78284148034799,305.161438262117));
#7330=CARTESIAN_POINT('Ctrl Pts',(1.1880964209889,3.75105402941691,305.155576417892));
#7331=CARTESIAN_POINT('Ctrl Pts',(1.29845047356426,3.71429966859478,305.149714573668));
#7332=CARTESIAN_POINT('Ctrl Pts',(1.40697761397419,3.67272419244564,305.143852729443));
#7333=CARTESIAN_POINT('Ctrl Pts',(1.51548976076468,3.63115446017646,305.137991695065));
#7334=CARTESIAN_POINT('Ctrl Pts',(1.62217511289051,3.5847650844574,305.132130660686));
#7335=CARTESIAN_POINT('Ctrl Pts',(1.72658463093574,3.53375077109528,305.126269626308));
#7336=CARTESIAN_POINT('Ctrl Pts',(1.8310047706039,3.48273126802622,305.120407995684));
#7337=CARTESIAN_POINT('Ctrl Pts',(1.9331482459501,3.42708607278105,305.11454636506));
#7338=CARTESIAN_POINT('Ctrl Pts',(2.03258938448524,3.36705648810321,305.108684734436));
#7339=CARTESIAN_POINT('Ctrl Pts',(2.13557616081782,3.30488650994704,305.1026141036));
#7340=CARTESIAN_POINT('Ctrl Pts',(2.23566388700295,3.23801389423704,305.096543472763));
#7341=CARTESIAN_POINT('Ctrl Pts',(2.33241234604614,3.16675569755728,305.090472841926));
#7342=CARTESIAN_POINT('Ctrl Pts',(2.4259676516519,3.0978493559657,305.084602570413));
#7343=CARTESIAN_POINT('Ctrl Pts',(2.51640034868806,3.02484266621994,305.078732298899));
#7344=CARTESIAN_POINT('Ctrl Pts',(2.60334693356386,2.94806271023933,305.072862027385));
#7345=CARTESIAN_POINT('Ctrl Pts',(2.69474490339167,2.86735186794321,305.066691216887));
#7346=CARTESIAN_POINT('Ctrl Pts',(2.78228997826085,2.78247154443906,305.060520406389));
#7347=CARTESIAN_POINT('Ctrl Pts',(2.86560565657207,2.69384357768267,305.054349595891));
#7348=CARTESIAN_POINT('Ctrl Pts',(2.94892133488328,2.60521561092629,305.048178785394));
#7349=CARTESIAN_POINT('Ctrl Pts',(3.02800733135905,2.51284044262219,305.042007974896));
#7350=CARTESIAN_POINT('Ctrl Pts',(3.10253867254258,2.4171766144363,305.035837164398));
#7351=CARTESIAN_POINT('Ctrl Pts',(3.17348408456588,2.32611546353521,305.029963250333));
#7352=CARTESIAN_POINT('Ctrl Pts',(3.24053631565406,2.23177517989596,305.024089336267));
#7353=CARTESIAN_POINT('Ctrl Pts',(3.30337740364183,2.13452259981209,305.018215422202));
#7354=CARTESIAN_POINT('Ctrl Pts',(3.36614122950051,2.03738959024549,305.012348730021));
#7355=CARTESIAN_POINT('Ctrl Pts',(3.42470398349916,1.93735174536747,305.006482037841));
#7356=CARTESIAN_POINT('Ctrl Pts',(3.47878801540304,1.83480869408452,305.000615345661));
#7357=CARTESIAN_POINT('Ctrl Pts',(3.53281858841152,1.73236700059722,304.994754452361));
#7358=CARTESIAN_POINT('Ctrl Pts',(3.58237905098065,1.62742538710442,304.988893559062));
#7359=CARTESIAN_POINT('Ctrl Pts',(3.62723552917024,1.52041159424843,304.983032665763));
#7360=CARTESIAN_POINT('Ctrl Pts',(3.67205847953301,1.41347778849932,304.97717615317));
#7361=CARTESIAN_POINT('Ctrl Pts',(3.71218428023923,1.3044752631427,304.971319640576));
#7362=CARTESIAN_POINT('Ctrl Pts',(3.74742573860542,1.19385482100531,304.965463127982));
#7363=CARTESIAN_POINT('Ctrl Pts',(3.78265198772662,1.08328211961088,304.959609142899));
#7364=CARTESIAN_POINT('Ctrl Pts',(3.81299796052456,0.971093282010455,304.953755157815));
#7365=CARTESIAN_POINT('Ctrl Pts',(3.83832542279738,0.857756928685132,304.947901172731));
#7366=CARTESIAN_POINT('Ctrl Pts',(3.86364640261167,0.744449583327597,304.94204868595));
#7367=CARTESIAN_POINT('Ctrl Pts',(3.88395134062945,0.629995709581894,304.93619619917));
#7368=CARTESIAN_POINT('Ctrl Pts',(3.89915268039494,0.514876077293334,304.930343712389));
#7369=CARTESIAN_POINT('Ctrl Pts',(3.91435720086164,0.399732357578294,304.924490001044));
#7370=CARTESIAN_POINT('Ctrl Pts',(3.92445593538042,0.283923010003483,304.9186362897));
#7371=CARTESIAN_POINT('Ctrl Pts',(3.92941301624533,0.167935546450875,304.912782578355));
#7372=CARTESIAN_POINT('Ctrl Pts',(3.93184596613777,0.111008557631404,304.909909559582));
#7373=CARTESIAN_POINT('Ctrl Pts',(3.93304114942374,0.054038722546335,304.907036540808));
#7374=CARTESIAN_POINT('Ctrl Pts',(3.93299891885253,-0.00291621412706657,
304.904163522035));
#7375=CARTESIAN_POINT('',(3.93299992201116,0.000783236989828259,303.654163521989));
#7376=CARTESIAN_POINT('Ctrl Pts',(3.932998918852,-0.00291621483949189,304.904163521999));
#7377=CARTESIAN_POINT('Ctrl Pts',(3.93289858185281,-0.138237283777497,304.897337424136));
#7378=CARTESIAN_POINT('Ctrl Pts',(3.92581040854498,-0.273276789480336,304.890511326274));
#7379=CARTESIAN_POINT('Ctrl Pts',(3.91184495515244,-0.40737948751549,304.883685228411));
#7380=CARTESIAN_POINT('Ctrl Pts',(3.8977947592586,-0.542295921971808,304.876817709723));
#7381=CARTESIAN_POINT('Ctrl Pts',(3.87678367602707,-0.676264042733198,304.869950191035));
#7382=CARTESIAN_POINT('Ctrl Pts',(3.84897348829923,-0.80863594179929,304.863082672347));
#7383=CARTESIAN_POINT('Ctrl Pts',(3.82098188003345,-0.941871372653556,304.856170353208));
#7384=CARTESIAN_POINT('Ctrl Pts',(3.78610224826225,-1.07348958982204,304.84925803407));
#7385=CARTESIAN_POINT('Ctrl Pts',(3.74454784416664,-1.20285096447855,304.842345714931));
#7386=CARTESIAN_POINT('Ctrl Pts',(3.73868682341047,-1.22109667677811,304.841370770234));
#7387=CARTESIAN_POINT('Ctrl Pts',(3.73269309461101,-1.2392975278324,304.840395825536));
#7388=CARTESIAN_POINT('Ctrl Pts',(3.72656733149945,-1.25745175804126,304.839420880838));
#7389=CARTESIAN_POINT('Ctrl Pts',(3.68961247830752,-1.36697067021004,304.833539337996));
#7390=CARTESIAN_POINT('Ctrl Pts',(3.64776609021771,-1.47503554230942,304.827657795155));
#7391=CARTESIAN_POINT('Ctrl Pts',(3.60116145689045,-1.58117840910084,304.821776252313));
#7392=CARTESIAN_POINT('Ctrl Pts',(3.55461572171183,-1.68718713432952,304.815902142466));
#7393=CARTESIAN_POINT('Ctrl Pts',(3.50332386513835,-1.79127831134769,304.810028032619));
#7394=CARTESIAN_POINT('Ctrl Pts',(3.44746866921305,-1.89299994051621,304.804153922772));
#7395=CARTESIAN_POINT('Ctrl Pts',(3.39166926383829,-1.99461996578561,304.798285680236));
#7396=CARTESIAN_POINT('Ctrl Pts',(3.33131578337192,-2.09387479244845,304.7924174377));
#7397=CARTESIAN_POINT('Ctrl Pts',(3.26663846483617,-2.19033379649149,304.786549195164));
#7398=CARTESIAN_POINT('Ctrl Pts',(3.20071810605026,-2.28864665637192,304.780568170252));
#7399=CARTESIAN_POINT('Ctrl Pts',(3.13030616592147,-2.38405471880515,304.77458714534));
#7400=CARTESIAN_POINT('Ctrl Pts',(3.05569496827276,-2.47612949194353,304.768606120428));
#7401=CARTESIAN_POINT('Ctrl Pts',(2.98257122751017,-2.5663686524707,304.762744333874));
#7402=CARTESIAN_POINT('Ctrl Pts',(2.90541438336051,-2.65340586451198,304.75688254732));
#7403=CARTESIAN_POINT('Ctrl Pts',(2.82454200990618,-2.7368689106852,304.751020760766));
#7404=CARTESIAN_POINT('Ctrl Pts',(2.74368082089702,-2.82032041412975,304.745159784883));
#7405=CARTESIAN_POINT('Ctrl Pts',(2.65910541096222,-2.90019843905125,304.739298808999));
#7406=CARTESIAN_POINT('Ctrl Pts',(2.57117124949181,-2.97616656217133,304.733437833115));
#7407=CARTESIAN_POINT('Ctrl Pts',(2.48322815377449,-3.0521424037703,304.727576261747));
#7408=CARTESIAN_POINT('Ctrl Pts',(2.39192593975536,-3.12420728464715,304.721714690379));
#7409=CARTESIAN_POINT('Ctrl Pts',(2.29765374571631,-3.19206457716567,304.715853119011));
#7410=CARTESIAN_POINT('Ctrl Pts',(2.20001795340542,-3.26234299368764,304.709782408867));
#7411=CARTESIAN_POINT('Ctrl Pts',(2.09919667238236,-3.32810768296923,304.703711698722));
#7412=CARTESIAN_POINT('Ctrl Pts',(1.99565444942337,-3.38907838777694,304.697640988578));
#7413=CARTESIAN_POINT('Ctrl Pts',(1.89553194798443,-3.44803539396618,304.691770777684));
#7414=CARTESIAN_POINT('Ctrl Pts',(1.7928657960717,-3.50250993923882,304.68590056679));
#7415=CARTESIAN_POINT('Ctrl Pts',(1.68809958710319,-3.55229626917886,304.680030355896));
#7416=CARTESIAN_POINT('Ctrl Pts',(1.57796588450083,-3.60463330522573,304.673859396126));
#7417=CARTESIAN_POINT('Ctrl Pts',(1.46551172948751,-3.65178881521169,304.667688436356));
#7418=CARTESIAN_POINT('Ctrl Pts',(1.35127301287926,-3.69358230511575,304.661517476586));
#7419=CARTESIAN_POINT('Ctrl Pts',(1.23703429627102,-3.73537579501982,304.655346516817));
#7420=CARTESIAN_POINT('Ctrl Pts',(1.12101153643795,-3.77180717603904,304.649175557047));
#7421=CARTESIAN_POINT('Ctrl Pts',(1.0037541319802,-3.80275776805895,304.643004597277));
#7422=CARTESIAN_POINT('Ctrl Pts',(0.891996200861796,-3.83225675063519,304.637123060839));
#7423=CARTESIAN_POINT('Ctrl Pts',(0.778756740574146,-3.85687246499804,304.631241524402));
#7424=CARTESIAN_POINT('Ctrl Pts',(0.664499721253345,-3.87645832177443,304.625359987964));
#7425=CARTESIAN_POINT('Ctrl Pts',(0.550387097470445,-3.89601942637068,304.619485884484));
#7426=CARTESIAN_POINT('Ctrl Pts',(0.435259874635114,-3.91056324675774,304.613611781005));
#7427=CARTESIAN_POINT('Ctrl Pts',(0.319595966757183,-3.91999329311066,304.607737677525));
#7428=CARTESIAN_POINT('Ctrl Pts',(0.204047588166283,-3.92941392039282,304.601869441312));
#7429=CARTESIAN_POINT('Ctrl Pts',(0.087963999044487,-3.93373090115052,304.596001205099));
#7430=CARTESIAN_POINT('Ctrl Pts',(-0.0281685801207231,-3.93289912546635,
304.590132968886));
#7431=CARTESIAN_POINT('Ctrl Pts',(-0.14653329841826,-3.93205136254529,304.584151941587));
#7432=CARTESIAN_POINT('Ctrl Pts',(-0.264948481105593,-3.92585479991437,
304.578170914289));
#7433=CARTESIAN_POINT('Ctrl Pts',(-0.382895478197291,-3.9143173163115,304.57218988699));
#7434=CARTESIAN_POINT('Ctrl Pts',(-0.498490903448139,-3.90300986163878,
304.566328106605));
#7435=CARTESIAN_POINT('Ctrl Pts',(-0.613636211076912,-3.8865725252648,304.56046632622));
#7436=CARTESIAN_POINT('Ctrl Pts',(-0.727845804985477,-3.86506526260101,
304.554604545835));
#7437=CARTESIAN_POINT('Ctrl Pts',(-0.84203960532356,-3.84356097408727,304.548743576051));
#7438=CARTESIAN_POINT('Ctrl Pts',(-0.955297544684902,-3.81698822974895,
304.542882606267));
#7439=CARTESIAN_POINT('Ctrl Pts',(-1.06714302021621,-3.78545833082387,304.537021636483));
#7440=CARTESIAN_POINT('Ctrl Pts',(-1.17899986089018,-3.75392522799806,304.531160071139));
#7441=CARTESIAN_POINT('Ctrl Pts',(-1.28944355605526,-3.71743408096652,304.525298505794));
#7442=CARTESIAN_POINT('Ctrl Pts',(-1.39801216409406,-3.67614621431807,304.51943694045));
#7443=CARTESIAN_POINT('Ctrl Pts',(-1.51045473897567,-3.63338510573259,304.513366221556));
#7444=CARTESIAN_POINT('Ctrl Pts',(-1.62088546638646,-3.58547873559274,304.507295502661));
#7445=CARTESIAN_POINT('Ctrl Pts',(-1.72881451684019,-3.53266038084085,304.501224783767));
#7446=CARTESIAN_POINT('Ctrl Pts',(-1.83317870755128,-3.48158659834023,304.495354578648));
#7447=CARTESIAN_POINT('Ctrl Pts',(-1.93520353332699,-3.42592044450438,304.489484373529));
#7448=CARTESIAN_POINT('Ctrl Pts',(-2.03447288800904,-3.3659187554004,304.48361416841));
#7449=CARTESIAN_POINT('Ctrl Pts',(-2.13882848909092,-3.3028427703451,304.477443192628));
#7450=CARTESIAN_POINT('Ctrl Pts',(-2.24013833713969,-3.2349754993727,304.471272216846));
#7451=CARTESIAN_POINT('Ctrl Pts',(-2.33795655125514,-3.16266472526621,304.465101241064));
#7452=CARTESIAN_POINT('Ctrl Pts',(-2.43577476537058,-3.09035395115972,304.458930265281));
#7453=CARTESIAN_POINT('Ctrl Pts',(-2.53010098584207,-3.01360005760262,304.452759289499));
#7454=CARTESIAN_POINT('Ctrl Pts',(-2.62053347657117,-2.93279615694132,304.446588313717));
#7455=CARTESIAN_POINT('Ctrl Pts',(-2.70672423362637,-2.85578236118208,304.440706787397));
#7456=CARTESIAN_POINT('Ctrl Pts',(-2.78965597749972,-2.77484175200591,304.434825261076));
#7457=CARTESIAN_POINT('Ctrl Pts',(-2.86895074997518,-2.69028076494198,304.428943734756));
#7458=CARTESIAN_POINT('Ctrl Pts',(-2.94814530867894,-2.60582664716071,304.423069641586));
#7459=CARTESIAN_POINT('Ctrl Pts',(-3.02371175836546,-2.51776154922697,304.417195548415));
#7460=CARTESIAN_POINT('Ctrl Pts',(-3.09530626831255,-2.42643114580757,304.411321455245));
#7461=CARTESIAN_POINT('Ctrl Pts',(-3.16682926478493,-2.33519196941801,304.405453229519));
#7462=CARTESIAN_POINT('Ctrl Pts',(-3.23438796115451,-2.24069429801477,304.399585003793));
#7463=CARTESIAN_POINT('Ctrl Pts',(-3.2976768286533,-2.14331904619053,304.393716778068));
#7464=CARTESIAN_POINT('Ctrl Pts',(-3.3621823038106,-2.04407194104044,304.387735746905));
#7465=CARTESIAN_POINT('Ctrl Pts',(-3.42225179757432,-1.94183579710125,304.381754715742));
#7466=CARTESIAN_POINT('Ctrl Pts',(-3.47760613315286,-1.83704778997651,304.375773684579));
#7467=CARTESIAN_POINT('Ctrl Pts',(-3.53185670443235,-1.73434925353234,304.369911915053));
#7468=CARTESIAN_POINT('Ctrl Pts',(-3.58157821540421,-1.62920005989815,304.364050145527));
#7469=CARTESIAN_POINT('Ctrl Pts',(-3.62655316235846,-1.52203848853696,304.358188376));
#7470=CARTESIAN_POINT('Ctrl Pts',(-3.67152188898382,-1.41489173832094,304.352327417195));
#7471=CARTESIAN_POINT('Ctrl Pts',(-3.71174519781089,-1.30573354350387,304.34646645839));
#7472=CARTESIAN_POINT('Ctrl Pts',(-3.74705338999338,-1.19502296736888,304.340605499585));
#7473=CARTESIAN_POINT('Ctrl Pts',(-3.78236516936451,-1.0843011434272,304.334743945327));
#7474=CARTESIAN_POINT('Ctrl Pts',(-3.81276071427995,-0.972027016978667,
304.328882391069));
#7475=CARTESIAN_POINT('Ctrl Pts',(-3.83812014989347,-0.858674976333749,
304.323020836812));
#7476=CARTESIAN_POINT('Ctrl Pts',(-3.86438458051746,-0.741277773455159,
304.316950102924));
#7477=CARTESIAN_POINT('Ctrl Pts',(-3.88524663614198,-0.622724749329648,
304.310879369036));
#7478=CARTESIAN_POINT('Ctrl Pts',(-3.90063112327204,-0.503553214825912,
304.304808635148));
#7479=CARTESIAN_POINT('Ctrl Pts',(-3.91550740077476,-0.388318381014748,
304.298938441283));
#7480=CARTESIAN_POINT('Ctrl Pts',(-3.92526231205771,-0.272505677092596,
304.293068247419));
#7481=CARTESIAN_POINT('Ctrl Pts',(-3.92988094354268,-0.156603861957868,
304.287198053554));
#7482=CARTESIAN_POINT('Ctrl Pts',(-3.93473625046463,-0.0347628172409708,
304.281027049654));
#7483=CARTESIAN_POINT('Ctrl Pts',(-3.93391493363068,0.087176183760976,304.274856045755));
#7484=CARTESIAN_POINT('Ctrl Pts',(-3.92746157474384,0.208649416271988,304.268685041856));
#7485=CARTESIAN_POINT('Ctrl Pts',(-3.921008215857,0.33012264878301,304.262514037956));
#7486=CARTESIAN_POINT('Ctrl Pts',(-3.90892293693869,0.451129601202003,304.256343034056));
#7487=CARTESIAN_POINT('Ctrl Pts',(-3.89131247210783,0.571118415407881,304.250172030157));
#7488=CARTESIAN_POINT('Ctrl Pts',(-3.87452808317339,0.685478765617703,304.244290497184));
#7489=CARTESIAN_POINT('Ctrl Pts',(-3.8526710536493,0.799282807439263,304.238408964212));
#7490=CARTESIAN_POINT('Ctrl Pts',(-3.82578888167082,0.912046288783581,304.232527431239));
#7491=CARTESIAN_POINT('Ctrl Pts',(-3.79894068327732,1.02466726007633,304.226653331325));
#7492=CARTESIAN_POINT('Ctrl Pts',(-3.76708006778264,1.13624988921146,304.220779231411));
#7493=CARTESIAN_POINT('Ctrl Pts',(-3.73030608239908,1.24631678622106,304.214905131497));
#7494=CARTESIAN_POINT('Ctrl Pts',(-3.69356882882083,1.35627374258135,304.209036898946));
#7495=CARTESIAN_POINT('Ctrl Pts',(-3.65192809787854,1.46471759014417,304.203168666394));
#7496=CARTESIAN_POINT('Ctrl Pts',(-3.60553344826318,1.57118348815644,304.197300433842));
#7497=CARTESIAN_POINT('Ctrl Pts',(-3.55824702506397,1.67969581773388,304.191319405207));
#7498=CARTESIAN_POINT('Ctrl Pts',(-3.50602214065162,1.78615295097963,304.185338376572));
#7499=CARTESIAN_POINT('Ctrl Pts',(-3.44906982329833,1.89008104429752,304.179357347937));
#7500=CARTESIAN_POINT('Ctrl Pts',(-3.39325304387148,1.99193697800772,304.173495571426));
#7501=CARTESIAN_POINT('Ctrl Pts',(-3.33289580730175,2.09136341065753,304.167633794916));
#7502=CARTESIAN_POINT('Ctrl Pts',(-3.26824404264322,2.18793735690195,304.161772018405));
#7503=CARTESIAN_POINT('Ctrl Pts',(-3.2036012192196,2.28449794712517,304.155911052569));
#7504=CARTESIAN_POINT('Ctrl Pts',(-3.13466527787735,2.378206493361,304.150050086733));
#7505=CARTESIAN_POINT('Ctrl Pts',(-3.06172583056679,2.46866845453983,304.144189120897));
#7506=CARTESIAN_POINT('Ctrl Pts',(-2.98877897238865,2.55913960692645,304.138327559569));
#7507=CARTESIAN_POINT('Ctrl Pts',(-2.91182805810292,2.64636319793497,304.132465998241));
#7508=CARTESIAN_POINT('Ctrl Pts',(-2.83120293942275,2.72997782331725,304.126604436913));
#7509=CARTESIAN_POINT('Ctrl Pts',(-2.74770080899298,2.81657613745064,304.12053371272));
#7510=CARTESIAN_POINT('Ctrl Pts',(-2.66025768582945,2.8993027666353,304.114462988527));
#7511=CARTESIAN_POINT('Ctrl Pts',(-2.56928054670307,2.97779893081,304.108392264334));
#7512=CARTESIAN_POINT('Ctrl Pts',(-2.48130849047592,3.05370227350359,304.102522063367));
#7513=CARTESIAN_POINT('Ctrl Pts',(-2.39003256385641,3.12565000216864,304.0966518624));
#7514=CARTESIAN_POINT('Ctrl Pts',(-2.29585243950112,3.19336038931354,304.090781661434));
#7515=CARTESIAN_POINT('Ctrl Pts',(-2.19684659388923,3.26454020758072,304.084610675627));
#7516=CARTESIAN_POINT('Ctrl Pts',(-2.09463149333541,3.33103665703813,304.078439689821));
#7517=CARTESIAN_POINT('Ctrl Pts',(-1.9897021452276,3.39257636218799,304.072268704015));
#7518=CARTESIAN_POINT('Ctrl Pts',(-1.8847727971198,3.45411606733785,304.066097718209));
#7519=CARTESIAN_POINT('Ctrl Pts',(-1.77712969562501,3.51069884814968,304.059926732403));
#7520=CARTESIAN_POINT('Ctrl Pts',(-1.66729218737832,3.56210973468073,304.053755746597));
#7521=CARTESIAN_POINT('Ctrl Pts',(-1.56260667784775,3.61110916063123,304.047874214835));
#7522=CARTESIAN_POINT('Ctrl Pts',(-1.45559066607334,3.65556877396117,304.041992683073));
#7523=CARTESIAN_POINT('Ctrl Pts',(-1.34667444822617,3.69526141571807,304.03611115131));
#7524=CARTESIAN_POINT('Ctrl Pts',(-1.2378958783929,3.73490389402446,304.030237052612));
#7525=CARTESIAN_POINT('Ctrl Pts',(-1.12722226223042,3.76979124274884,304.024362953913));
#7526=CARTESIAN_POINT('Ctrl Pts',(-1.01510657010295,3.79974310333394,304.018488855215));
#7527=CARTESIAN_POINT('Ctrl Pts',(-0.903102865156112,3.82966504639047,304.012620623882));
#7528=CARTESIAN_POINT('Ctrl Pts',(-0.789660345248424,3.85466120232958,304.006752392549));
#7529=CARTESIAN_POINT('Ctrl Pts',(-0.675249337169474,3.87460028037115,304.000884161216));
#7530=CARTESIAN_POINT('Ctrl Pts',(-0.558639147693519,3.89492262266533,303.994903132125));
#7531=CARTESIAN_POINT('Ctrl Pts',(-0.441023261496849,3.90999131716952,303.988922103034));
#7532=CARTESIAN_POINT('Ctrl Pts',(-0.322913385607228,3.91972141170717,303.982941073943));
#7533=CARTESIAN_POINT('Ctrl Pts',(-0.207158464222991,3.92925750104588,303.977079298651));
#7534=CARTESIAN_POINT('Ctrl Pts',(-0.0909294983870328,3.93366587280026,
303.97121752336));
#7535=CARTESIAN_POINT('Ctrl Pts',(0.0252850199611637,3.93291872122544,303.965355748068));
#7536=CARTESIAN_POINT('Ctrl Pts',(0.141483466069428,3.93217167298022,303.959494783448));
#7537=CARTESIAN_POINT('Ctrl Pts',(0.257667056973605,3.92627052199346,303.953633818828));
#7538=CARTESIAN_POINT('Ctrl Pts',(0.373346971566622,3.91523958894242,303.947772854208));
#7539=CARTESIAN_POINT('Ctrl Pts',(0.489038639661692,3.90420753510828,303.941911294093));
#7540=CARTESIAN_POINT('Ctrl Pts',(0.604226119765026,3.88804470218821,303.936049733978));
#7541=CARTESIAN_POINT('Ctrl Pts',(0.718426074707708,3.86682724920316,303.930188173863));
#7542=CARTESIAN_POINT('Ctrl Pts',(0.836701177391101,3.84485266583536,303.924117447961));
#7543=CARTESIAN_POINT('Ctrl Pts',(0.953916490991689,3.81745606708269,303.918046722058));
#7544=CARTESIAN_POINT('Ctrl Pts',(1.06954837564919,3.78477942186149,303.911975996156));
#7545=CARTESIAN_POINT('Ctrl Pts',(1.18136074770322,3.75318214033509,303.906105796382));
#7546=CARTESIAN_POINT('Ctrl Pts',(1.2916922678671,3.71664831157857,303.900235596608));
#7547=CARTESIAN_POINT('Ctrl Pts',(1.40008762461898,3.67535626074382,303.894365396833));
#7548=CARTESIAN_POINT('Ctrl Pts',(1.51403716232148,3.63194840413075,303.888194407867));
#7549=CARTESIAN_POINT('Ctrl Pts',(1.62584637718348,3.58328199783037,303.882023418901));
#7550=CARTESIAN_POINT('Ctrl Pts',(1.73501440219909,3.52961952966063,303.875852429935));
#7551=CARTESIAN_POINT('Ctrl Pts',(1.8441824272147,3.47595706149089,303.869681440968));
#7552=CARTESIAN_POINT('Ctrl Pts',(1.95070883987929,3.41729884466744,303.863510452002));
#7553=CARTESIAN_POINT('Ctrl Pts',(2.0541281053617,3.3539598576553,303.857339463036));
#7554=CARTESIAN_POINT('Ctrl Pts',(2.15269635933167,3.29359186597704,303.851457932116));
#7555=CARTESIAN_POINT('Ctrl Pts',(2.24875994985064,3.22877777680599,303.845576401196));
#7556=CARTESIAN_POINT('Ctrl Pts',(2.3418922328573,3.15975153606777,303.839694870276));
#7557=CARTESIAN_POINT('Ctrl Pts',(2.43490681524703,3.09081253072051,303.833820772437));
#7558=CARTESIAN_POINT('Ctrl Pts',(2.52499712999191,3.01767220416633,303.827946674598));
#7559=CARTESIAN_POINT('Ctrl Pts',(2.61176309746407,2.94060920945387,303.822072576759));
#7560=CARTESIAN_POINT('Ctrl Pts',(2.69844239816774,2.86362318963049,303.816204346302));
#7561=CARTESIAN_POINT('Ctrl Pts',(2.78180365085279,2.78272256786997,303.810336115845));
#7562=CARTESIAN_POINT('Ctrl Pts',(2.86147816236328,2.69822751566988,303.804467885388));
#7563=CARTESIAN_POINT('Ctrl Pts',(2.94268417502951,2.61210830202036,303.798486855975));
#7564=CARTESIAN_POINT('Ctrl Pts',(3.02005989973372,2.52225530454719,303.792505826562));
#7565=CARTESIAN_POINT('Ctrl Pts',(3.09325251609353,2.42904875860511,303.786524797149));
#7566=CARTESIAN_POINT('Ctrl Pts',(3.16498575360255,2.3377006468695,303.780663022768));
#7567=CARTESIAN_POINT('Ctrl Pts',(3.23270088527501,2.24313181847449,303.774801248388));
#7568=CARTESIAN_POINT('Ctrl Pts',(3.2961055721996,2.14573461940539,303.768939474007));
#7569=CARTESIAN_POINT('Ctrl Pts',(3.35950149025488,2.0483508903706,303.76307851031));
#7570=CARTESIAN_POINT('Ctrl Pts',(3.41858792448416,1.94813991359881,303.757217546613));
#7571=CARTESIAN_POINT('Ctrl Pts',(3.47311585615841,1.84552302876476,303.751356582916));
#7572=CARTESIAN_POINT('Ctrl Pts',(3.52764932797323,1.7428957178619,303.745495023734));
#7573=CARTESIAN_POINT('Ctrl Pts',(3.57762318328595,1.63786237661532,303.739633464551));
#7574=CARTESIAN_POINT('Ctrl Pts',(3.62283468586133,1.53086832840712,303.733771905369));
#7575=CARTESIAN_POINT('Ctrl Pts',(3.66965954730188,1.42005622978335,303.727701178212));
#7576=CARTESIAN_POINT('Ctrl Pts',(3.71137563286428,1.30714131382758,303.721630451054));
#7577=CARTESIAN_POINT('Ctrl Pts',(3.74781292236082,1.19263879652864,303.715559723896));
#7578=CARTESIAN_POINT('Ctrl Pts',(3.78304661486231,1.08191852779017,303.709689525072));
#7579=CARTESIAN_POINT('Ctrl Pts',(3.81334469335758,0.969714304700055,303.703819326249));
#7580=CARTESIAN_POINT('Ctrl Pts',(3.83860512395872,0.856504350437184,303.697949127425));
#7581=CARTESIAN_POINT('Ctrl Pts',(3.86515991414326,0.737493450357144,303.6917781361));
#7582=CARTESIAN_POINT('Ctrl Pts',(3.88614702616928,0.617371542182774,303.685607144776));
#7583=CARTESIAN_POINT('Ctrl Pts',(3.90150956439052,0.496701237132804,303.679436153451));
#7584=CARTESIAN_POINT('Ctrl Pts',(3.91687210261177,0.376030932082834,303.673265162126));
#7585=CARTESIAN_POINT('Ctrl Pts',(3.92661009564078,0.254812755321279,303.667094170801));
#7586=CARTESIAN_POINT('Ctrl Pts',(3.93072991968281,0.13360875162347,303.660923179476));
#7587=CARTESIAN_POINT('Ctrl Pts',(3.93223419442983,0.0893534338866097,303.658669960329));
#7588=CARTESIAN_POINT('Ctrl Pts',(3.93299110200493,0.0450725701889574,303.656416741182));
#7589=CARTESIAN_POINT('Ctrl Pts',(3.93299992201098,0.000783237888672866,
303.654163522035));
#7590=CARTESIAN_POINT('',(3.93299951520447,0.0019527932382245,302.404163522072));
#7591=CARTESIAN_POINT('Ctrl Pts',(3.93299992201116,0.00078323698981516,
303.654163521989));
#7592=CARTESIAN_POINT('Ctrl Pts',(3.93302281745676,-0.114185523302119,303.648314487955));
#7593=CARTESIAN_POINT('Ctrl Pts',(3.92800032631236,-0.229348643469013,303.64246545392));
#7594=CARTESIAN_POINT('Ctrl Pts',(3.91790739951338,-0.344224648795359,303.636616419885));
#7595=CARTESIAN_POINT('Ctrl Pts',(3.90782710347176,-0.458956892953262,303.630774705603));
#7596=CARTESIAN_POINT('Ctrl Pts',(3.8926890250553,-0.573402325072434,303.624932991321));
#7597=CARTESIAN_POINT('Ctrl Pts',(3.87252011576164,-0.687078563936791,303.619091277039));
#7598=CARTESIAN_POINT('Ctrl Pts',(3.85237094282903,-0.800643564495698,303.613255279188));
#7599=CARTESIAN_POINT('Ctrl Pts',(3.82720080237384,-0.913440460580957,303.607419281338));
#7600=CARTESIAN_POINT('Ctrl Pts',(3.79708846201241,-1.02499181052936,303.601583283487));
#7601=CARTESIAN_POINT('Ctrl Pts',(3.76699639105037,-1.13646807236309,303.595751213998));
#7602=CARTESIAN_POINT('Ctrl Pts',(3.73196884489983,-1.2467000542881,303.589919144509));
#7603=CARTESIAN_POINT('Ctrl Pts',(3.69213556805134,-1.35522099567937,303.58408707502));
#7604=CARTESIAN_POINT('Ctrl Pts',(3.65231622209874,-1.46370398403098,303.578257045182));
#7605=CARTESIAN_POINT('Ctrl Pts',(3.6076946297648,-1.57047673042795,303.572427015343));
#7606=CARTESIAN_POINT('Ctrl Pts',(3.55845004246602,-1.67508874250696,303.566596985505));
#7607=CARTESIAN_POINT('Ctrl Pts',(3.50921051334932,-1.77969000931156,303.5607675545));
#7608=CARTESIAN_POINT('Ctrl Pts',(3.45534911114047,-1.88213060601439,303.554938123496));
#7609=CARTESIAN_POINT('Ctrl Pts',(3.39709245674577,-1.98198179616287,303.549108692492));
#7610=CARTESIAN_POINT('Ctrl Pts',(3.33882739578794,-2.08184739505731,303.543278420288));
#7611=CARTESIAN_POINT('Ctrl Pts',(3.2761660323174,-2.17912248475528,303.537448148084));
#7612=CARTESIAN_POINT('Ctrl Pts',(3.20937959701542,-2.27340528772613,303.53161787588));
#7613=CARTESIAN_POINT('Ctrl Pts',(3.14252613685886,-2.36778271007785,303.525781752591));
#7614=CARTESIAN_POINT('Ctrl Pts',(3.07153957837072,-2.45916150746637,303.519945629302));
#7615=CARTESIAN_POINT('Ctrl Pts',(2.99673300382066,-2.54717103937133,303.514109506012));
#7616=CARTESIAN_POINT('Ctrl Pts',(2.92188788897986,-2.63522591372069,303.508270375956));
#7617=CARTESIAN_POINT('Ctrl Pts',(2.84321912185116,-2.71990775983271,303.502431245901));
#7618=CARTESIAN_POINT('Ctrl Pts',(2.76107712497651,-2.8008823805957,303.496592115845));
#7619=CARTESIAN_POINT('Ctrl Pts',(2.67880484893882,-2.88198542903542,303.49074372479));
#7620=CARTESIAN_POINT('Ctrl Pts',(2.59304864821594,-2.95936922681172,303.484895333735));
#7621=CARTESIAN_POINT('Ctrl Pts',(2.50419283663215,-3.03273922996361,303.47904694268));
#7622=CARTESIAN_POINT('Ctrl Pts',(2.43055619346647,-3.09354246438193,303.474200260425));
#7623=CARTESIAN_POINT('Ctrl Pts',(2.35479148636737,-3.15158980484418,303.469353578171));
#7624=CARTESIAN_POINT('Ctrl Pts',(2.27713161213407,-3.20673675580327,303.464506895916));
#7625=CARTESIAN_POINT('Ctrl Pts',(2.18289003236076,-3.2736585198336,303.458625364471));
#7626=CARTESIAN_POINT('Ctrl Pts',(2.08554403724773,-3.33653013104214,303.452743833026));
#7627=CARTESIAN_POINT('Ctrl Pts',(1.98547639138384,-3.39505117770814,303.446862301581));
#7628=CARTESIAN_POINT('Ctrl Pts',(1.88553521088994,-3.45349826554603,303.440988203208));
#7629=CARTESIAN_POINT('Ctrl Pts',(1.7828795729352,-3.50760551789798,303.435114104835));
#7630=CARTESIAN_POINT('Ctrl Pts',(1.67792291624083,-3.5571145170143,303.429240006462));
#7631=CARTESIAN_POINT('Ctrl Pts',(1.57307109605297,-3.60657406380742,303.423371775464));
#7632=CARTESIAN_POINT('Ctrl Pts',(1.4659231995758,-3.65144431930907,303.417503544465));
#7633=CARTESIAN_POINT('Ctrl Pts',(1.35691851279986,-3.6915120411047,303.411635313466));
#7634=CARTESIAN_POINT('Ctrl Pts',(1.24581855506428,-3.73234993835224,303.405654284253));
#7635=CARTESIAN_POINT('Ctrl Pts',(1.13279006261976,-3.76819854734679,303.39967325504));
#7636=CARTESIAN_POINT('Ctrl Pts',(1.0183213179728,-3.7988828217467,303.393692225827));
#7637=CARTESIAN_POINT('Ctrl Pts',(0.906134937536904,-3.82895528992868,303.387830450888));
#7638=CARTESIAN_POINT('Ctrl Pts',(0.792565622138403,-3.85406734576113,303.381968675949));
#7639=CARTESIAN_POINT('Ctrl Pts',(0.678089027243571,-3.87410431856602,303.37610690101));
#7640=CARTESIAN_POINT('Ctrl Pts',(0.563628264361583,-3.89413852027511,303.370245936749));
#7641=CARTESIAN_POINT('Ctrl Pts',(0.448260877050694,-3.90909896380373,303.364384972489));
#7642=CARTESIAN_POINT('Ctrl Pts',(0.332472161685852,-3.918922206641,303.358524008228));
#7643=CARTESIAN_POINT('Ctrl Pts',(0.21667168188089,-3.92874644754575,303.352662448478));
#7644=CARTESIAN_POINT('Ctrl Pts',(0.100450199256683,-3.93343241534604,303.346800888727));
#7645=CARTESIAN_POINT('Ctrl Pts',(-0.0157031198889865,-3.93296865128947,
303.340939328977));
#7646=CARTESIAN_POINT('Ctrl Pts',(-0.136001308306843,-3.93248833805979,
303.334868602592));
#7647=CARTESIAN_POINT('Ctrl Pts',(-0.256225900974122,-3.92648389608309,
303.328797876207));
#7648=CARTESIAN_POINT('Ctrl Pts',(-0.375836314876531,-3.91500141308021,
303.322727149822));
#7649=CARTESIAN_POINT('Ctrl Pts',(-0.491495782150235,-3.90389821709783,
303.316856950424));
#7650=CARTESIAN_POINT('Ctrl Pts',(-0.606580599238758,-3.88767328386376,
303.310986751026));
#7651=CARTESIAN_POINT('Ctrl Pts',(-0.720610913079052,-3.8664206848132,303.305116551628));
#7652=CARTESIAN_POINT('Ctrl Pts',(-0.840484168634247,-3.8440790972879,303.29894556175));
#7653=CARTESIAN_POINT('Ctrl Pts',(-0.959191476892085,-3.81618107976753,
303.292774571871));
#7654=CARTESIAN_POINT('Ctrl Pts',(-1.07619311940163,-3.78289536859699,303.286603581992));
#7655=CARTESIAN_POINT('Ctrl Pts',(-1.19319476191117,-3.74960965742646,303.280432592113));
#7656=CARTESIAN_POINT('Ctrl Pts',(-1.3084902669871,-3.71093648525967,303.274261602235));
#7657=CARTESIAN_POINT('Ctrl Pts',(-1.42156529726405,-3.66710254909984,303.268090612356));
#7658=CARTESIAN_POINT('Ctrl Pts',(-1.5293363926921,-3.62532470207829,303.262209080974));
#7659=CARTESIAN_POINT('Ctrl Pts',(-1.63543784988199,-3.57872467305038,303.256327549592));
#7660=CARTESIAN_POINT('Ctrl Pts',(-1.73940807988741,-3.5274563826676,303.25044601821));
#7661=CARTESIAN_POINT('Ctrl Pts',(-1.84324691241313,-3.47625288510239,303.244571919901));
#7662=CARTESIAN_POINT('Ctrl Pts',(-1.94495950844133,-3.42039304042524,303.238697821593));
#7663=CARTESIAN_POINT('Ctrl Pts',(-2.04410242477204,-3.36007950457144,303.232823723285));
#7664=CARTESIAN_POINT('Ctrl Pts',(-2.14314631165635,-3.29982621322413,303.226955492352));
#7665=CARTESIAN_POINT('Ctrl Pts',(-2.23962527490243,-3.23512829294086,303.221087261419));
#7666=CARTESIAN_POINT('Ctrl Pts',(-2.3331193313831,-3.16623485950213,303.215219030486));
#7667=CARTESIAN_POINT('Ctrl Pts',(-2.42841051738148,-3.0960171662391,303.209238001249));
#7668=CARTESIAN_POINT('Ctrl Pts',(-2.52060047000611,-3.02144119402228,303.203256972012));
#7669=CARTESIAN_POINT('Ctrl Pts',(-2.60927408767226,-2.94281799223161,303.197275942775));
#7670=CARTESIAN_POINT('Ctrl Pts',(-2.69617966245841,-2.865762440389,303.191414167905));
#7671=CARTESIAN_POINT('Ctrl Pts',(-2.77970750465655,-2.78481984324435,303.185552393035));
#7672=CARTESIAN_POINT('Ctrl Pts',(-2.85949985540938,-2.70032397628762,303.179690618165));
#7673=CARTESIAN_POINT('Ctrl Pts',(-2.9392811709355,-2.61583979505061,303.173829653975));
#7674=CARTESIAN_POINT('Ctrl Pts',(-3.01532773974606,-2.52780362060482,303.167968689784));
#7675=CARTESIAN_POINT('Ctrl Pts',(-3.08731924325342,-2.43658549824075,303.162107725594));
#7676=CARTESIAN_POINT('Ctrl Pts',(-3.15931806127636,-2.34535810788888,303.156246165914));
#7677=CARTESIAN_POINT('Ctrl Pts',(-3.22726073983907,-2.25094845019649,303.150384606235));
#7678=CARTESIAN_POINT('Ctrl Pts',(-3.29086821071063,-2.1537584404325,303.144523046556));
#7679=CARTESIAN_POINT('Ctrl Pts',(-3.35674548210072,-2.05310025418646,303.138452320076));
#7680=CARTESIAN_POINT('Ctrl Pts',(-3.41797210375618,-1.94945997573294,303.132381593596));
#7681=CARTESIAN_POINT('Ctrl Pts',(-3.47428870424946,-1.84331413479217,303.126310867116));
#7682=CARTESIAN_POINT('Ctrl Pts',(-3.52874506483207,-1.74067448435188,303.120440667791));
#7683=CARTESIAN_POINT('Ctrl Pts',(-3.57861053220966,-1.63569258845348,303.114570468466));
#7684=CARTESIAN_POINT('Ctrl Pts',(-3.62369923834598,-1.52882073180958,303.108700269142));
#7685=CARTESIAN_POINT('Ctrl Pts',(-3.67109830299077,-1.4164727299295,303.102529279084));
#7686=CARTESIAN_POINT('Ctrl Pts',(-3.713217931585,-1.30203644971664,303.096358289026));
#7687=CARTESIAN_POINT('Ctrl Pts',(-3.74990158412267,-1.18605527248703,303.090187298969));
#7688=CARTESIAN_POINT('Ctrl Pts',(-3.78658523666034,-1.07007409525744,303.084016308911));
#7689=CARTESIAN_POINT('Ctrl Pts',(-3.81783284742591,-0.952548542831441,
303.077845318853));
#7690=CARTESIAN_POINT('Ctrl Pts',(-3.84355023053837,-0.834032748354919,
303.071674328796));
#7691=CARTESIAN_POINT('Ctrl Pts',(-3.86806130514394,-0.721076096908286,
303.065792797342));
#7692=CARTESIAN_POINT('Ctrl Pts',(-3.88762819483243,-0.606856050001968,
303.059911265888));
#7693=CARTESIAN_POINT('Ctrl Pts',(-3.90212504068358,-0.491842624088376,
303.054029734433));
#7694=CARTESIAN_POINT('Ctrl Pts',(-3.91660356543746,-0.376974552011518,
303.048155636052));
#7695=CARTESIAN_POINT('Ctrl Pts',(-3.92602473886699,-0.261315500137586,
303.042281537671));
#7696=CARTESIAN_POINT('Ctrl Pts',(-3.93031337093058,-0.14534719221326,303.036407439289));
#7697=CARTESIAN_POINT('Ctrl Pts',(-3.93459771927125,-0.029494719849412,
303.030539208283));
#7698=CARTESIAN_POINT('Ctrl Pts',(-3.93375970938358,0.0866659848548804,
303.024670977276));
#7699=CARTESIAN_POINT('Ctrl Pts',(-3.927775849082,0.202647179521869,303.018802746269));
#7700=CARTESIAN_POINT('Ctrl Pts',(-3.92167696796974,0.320857746260009,303.012821717059));
#7701=CARTESIAN_POINT('Ctrl Pts',(-3.91023231220583,0.438881399424562,303.006840687849));
#7702=CARTESIAN_POINT('Ctrl Pts',(-3.89347276509992,0.556200348278578,303.000859658639));
#7703=CARTESIAN_POINT('Ctrl Pts',(-3.87704738246301,0.671180103597108,302.994997883693));
#7704=CARTESIAN_POINT('Ctrl Pts',(-3.8555171511324,0.785482570408821,302.989136108747));
#7705=CARTESIAN_POINT('Ctrl Pts',(-3.82896351313979,0.898625291789752,302.983274333801));
#7706=CARTESIAN_POINT('Ctrl Pts',(-3.80241354749404,1.01175236562296,302.977413369534));
#7707=CARTESIAN_POINT('Ctrl Pts',(-3.77084165086854,1.12371961218863,302.971552405267));
#7708=CARTESIAN_POINT('Ctrl Pts',(-3.73438016152757,1.23405583714405,302.965691440999));
#7709=CARTESIAN_POINT('Ctrl Pts',(-3.69791496760562,1.34440327254336,302.959829881243));
#7710=CARTESIAN_POINT('Ctrl Pts',(-3.65655932259171,1.45311896589117,302.953968321487));
#7711=CARTESIAN_POINT('Ctrl Pts',(-3.61049488832033,1.55974858916838,302.948106761731));
#7712=CARTESIAN_POINT('Ctrl Pts',(-3.56278666940059,1.6701832334032,302.942036035356));
#7713=CARTESIAN_POINT('Ctrl Pts',(-3.51002750913876,1.77837970737051,302.935965308981));
#7714=CARTESIAN_POINT('Ctrl Pts',(-3.45247218995707,1.88385901212724,302.929894582607));
#7715=CARTESIAN_POINT('Ctrl Pts',(-3.39681802611691,1.98585414641094,302.924024383204));
#7716=CARTESIAN_POINT('Ctrl Pts',(-3.33667982061495,2.08530845684434,302.918154183801));
#7717=CARTESIAN_POINT('Ctrl Pts',(-3.27233261907056,2.18181764365558,302.912283984399));
#7718=CARTESIAN_POINT('Ctrl Pts',(-3.20468825112871,2.28327198488167,302.906112994538));
#7719=CARTESIAN_POINT('Ctrl Pts',(-3.13239243580357,2.3814709637078,302.899942004677));
#7720=CARTESIAN_POINT('Ctrl Pts',(-3.05581240058875,2.47598456627016,302.893771014817));
#7721=CARTESIAN_POINT('Ctrl Pts',(-2.97923236537393,2.5704981688325,302.887600024956));
#7722=CARTESIAN_POINT('Ctrl Pts',(-2.89836850954299,2.6613260527928,302.881429035095));
#7723=CARTESIAN_POINT('Ctrl Pts',(-2.8136313873192,2.74808431753689,302.875258045235));
#7724=CARTESIAN_POINT('Ctrl Pts',(-2.73286897173148,2.83077307128554,302.869376513804));
#7725=CARTESIAN_POINT('Ctrl Pts',(-2.64832821169403,2.9100317746915,302.863494982373));
#7726=CARTESIAN_POINT('Ctrl Pts',(-2.56033201258136,2.98549643867667,302.857613450943));
#7727=CARTESIAN_POINT('Ctrl Pts',(-2.47244702296915,3.06086573050181,302.851739352585));
#7728=CARTESIAN_POINT('Ctrl Pts',(-2.38111558943836,3.13245025346504,302.845865254227));
#7729=CARTESIAN_POINT('Ctrl Pts',(-2.28669830350421,3.19992185353814,302.83999115587));
#7730=CARTESIAN_POINT('Ctrl Pts',(-2.19237532678118,3.26732605924258,302.834122924886));
#7731=CARTESIAN_POINT('Ctrl Pts',(-2.09497296236576,3.3306252762734,302.828254693903));
#7732=CARTESIAN_POINT('Ctrl Pts',(-1.99488530741481,3.38953117853495,302.82238646292));
#7733=CARTESIAN_POINT('Ctrl Pts',(-1.89287378292001,3.44956936100997,302.816405433702));
#7734=CARTESIAN_POINT('Ctrl Pts',(-1.78807299843604,3.50504330508081,302.810424404483));
#7735=CARTESIAN_POINT('Ctrl Pts',(-1.68093208576082,3.55569350803184,302.804443375264));
#7736=CARTESIAN_POINT('Ctrl Pts',(-1.57592742985989,3.60533380882251,302.798581600343));
#7737=CARTESIAN_POINT('Ctrl Pts',(-1.46867548891796,3.65034076207152,302.792719825421));
#7738=CARTESIAN_POINT('Ctrl Pts',(-1.35962376252657,3.69051652541661,302.786858050499));
#7739=CARTESIAN_POINT('Ctrl Pts',(-1.25058711790335,3.73068673248516,302.780997086256));
#7740=CARTESIAN_POINT('Ctrl Pts',(-1.13975156915167,3.76602693607683,302.775136122013));
#7741=CARTESIAN_POINT('Ctrl Pts',(-1.02758325800181,3.79638797383439,302.76927515777));
#7742=CARTESIAN_POINT('Ctrl Pts',(-0.915403550264176,3.82675209635117,302.763413598038));
#7743=CARTESIAN_POINT('Ctrl Pts',(-0.801891208443604,3.85213593975903,302.757552038306));
#7744=CARTESIAN_POINT('Ctrl Pts',(-0.687525473410276,3.87244079663098,302.751690478574));
#7745=CARTESIAN_POINT('Ctrl Pts',(-0.569078657271046,3.8934702216414,302.745619752166));
#7746=CARTESIAN_POINT('Ctrl Pts',(-0.449716873294232,3.90905132129786,302.739549025757));
#7747=CARTESIAN_POINT('Ctrl Pts',(-0.329980236899369,3.91913281776158,302.733478299349));
#7748=CARTESIAN_POINT('Ctrl Pts',(-0.21419871731156,3.92888130423517,302.727608099971));
#7749=CARTESIAN_POINT('Ctrl Pts',(-0.0980671387366002,3.93348781893119,
302.721737900592));
#7750=CARTESIAN_POINT('Ctrl Pts',(0.0179255588310843,3.93295914984387,302.715867701214));
#7751=CARTESIAN_POINT('Ctrl Pts',(0.139861752424025,3.93240339161486,302.709696711291));
#7752=CARTESIAN_POINT('Ctrl Pts',(0.261643926491458,3.92617228084734,302.703525721368));
#7753=CARTESIAN_POINT('Ctrl Pts',(0.38271089412944,3.91433536778782,302.697354731444));
#7754=CARTESIAN_POINT('Ctrl Pts',(0.503777861767422,3.90249845472831,302.691183741521));
#7755=CARTESIAN_POINT('Ctrl Pts',(0.62412911730201,3.88505588397551,302.685012751598));
#7756=CARTESIAN_POINT('Ctrl Pts',(0.743218086348091,3.86213876966184,302.678841761675));
#7757=CARTESIAN_POINT('Ctrl Pts',(0.856721028788252,3.84029661309877,302.672960230248));
#7758=CARTESIAN_POINT('Ctrl Pts',(0.969443132990848,3.81341149870362,302.667078698821));
#7759=CARTESIAN_POINT('Ctrl Pts',(1.08090273155214,3.7815523644296,302.661197167394));
#7760=CARTESIAN_POINT('Ctrl Pts',(1.19222146759259,3.74973349369523,302.655323069041));
#7761=CARTESIAN_POINT('Ctrl Pts',(1.30228047876846,3.71295321749396,302.649448970687));
#7762=CARTESIAN_POINT('Ctrl Pts',(1.41060724030692,3.67133166760968,302.643574872333));
#7763=CARTESIAN_POINT('Ctrl Pts',(1.51882579907799,3.62975169163398,302.637706641354));
#7764=CARTESIAN_POINT('Ctrl Pts',(1.6253151679036,3.58334020837525,302.631838410375));
#7765=CARTESIAN_POINT('Ctrl Pts',(1.72961760009881,3.5322672545305,302.625970179396));
#7766=CARTESIAN_POINT('Ctrl Pts',(1.83592491773799,3.48021258415634,302.619989150176));
#7767=CARTESIAN_POINT('Ctrl Pts',(1.93995993808236,3.4233155064749,302.614008120956));
#7768=CARTESIAN_POINT('Ctrl Pts',(2.04125864743232,3.36180786694938,302.608027091735));
#7769=CARTESIAN_POINT('Ctrl Pts',(2.14053758619138,3.30152661344821,302.602165316818));
#7770=CARTESIAN_POINT('Ctrl Pts',(2.23718795307342,3.23681717642422,302.5963035419));
#7771=CARTESIAN_POINT('Ctrl Pts',(2.33079809162539,3.16794401088078,302.590441766983));
#7772=CARTESIAN_POINT('Ctrl Pts',(2.4243952839673,3.0990803704431,302.584580802744));
#7773=CARTESIAN_POINT('Ctrl Pts',(2.51495275253663,3.02605439064325,302.578719838506));
#7774=CARTESIAN_POINT('Ctrl Pts',(2.60208919539501,2.94917290425783,302.572858874267));
#7775=CARTESIAN_POINT('Ctrl Pts',(2.68923449153811,2.87228360651741,302.566997314539));
#7776=CARTESIAN_POINT('Ctrl Pts',(2.77295776220374,2.79153829591852,302.561135754812));
#7777=CARTESIAN_POINT('Ctrl Pts',(2.85291259512011,2.70728253505337,302.555274195084));
#7778=CARTESIAN_POINT('Ctrl Pts',(2.93572057434127,2.62002015152389,302.54920346867));
#7779=CARTESIAN_POINT('Ctrl Pts',(3.01448581251738,2.52899244459729,302.543132742256));
#7780=CARTESIAN_POINT('Ctrl Pts',(3.08886794048322,2.43462191032919,302.537062015842));
#7781=CARTESIAN_POINT('Ctrl Pts',(3.16079309263549,2.34336860497818,302.531191816468));
#7782=CARTESIAN_POINT('Ctrl Pts',(3.22861993213251,2.24899019988977,302.525321617094));
#7783=CARTESIAN_POINT('Ctrl Pts',(3.29208474305134,2.15189847450305,302.51945141772));
#7784=CARTESIAN_POINT('Ctrl Pts',(3.35880150757975,2.04983174356193,302.513280427786));
#7785=CARTESIAN_POINT('Ctrl Pts',(3.42069711094658,1.94476672081367,302.507109437852));
#7786=CARTESIAN_POINT('Ctrl Pts',(3.47752041045996,1.83721005735175,302.500938447918));
#7787=CARTESIAN_POINT('Ctrl Pts',(3.53434370997332,1.72965339388984,302.494767457983));
#7788=CARTESIAN_POINT('Ctrl Pts',(3.5860945477062,1.61960559138547,302.488596468049));
#7789=CARTESIAN_POINT('Ctrl Pts',(3.6325812091907,1.5075950247446,302.482425478115));
#7790=CARTESIAN_POINT('Ctrl Pts',(3.68173078294175,1.38916811624636,302.475900993129));
#7791=CARTESIAN_POINT('Ctrl Pts',(3.72513134234822,1.26822460025763,302.469376508143));
#7792=CARTESIAN_POINT('Ctrl Pts',(3.76254653351109,1.14530894660074,302.462852023158));
#7793=CARTESIAN_POINT('Ctrl Pts',(3.79986192435122,1.02272115501065,302.456344941416));
#7794=CARTESIAN_POINT('Ctrl Pts',(3.83122370243373,0.898171951789454,302.449837859675));
#7795=CARTESIAN_POINT('Ctrl Pts',(3.85644381831002,0.772224110099149,302.443330777933));
#7796=CARTESIAN_POINT('Ctrl Pts',(3.88174452838295,0.645873785519059,302.436802901956));
#7797=CARTESIAN_POINT('Ctrl Pts',(3.90086408695092,0.518116083530064,302.430275025979));
#7798=CARTESIAN_POINT('Ctrl Pts',(3.91366178017579,0.38953879189533,302.423747150002));
#7799=CARTESIAN_POINT('Ctrl Pts',(3.92645947340065,0.260961500260597,302.417219274026));
#7800=CARTESIAN_POINT('Ctrl Pts',(3.93293516086949,0.131564860360707,302.410691398049));
#7801=CARTESIAN_POINT('Ctrl Pts',(3.93299951520447,0.00195279323822586,
302.404163522072));
#7802=CARTESIAN_POINT('',(3.93299852553402,-0.00340560526560608,301.154163522075));
#7803=CARTESIAN_POINT('Ctrl Pts',(3.93299951520483,0.00195279250481771,
302.404163522035));
#7804=CARTESIAN_POINT('Ctrl Pts',(3.93305803804962,-0.115914476855165,302.398227169555));
#7805=CARTESIAN_POINT('Ctrl Pts',(3.92781370480953,-0.233779881318091,302.392290817075));
#7806=CARTESIAN_POINT('Ctrl Pts',(3.91729349463852,-0.351141961125049,302.386354464595));
#7807=CARTESIAN_POINT('Ctrl Pts',(3.90677049323188,-0.46853517958927,302.380416537074));
#7808=CARTESIAN_POINT('Ctrl Pts',(3.89096886348083,-0.585424412293054,302.374478609553));
#7809=CARTESIAN_POINT('Ctrl Pts',(3.86996741386578,-0.701313920877823,302.368540682032));
#7810=CARTESIAN_POINT('Ctrl Pts',(3.84895588624024,-0.817259041608628,302.362599905066));
#7811=CARTESIAN_POINT('Ctrl Pts',(3.82273964196988,-0.932203092995342,302.356659128099));
#7812=CARTESIAN_POINT('Ctrl Pts',(3.79144837889095,-1.04566160405993,302.350718351132));
#7813=CARTESIAN_POINT('Ctrl Pts',(3.76011406092106,-1.15927622719358,302.344769400015));
#7814=CARTESIAN_POINT('Ctrl Pts',(3.72369088340339,-1.27140084469433,302.338820448897));
#7815=CARTESIAN_POINT('Ctrl Pts',(3.68235826933376,-1.38156671075605,302.33287149778));
#7816=CARTESIAN_POINT('Ctrl Pts',(3.64099469302163,-1.49181510201818,302.326918090305));
#7817=CARTESIAN_POINT('Ctrl Pts',(3.59471450688456,-1.60010145340699,302.320964682831));
#7818=CARTESIAN_POINT('Ctrl Pts',(3.54374435715108,-1.70597917078722,302.315011275357));
#7819=CARTESIAN_POINT('Ctrl Pts',(3.49268548173506,-1.81204119354598,302.30904750456));
#7820=CARTESIAN_POINT('Ctrl Pts',(3.4369205206017,-1.91568585680902,302.303083733762));
#7821=CARTESIAN_POINT('Ctrl Pts',(3.37672123785625,-2.0164926684247,302.297119962965));
#7822=CARTESIAN_POINT('Ctrl Pts',(3.33933659695329,-2.0790951826234,302.293416373495));
#7823=CARTESIAN_POINT('Ctrl Pts',(3.30024267610691,-2.14060383582257,302.289712784024));
#7824=CARTESIAN_POINT('Ctrl Pts',(3.25951245570129,-2.2009242492935,302.286009194554));
#7825=CARTESIAN_POINT('Ctrl Pts',(3.1948303213986,-2.29671683392635,302.280127663123));
#7826=CARTESIAN_POINT('Ctrl Pts',(3.12581760277882,-2.38980994238612,302.274246131692));
#7827=CARTESIAN_POINT('Ctrl Pts',(3.0527269461845,-2.47978773124617,302.268364600261));
#7828=CARTESIAN_POINT('Ctrl Pts',(2.97972866148272,-2.56965180627423,302.262490501903));
#7829=CARTESIAN_POINT('Ctrl Pts',(2.90266294612185,-2.65640807518571,302.256616403544));
#7830=CARTESIAN_POINT('Ctrl Pts',(2.82182593083435,-2.73966921654255,302.250742305186));
#7831=CARTESIAN_POINT('Ctrl Pts',(2.74106966003267,-2.82284719206225,302.244874074203));
#7832=CARTESIAN_POINT('Ctrl Pts',(2.65654986806645,-2.90253669097776,302.239005843219));
#7833=CARTESIAN_POINT('Ctrl Pts',(2.56860277056448,-2.97838358964195,302.233137612236));
#7834=CARTESIAN_POINT('Ctrl Pts',(2.47896516745839,-3.05568840574616,302.227156583017));
#7835=CARTESIAN_POINT('Ctrl Pts',(2.38576741288148,-3.12900103385408,302.221175553799));
#7836=CARTESIAN_POINT('Ctrl Pts',(2.28940502272061,-3.19798587269263,302.215194524581));
#7837=CARTESIAN_POINT('Ctrl Pts',(2.19496397897108,-3.26559523949984,302.209332749658));
#7838=CARTESIAN_POINT('Ctrl Pts',(2.0974836784843,-3.32904754989813,302.203470974736));
#7839=CARTESIAN_POINT('Ctrl Pts',(1.99736905234799,-3.38806816175863,302.197609199814));
#7840=CARTESIAN_POINT('Ctrl Pts',(1.8972682719864,-3.44708061111453,302.191748235571));
#7841=CARTESIAN_POINT('Ctrl Pts',(1.79453424516496,-3.50166237172745,302.185887271328));
#7842=CARTESIAN_POINT('Ctrl Pts',(1.68959894593192,-3.55158336547317,302.180026307084));
#7843=CARTESIAN_POINT('Ctrl Pts',(1.58465298500415,-3.60150943131951,302.174164747352));
#7844=CARTESIAN_POINT('Ctrl Pts',(1.47750567892787,-3.64677361201655,302.16830318762));
#7845=CARTESIAN_POINT('Ctrl Pts',(1.3686109082234,-3.68719313053872,302.162441627888));
#7846=CARTESIAN_POINT('Ctrl Pts',(1.25583028490952,-3.729054998317,302.15637090148));
#7847=CARTESIAN_POINT('Ctrl Pts',(1.141175598582,-3.76571981855618,302.150300175072));
#7848=CARTESIAN_POINT('Ctrl Pts',(1.02516910154346,-3.7970405993669,302.144229448664));
#7849=CARTESIAN_POINT('Ctrl Pts',(0.912994508079632,-3.82732679836527,302.138359249286));
#7850=CARTESIAN_POINT('Ctrl Pts',(0.799556420830987,-3.85261639866862,302.132489049907));
#7851=CARTESIAN_POINT('Ctrl Pts',(0.685337119420493,-3.87282868621172,302.126618850529));
#7852=CARTESIAN_POINT('Ctrl Pts',(0.565265191280603,-3.8940766566287,302.120447860606));
#7853=CARTESIAN_POINT('Ctrl Pts',(0.44433039437697,-3.90971313830006,302.114276870684));
#7854=CARTESIAN_POINT('Ctrl Pts',(0.32309730988824,-3.91970625536442,302.108105880761));
#7855=CARTESIAN_POINT('Ctrl Pts',(0.20186422539951,-3.92969937242878,302.101934890839));
#7856=CARTESIAN_POINT('Ctrl Pts',(0.0803333767019532,-3.93404917677253,
302.095763900916));
#7857=CARTESIAN_POINT('Ctrl Pts',(-0.0409340283512824,-3.93278697685534,
302.089592910994));
#7858=CARTESIAN_POINT('Ctrl Pts',(-0.156513224452078,-3.93158398210432,
302.083711379563));
#7859=CARTESIAN_POINT('Ctrl Pts',(-0.272225530854058,-3.92527967244628,
302.077829848132));
#7860=CARTESIAN_POINT('Ctrl Pts',(-0.387584714775374,-3.9138557828403,302.071948316701));
#7861=CARTESIAN_POINT('Ctrl Pts',(-0.50279810788512,-3.90244633073363,302.066074218343));
#7862=CARTESIAN_POINT('Ctrl Pts',(-0.617658859820622,-3.88593020698841,
302.060200119985));
#7863=CARTESIAN_POINT('Ctrl Pts',(-0.731680582857664,-3.86434115014048,
302.054326021627));
#7864=CARTESIAN_POINT('Ctrl Pts',(-0.845588414685746,-3.84277365763765,
302.048457790644));
#7865=CARTESIAN_POINT('Ctrl Pts',(-0.958658482396879,-3.81614338804557,
302.04258955966));
#7866=CARTESIAN_POINT('Ctrl Pts',(-1.07041001841095,-3.78453582259244,302.036721328677));
#7867=CARTESIAN_POINT('Ctrl Pts',(-1.18430962529428,-3.75232070136855,302.030740299458));
#7868=CARTESIAN_POINT('Ctrl Pts',(-1.29683905491205,-3.71493500399161,302.02475927024));
#7869=CARTESIAN_POINT('Ctrl Pts',(-1.40750032594185,-3.67252390495604,302.018778241021));
#7870=CARTESIAN_POINT('Ctrl Pts',(-1.51595514862634,-3.63095843057686,302.0129164661));
#7871=CARTESIAN_POINT('Ctrl Pts',(-1.62261521870106,-3.58456625312323,302.007054691177));
#7872=CARTESIAN_POINT('Ctrl Pts',(-1.72702824034959,-3.53353398979478,302.001192916255));
#7873=CARTESIAN_POINT('Ctrl Pts',(-1.83142682175857,-3.48250878418858,301.995331952012));
#7874=CARTESIAN_POINT('Ctrl Pts',(-1.93357860287678,-3.42684494967867,301.989470987769));
#7875=CARTESIAN_POINT('Ctrl Pts',(-2.03305357901847,-3.36677622434878,301.983610023526));
#7876=CARTESIAN_POINT('Ctrl Pts',(-2.13253866207163,-3.30670139588306,301.977748463794));
#7877=CARTESIAN_POINT('Ctrl Pts',(-2.22934604697232,-3.24222099977972,301.971886904062));
#7878=CARTESIAN_POINT('Ctrl Pts',(-2.32307313431842,-3.17361311640345,301.96602534433));
#7879=CARTESIAN_POINT('Ctrl Pts',(-2.42014482347843,-3.10255699679487,301.959954617922));
#7880=CARTESIAN_POINT('Ctrl Pts',(-2.51391188486858,-3.02707359239639,301.953883891514));
#7881=CARTESIAN_POINT('Ctrl Pts',(-2.60396391385376,-2.94751775827516,301.947813165106));
#7882=CARTESIAN_POINT('Ctrl Pts',(-2.69104136209353,-2.87058979667417,301.941942965728));
#7883=CARTESIAN_POINT('Ctrl Pts',(-2.7746450727689,-2.78985453125091,301.936072766349));
#7884=CARTESIAN_POINT('Ctrl Pts',(-2.85444197557788,-2.705669973973,301.930202566971));
#7885=CARTESIAN_POINT('Ctrl Pts',(-2.93832769246163,-2.61717177806302,301.924031577048));
#7886=CARTESIAN_POINT('Ctrl Pts',(-3.01800579814773,-2.52486184285643,301.917860587125));
#7887=CARTESIAN_POINT('Ctrl Pts',(-3.09313863580993,-2.42919377153407,301.911689597202));
#7888=CARTESIAN_POINT('Ctrl Pts',(-3.16827147347212,-2.3335257002117,301.90551860728));
#7889=CARTESIAN_POINT('Ctrl Pts',(-3.23885879805824,-2.23449995813832,301.899347617357));
#7890=CARTESIAN_POINT('Ctrl Pts',(-3.30461754106511,-2.13260214463101,301.893176627434));
#7891=CARTESIAN_POINT('Ctrl Pts',(-3.36729178276125,-2.03548398360718,301.887295096002));
#7892=CARTESIAN_POINT('Ctrl Pts',(-3.42578211398755,-1.93544417487477,301.88141356457));
#7893=CARTESIAN_POINT('Ctrl Pts',(-3.47980540261538,-1.83287843566583,301.875532033138));
#7894=CARTESIAN_POINT('Ctrl Pts',(-3.53376041666969,-1.73044231892676,301.869657934779));
#7895=CARTESIAN_POINT('Ctrl Pts',(-3.58325942579112,-1.62548698185613,301.86378383642));
#7896=CARTESIAN_POINT('Ctrl Pts',(-3.62806261151043,-1.51843692228557,301.857909738061));
#7897=CARTESIAN_POINT('Ctrl Pts',(-3.67282104532781,-1.41149379024019,301.852041507076));
#7898=CARTESIAN_POINT('Ctrl Pts',(-3.71289282816416,-1.30246047562573,301.846173276092));
#7899=CARTESIAN_POINT('Ctrl Pts',(-3.74808441926684,-1.19178529360331,301.840305045107));
#7900=CARTESIAN_POINT('Ctrl Pts',(-3.78395245772235,-1.07898273025041,301.834324015889));
#7901=CARTESIAN_POINT('Ctrl Pts',(-3.81475055041141,-0.964474912250716,
301.828342986671));
#7902=CARTESIAN_POINT('Ctrl Pts',(-3.84032548906766,-0.848757408225265,
301.822361957453));
#7903=CARTESIAN_POINT('Ctrl Pts',(-3.86539049520763,-0.735347167524981,
301.81650018253));
#7904=CARTESIAN_POINT('Ctrl Pts',(-3.88543861199051,-0.620775453322663,
301.810638407607));
#7905=CARTESIAN_POINT('Ctrl Pts',(-3.90037638707522,-0.505522540690357,
301.804776632684));
#7906=CARTESIAN_POINT('Ctrl Pts',(-3.91531209627727,-0.390285567446099,
301.79891566844));
#7907=CARTESIAN_POINT('Ctrl Pts',(-3.92513881639053,-0.274367991409209,
301.793054704196));
#7908=CARTESIAN_POINT('Ctrl Pts',(-3.92981470056569,-0.158257446010553,
301.787193739952));
#7909=CARTESIAN_POINT('Ctrl Pts',(-3.93449105982262,-0.0421351034841711,
301.781332180218));
#7910=CARTESIAN_POINT('Ctrl Pts',(-3.93401552621659,0.0741798359052884,
301.775470620485));
#7911=CARTESIAN_POINT('Ctrl Pts',(-3.92839835717182,0.190198179196717,301.769609060752));
#7912=CARTESIAN_POINT('Ctrl Pts',(-3.92258074240665,0.310356575994506,301.763538334346));
#7913=CARTESIAN_POINT('Ctrl Pts',(-3.91124770501772,0.430196337331117,301.757467607939));
#7914=CARTESIAN_POINT('Ctrl Pts',(-3.89446927364822,0.54917945756368,301.751396881533));
#7915=CARTESIAN_POINT('Ctrl Pts',(-3.87824506408611,0.664232351037048,301.745526682153));
#7916=CARTESIAN_POINT('Ctrl Pts',(-3.85692965953988,0.778483902690411,301.739656482774));
#7917=CARTESIAN_POINT('Ctrl Pts',(-3.83063833044708,0.891458906125011,301.733786283394));
#7918=CARTESIAN_POINT('Ctrl Pts',(-3.80299982682417,1.01022277807323,301.727615293474));
#7919=CARTESIAN_POINT('Ctrl Pts',(-3.76986210004843,1.12757530558744,301.721444303554));
#7920=CARTESIAN_POINT('Ctrl Pts',(-3.73141766823532,1.24298478879724,301.715273313634));
#7921=CARTESIAN_POINT('Ctrl Pts',(-3.6929732364222,1.35839427200703,301.709102323714));
#7922=CARTESIAN_POINT('Ctrl Pts',(-3.64922235292573,1.47186025001474,301.702931333794));
#7923=CARTESIAN_POINT('Ctrl Pts',(-3.60041431324824,1.58287895082258,301.696760343874));
#7924=CARTESIAN_POINT('Ctrl Pts',(-3.55389567958219,1.68869017182402,301.690878812443));
#7925=CARTESIAN_POINT('Ctrl Pts',(-3.5026336969854,1.79261943292805,301.684997281012));
#7926=CARTESIAN_POINT('Ctrl Pts',(-3.44680261578062,1.89421242944076,301.679115749581));
#7927=CARTESIAN_POINT('Ctrl Pts',(-3.39104209383567,1.99567703283474,301.673241651223));
#7928=CARTESIAN_POINT('Ctrl Pts',(-3.33072415434749,2.0948108860578,301.667367552865));
#7929=CARTESIAN_POINT('Ctrl Pts',(-3.26607092977496,2.19117997473482,301.661493454507));
#7930=CARTESIAN_POINT('Ctrl Pts',(-3.20148228442217,2.28745280463135,301.655625223524));
#7931=CARTESIAN_POINT('Ctrl Pts',(-3.13256719626732,2.38096602345882,301.649756992541));
#7932=CARTESIAN_POINT('Ctrl Pts',(-3.05959317090488,2.47131111528926,301.643888761557));
#7933=CARTESIAN_POINT('Ctrl Pts',(-2.98521645002921,2.56339280660591,301.637907732339));
#7934=CARTESIAN_POINT('Ctrl Pts',(-2.90662334810153,2.65218293684628,301.63192670312));
#7935=CARTESIAN_POINT('Ctrl Pts',(-2.82414302670634,2.73728061489975,301.625945673902));
#7936=CARTESIAN_POINT('Ctrl Pts',(-2.743307260511,2.82068155091134,301.62008389898));
#7937=CARTESIAN_POINT('Ctrl Pts',(-2.65873815131181,2.9005356080816,301.614222124058));
#7938=CARTESIAN_POINT('Ctrl Pts',(-2.57078502006558,2.97650018992212,301.608360349136));
#7939=CARTESIAN_POINT('Ctrl Pts',(-2.48284405266893,3.05245426592011,301.602499384893));
#7940=CARTESIAN_POINT('Ctrl Pts',(-2.39152030552613,3.12451966722843,301.59663842065));
#7941=CARTESIAN_POINT('Ctrl Pts',(-2.29719767240283,3.19239281008885,301.590777456407));
#7942=CARTESIAN_POINT('Ctrl Pts',(-2.202865455859,3.26027284903402,301.584915896675));
#7943=CARTESIAN_POINT('Ctrl Pts',(-2.10553408188822,3.32395954225842,301.579054336943));
#7944=CARTESIAN_POINT('Ctrl Pts',(-2.0056174525181,3.383191929843,301.573192777211));
#7945=CARTESIAN_POINT('Ctrl Pts',(-1.90213535078211,3.44453799402405,301.567122050803));
#7946=CARTESIAN_POINT('Ctrl Pts',(-1.79588044885803,3.50110566993863,301.561051324394));
#7947=CARTESIAN_POINT('Ctrl Pts',(-1.68734031573684,3.55265698581908,301.554980597986));
#7948=CARTESIAN_POINT('Ctrl Pts',(-1.58238545874679,3.60250546886673,301.549110398608));
#7949=CARTESIAN_POINT('Ctrl Pts',(-1.47529436655568,3.64766365189979,301.54324019923));
#7950=CARTESIAN_POINT('Ctrl Pts',(-1.36652712562136,3.68796591835405,301.537369999851));
#7951=CARTESIAN_POINT('Ctrl Pts',(-1.2521866229445,3.73033328343394,301.531199009928));
#7952=CARTESIAN_POINT('Ctrl Pts',(-1.1359941536543,3.76733375293836,301.525028020005));
#7953=CARTESIAN_POINT('Ctrl Pts',(-1.01849950972214,3.79883505152511,301.518857030082));
#7954=CARTESIAN_POINT('Ctrl Pts',(-0.901004865789978,3.83033635011185,301.51268604016));
#7955=CARTESIAN_POINT('Ctrl Pts',(-0.782208571438065,3.85633843528389,301.506515050237));
#7956=CARTESIAN_POINT('Ctrl Pts',(-0.662668393150373,3.876771801476,301.500344060314));
#7957=CARTESIAN_POINT('Ctrl Pts',(-0.548735405950678,3.89624671344418,301.494462528883));
#7958=CARTESIAN_POINT('Ctrl Pts',(-0.433759646993851,3.91072625163271,301.488580997451));
#7959=CARTESIAN_POINT('Ctrl Pts',(-0.318216254326227,3.92010553626845,301.48269946602));
#7960=CARTESIAN_POINT('Ctrl Pts',(-0.202818885273205,3.92947296737443,301.476825367662));
#7961=CARTESIAN_POINT('Ctrl Pts',(-0.0868557161747232,3.93375293139621,
301.470951269304));
#7962=CARTESIAN_POINT('Ctrl Pts',(0.0291886673973893,3.93289168700278,301.465077170946));
#7963=CARTESIAN_POINT('Ctrl Pts',(0.145117139415245,3.93203130286792,301.459208939962));
#7964=CARTESIAN_POINT('Ctrl Pts',(0.261126255042988,3.92603992884983,301.453340708978));
#7965=CARTESIAN_POINT('Ctrl Pts',(0.376727709900824,3.91491573761082,301.447472477995));
#7966=CARTESIAN_POINT('Ctrl Pts',(0.494551238172704,3.90357771887599,301.441491448777));
#7967=CARTESIAN_POINT('Ctrl Pts',(0.61195083854817,3.8869074840324,301.435510419558));
#7968=CARTESIAN_POINT('Ctrl Pts',(0.728410600579671,3.86495886096646,301.42952939034));
#7969=CARTESIAN_POINT('Ctrl Pts',(0.842548299559075,3.84344786619184,301.423667615417));
#7970=CARTESIAN_POINT('Ctrl Pts',(0.955782868850346,3.81686710255977,301.417805840495));
#7971=CARTESIAN_POINT('Ctrl Pts',(1.06763594037823,3.78531933907995,301.411944065573));
#7972=CARTESIAN_POINT('Ctrl Pts',(1.17947354271343,3.75377593863126,301.40608310133));
#7973=CARTESIAN_POINT('Ctrl Pts',(1.28992963100695,3.7172670161951,301.400222137087));
#7974=CARTESIAN_POINT('Ctrl Pts',(1.39853934699904,3.67594568715256,301.394361172843));
#7975=CARTESIAN_POINT('Ctrl Pts',(1.50716009801596,3.63462015975734,301.388499613111));
#7976=CARTESIAN_POINT('Ctrl Pts',(1.61393371891261,3.58848140019164,301.382638053379));
#7977=CARTESIAN_POINT('Ctrl Pts',(1.71841438968721,3.5377310504497,301.376776493647));
#7978=CARTESIAN_POINT('Ctrl Pts',(1.82662339823676,3.48516970117424,301.370705767239));
#7979=CARTESIAN_POINT('Ctrl Pts',(1.93237232452568,3.42766169539426,301.364635040831));
#7980=CARTESIAN_POINT('Ctrl Pts',(2.03519394636125,3.3654828183627,301.358564314423));
#7981=CARTESIAN_POINT('Ctrl Pts',(2.13461918480164,3.30535782165038,301.352694115045));
#7982=CARTESIAN_POINT('Ctrl Pts',(2.23130713953981,3.24086593897699,301.346823915666));
#7983=CARTESIAN_POINT('Ctrl Pts',(2.32486611309963,3.17229988433645,301.340953716287));
#7984=CARTESIAN_POINT('Ctrl Pts',(2.42321907281305,3.10022048721204,301.334782726365));
#7985=CARTESIAN_POINT('Ctrl Pts',(2.51811348592935,3.0236386680859,301.328611736443));
#7986=CARTESIAN_POINT('Ctrl Pts',(2.60913605640942,2.94294037301885,301.32244074652));
#7987=CARTESIAN_POINT('Ctrl Pts',(2.70015862688948,2.8622420779518,301.316269756598));
#7988=CARTESIAN_POINT('Ctrl Pts',(2.78730903044843,2.77742772101416,301.310098766675));
#7989=CARTESIAN_POINT('Ctrl Pts',(2.87022196134222,2.68892448622657,301.303927776753));
#7990=CARTESIAN_POINT('Ctrl Pts',(2.94828653660491,2.6055965015734,301.298117637103));
#7991=CARTESIAN_POINT('Ctrl Pts',(3.02286069147831,2.51871501896711,301.292307497454));
#7992=CARTESIAN_POINT('Ctrl Pts',(3.09359853530955,2.42860805860695,301.286497357804));
#7993=CARTESIAN_POINT('Ctrl Pts',(3.16422565332073,2.3386421425102,301.280696312756));
#7994=CARTESIAN_POINT('Ctrl Pts',(3.23102815063106,2.24546112486799,301.274895267708));
#7995=CARTESIAN_POINT('Ctrl Pts',(3.29369747789793,2.14942920890379,301.269094222659));
#7996=CARTESIAN_POINT('Ctrl Pts',(3.3563107355319,2.05348321175363,301.263298367749));
#7997=CARTESIAN_POINT('Ctrl Pts',(3.41479794135421,1.95469173649733,301.257502512839));
#7998=CARTESIAN_POINT('Ctrl Pts',(3.46889144557637,1.85345114281631,301.251706657929));
#7999=CARTESIAN_POINT('Ctrl Pts',(3.52295033287159,1.75227533765814,301.245914512053));
#8000=CARTESIAN_POINT('Ctrl Pts',(3.57262090867942,1.64865390115011,301.240122366178));
#8001=CARTESIAN_POINT('Ctrl Pts',(3.6176798727907,1.54301047890321,301.234330220302));
#8002=CARTESIAN_POINT('Ctrl Pts',(3.66272147733844,1.43740775718586,301.228540305928));
#8003=CARTESIAN_POINT('Ctrl Pts',(3.70315483784618,1.32978498747829,301.222750391554));
#8004=CARTESIAN_POINT('Ctrl Pts',(3.73880385742427,1.22058785661229,301.216960477179));
#8005=CARTESIAN_POINT('Ctrl Pts',(3.77445892735166,1.11137219281629,301.211169580141));
#8006=CARTESIAN_POINT('Ctrl Pts',(3.80532789413077,1.00058203347094,301.205378683103));
#8007=CARTESIAN_POINT('Ctrl Pts',(3.83128397436347,0.888679980524858,301.199587786064));
#8008=CARTESIAN_POINT('Ctrl Pts',(3.85724201819696,0.776769462087923,301.193796450939));
#8009=CARTESIAN_POINT('Ctrl Pts',(3.87828634872675,0.663747296822126,301.188005115815));
#8010=CARTESIAN_POINT('Ctrl Pts',(3.89434122249579,0.550086759311637,301.18221378069));
#8011=CARTESIAN_POINT('Ctrl Pts',(3.9104088514833,0.436335921185449,301.176417844486));
#8012=CARTESIAN_POINT('Ctrl Pts',(3.92147905828884,0.32194611844812,301.170621908282));
#8013=CARTESIAN_POINT('Ctrl Pts',(3.92752796032574,0.207396048321935,301.164825972078));
#8014=CARTESIAN_POINT('Ctrl Pts',(3.93123723255074,0.137152326254839,301.161271822077));
#8015=CARTESIAN_POINT('Ctrl Pts',(3.93305935886409,0.0668483962409372,301.157717672076));
#8016=CARTESIAN_POINT('Ctrl Pts',(3.93299852553402,-0.00340560526561647,
301.154163522075));
#8017=CARTESIAN_POINT('',(3.93299918092051,0.00253828261005724,299.904163521993));
#8018=CARTESIAN_POINT('Ctrl Pts',(3.93299852553333,-0.00340560606263315,
301.154163522035));
#8019=CARTESIAN_POINT('Ctrl Pts',(3.93286544172368,-0.157098786510854,301.146388183894));
#8020=CARTESIAN_POINT('Ctrl Pts',(3.92371953772783,-0.310406465359547,301.138612845754));
#8021=CARTESIAN_POINT('Ctrl Pts',(3.9057186758342,-0.462439861214385,301.130837507614));
#8022=CARTESIAN_POINT('Ctrl Pts',(3.88771781394057,-0.614473257069218,301.123062169474));
#8023=CARTESIAN_POINT('Ctrl Pts',(3.86086214198175,-0.76523283790746,301.115286831334));
#8024=CARTESIAN_POINT('Ctrl Pts',(3.82535752409155,-0.913853824676678,301.107511493194));
#8025=CARTESIAN_POINT('Ctrl Pts',(3.79850061804613,-1.0262758169477,301.101629961768));
#8026=CARTESIAN_POINT('Ctrl Pts',(3.76664036763773,-1.13769397793598,301.095748430341));
#8027=CARTESIAN_POINT('Ctrl Pts',(3.7298670150837,-1.24763017348516,301.089866898915));
#8028=CARTESIAN_POINT('Ctrl Pts',(3.69314013665271,-1.35742743178973,301.083992800562));
#8029=CARTESIAN_POINT('Ctrl Pts',(3.65151263467781,-1.46574606240973,301.078118702208));
#8030=CARTESIAN_POINT('Ctrl Pts',(3.60512548911743,-1.5721193363469,301.072244603855));
#8031=CARTESIAN_POINT('Ctrl Pts',(3.55878467760578,-1.67838635876979,301.066376372876));
#8032=CARTESIAN_POINT('Ctrl Pts',(3.50769384352751,-1.78271151453515,301.060508141897));
#8033=CARTESIAN_POINT('Ctrl Pts',(3.45204316688197,-1.88464505251878,301.054639910918));
#8034=CARTESIAN_POINT('Ctrl Pts',(3.39532278141295,-1.9885379414315,301.048658881698));
#8035=CARTESIAN_POINT('Ctrl Pts',(3.33386558241176,-2.08994590758908,301.042677852478));
#8036=CARTESIAN_POINT('Ctrl Pts',(3.26792377584436,-2.18841568155392,301.036696823258));
#8037=CARTESIAN_POINT('Ctrl Pts',(3.20329676709334,-2.28492209038627,301.03083504834));
#8038=CARTESIAN_POINT('Ctrl Pts',(3.134362568962,-2.37860603237732,301.024973273423));
#8039=CARTESIAN_POINT('Ctrl Pts',(3.0614036416859,-2.46906799069453,301.019111498505));
#8040=CARTESIAN_POINT('Ctrl Pts',(2.98845480457217,-2.5595174381939,301.013250534266));
#8041=CARTESIAN_POINT('Ctrl Pts',(2.91148260371487,-2.64674546771846,301.007389570028));
#8042=CARTESIAN_POINT('Ctrl Pts',(2.83081048851926,-2.73038476740721,301.001528605789));
#8043=CARTESIAN_POINT('Ctrl Pts',(2.75013017683002,-2.81403256506314,300.995667046061));
#8044=CARTESIAN_POINT('Ctrl Pts',(2.66574948938891,-2.89409061163738,300.989805486334));
#8045=CARTESIAN_POINT('Ctrl Pts',(2.57802901917603,-2.97022816906147,300.983943926606));
#8046=CARTESIAN_POINT('Ctrl Pts',(2.48717828995953,-3.04908265531714,300.977873200191));
#8047=CARTESIAN_POINT('Ctrl Pts',(2.3927453270273,-3.12373131025809,300.971802473777));
#8048=CARTESIAN_POINT('Ctrl Pts',(2.29516731291217,-3.19385284660072,300.965731747362));
#8049=CARTESIAN_POINT('Ctrl Pts',(2.20081247655601,-3.26165814215475,300.959861547988));
#8050=CARTESIAN_POINT('Ctrl Pts',(2.10351746537517,-3.32523049700673,300.953991348614));
#8051=CARTESIAN_POINT('Ctrl Pts',(2.00370535464434,-3.38432472611149,300.94812114924));
#8052=CARTESIAN_POINT('Ctrl Pts',(1.89877884510035,-3.44644695906252,300.941950159305));
#8053=CARTESIAN_POINT('Ctrl Pts',(1.79107091742521,-3.50361974134937,300.935779169371));
#8054=CARTESIAN_POINT('Ctrl Pts',(1.68109886722079,-3.55561465834376,300.929608179436));
#8055=CARTESIAN_POINT('Ctrl Pts',(1.57112681701637,-3.60760957533814,300.923437189501));
#8056=CARTESIAN_POINT('Ctrl Pts',(1.45889115246718,-3.65442649152832,300.917266199567));
#8057=CARTESIAN_POINT('Ctrl Pts',(1.34492823469044,-3.69589732589157,300.911095209632));
#8058=CARTESIAN_POINT('Ctrl Pts',(1.23631089938217,-3.73542291552566,300.905213678201));
#8059=CARTESIAN_POINT('Ctrl Pts',(1.12577471544002,-3.77021995865531,300.89933214677));
#8060=CARTESIAN_POINT('Ctrl Pts',(1.01376842338997,-3.80010033864073,300.893450615339));
#8061=CARTESIAN_POINT('Ctrl Pts',(0.90190368477125,-3.8299429558341,300.887576516981));
#8062=CARTESIAN_POINT('Ctrl Pts',(0.788572927624833,-3.85488116269691,300.881702418622));
#8063=CARTESIAN_POINT('Ctrl Pts',(0.674243328308639,-3.87477546887962,300.875828320264));
#8064=CARTESIAN_POINT('Ctrl Pts',(0.560027927726205,-3.89464990352785,300.869960089281));
#8065=CARTESIAN_POINT('Ctrl Pts',(0.444816073097176,-3.90949038943803,300.864091858297));
#8066=CARTESIAN_POINT('Ctrl Pts',(0.329087878767785,-3.91920784955941,300.858223627314));
#8067=CARTESIAN_POINT('Ctrl Pts',(0.211135174855668,-3.92911209720724,300.852242598096));
#8068=CARTESIAN_POINT('Ctrl Pts',(0.092646496011925,-3.93369422362777,300.846261568877));
#8069=CARTESIAN_POINT('Ctrl Pts',(-0.0258609341332851,-3.93291497646285,
300.840280539659));
#8070=CARTESIAN_POINT('Ctrl Pts',(-0.142005473262481,-3.93215126651886,
300.834418764737));
#8071=CARTESIAN_POINT('Ctrl Pts',(-0.258167592749956,-3.92623800412594,
300.828556989815));
#8072=CARTESIAN_POINT('Ctrl Pts',(-0.373858259075998,-3.91519080021915,
300.822695214893));
#8073=CARTESIAN_POINT('Ctrl Pts',(-0.48953292547211,-3.90414512413214,300.81683425065));
#8074=CARTESIAN_POINT('Ctrl Pts',(-0.604735858539051,-3.88796695768332,
300.810973286407));
#8075=CARTESIAN_POINT('Ctrl Pts',(-0.718982318146374,-3.86672386215939,
300.805112322164));
#8076=CARTESIAN_POINT('Ctrl Pts',(-0.833240385484909,-3.84547860828287,
300.799250762432));
#8077=CARTESIAN_POINT('Ctrl Pts',(-0.946541381309225,-3.81916747760979,
300.793389202701));
#8078=CARTESIAN_POINT('Ctrl Pts',(-1.05841062355543,-3.78790917947421,300.787527642969));
#8079=CARTESIAN_POINT('Ctrl Pts',(-1.17427186087287,-3.75553544541017,300.781456916561));
#8080=CARTESIAN_POINT('Ctrl Pts',(-1.28859679337923,-3.71785500023334,300.775386190153));
#8081=CARTESIAN_POINT('Ctrl Pts',(-1.40087642916247,-3.67505567715878,300.769315463745));
#8082=CARTESIAN_POINT('Ctrl Pts',(-1.5094472663012,-3.63367009282944,300.763445264367));
#8083=CARTESIAN_POINT('Ctrl Pts',(-1.61610543337552,-3.58749868482146,300.757575064989));
#8084=CARTESIAN_POINT('Ctrl Pts',(-1.72041322114692,-3.53675944170689,300.751704865611));
#8085=CARTESIAN_POINT('Ctrl Pts',(-1.83006576712542,-3.48342030656267,300.745533875688));
#8086=CARTESIAN_POINT('Ctrl Pts',(-1.93712022061616,-3.42503307634353,300.739362885765));
#8087=CARTESIAN_POINT('Ctrl Pts',(-2.04110095740411,-3.36190360981454,300.733191895842));
#8088=CARTESIAN_POINT('Ctrl Pts',(-2.14508169419205,-3.29877414328555,300.727020905919));
#8089=CARTESIAN_POINT('Ctrl Pts',(-2.24598832120386,-3.23090278988663,300.720849915996));
#8090=CARTESIAN_POINT('Ctrl Pts',(-2.3433850608668,-3.15864456001404,300.714678926073));
#8091=CARTESIAN_POINT('Ctrl Pts',(-2.43621327726425,-3.08977569826034,300.708797394618));
#8092=CARTESIAN_POINT('Ctrl Pts',(-2.52615252292027,-3.01670029628729,300.702915863163));
#8093=CARTESIAN_POINT('Ctrl Pts',(-2.61279857418619,-2.93968920308434,300.697034331708));
#8094=CARTESIAN_POINT('Ctrl Pts',(-2.6993351222681,-2.86277543641601,300.691160233326));
#8095=CARTESIAN_POINT('Ctrl Pts',(-2.78258644826526,-2.78193614210238,300.685286134944));
#8096=CARTESIAN_POINT('Ctrl Pts',(-2.86217875188137,-2.69748434514064,300.679412036562));
#8097=CARTESIAN_POINT('Ctrl Pts',(-2.9416915542995,-2.61311690330777,300.673543805554));
#8098=CARTESIAN_POINT('Ctrl Pts',(-3.01755232388958,-2.52514443481699,300.667675574547));
#8099=CARTESIAN_POINT('Ctrl Pts',(-3.08942220406522,-2.43391853705682,300.661807343539));
#8100=CARTESIAN_POINT('Ctrl Pts',(-3.16267355563161,-2.34093910961853,300.65582631433));
#8101=CARTESIAN_POINT('Ctrl Pts',(-3.23177868287738,-2.24458017523864,300.64984528512));
#8102=CARTESIAN_POINT('Ctrl Pts',(-3.29641986457654,-2.14525175129288,300.643864255911));
#8103=CARTESIAN_POINT('Ctrl Pts',(-3.35977218172926,-2.0479038122441,300.638002480965));
#8104=CARTESIAN_POINT('Ctrl Pts',(-3.41883668120434,-1.94770406333801,300.632140706019));
#8105=CARTESIAN_POINT('Ctrl Pts',(-3.47335695864057,-1.84506922305455,300.626278931072));
#8106=CARTESIAN_POINT('Ctrl Pts',(-3.52786969596439,-1.74244857709051,300.620417966805));
#8107=CARTESIAN_POINT('Ctrl Pts',(-3.57783926793467,-1.63739387307015,300.614557002538));
#8108=CARTESIAN_POINT('Ctrl Pts',(-3.62305499023294,-1.53034686844134,300.608696038271));
#8109=CARTESIAN_POINT('Ctrl Pts',(-3.66827530656344,-1.42328898756495,300.602834478515));
#8110=CARTESIAN_POINT('Ctrl Pts',(-3.70874065281395,-1.3142387830344,300.596972918758));
#8111=CARTESIAN_POINT('Ctrl Pts',(-3.74428857119481,-1.20365779838788,300.591111359002));
#8112=CARTESIAN_POINT('Ctrl Pts',(-3.78110499798921,-1.08913079057624,300.585040632628));
#8113=CARTESIAN_POINT('Ctrl Pts',(-3.8126463413861,-0.972962164740077,300.578969906254));
#8114=CARTESIAN_POINT('Ctrl Pts',(-3.8387889272288,-0.85568018101715,300.57289917988));
#8115=CARTESIAN_POINT('Ctrl Pts',(-3.86406797660831,-0.74227223140965,300.567028980478));
#8116=CARTESIAN_POINT('Ctrl Pts',(-3.88429928560468,-0.627823737477159,
300.561158781076));
#8117=CARTESIAN_POINT('Ctrl Pts',(-3.89942361896982,-0.512820085234843,
300.555288581674));
#8118=CARTESIAN_POINT('Ctrl Pts',(-3.91532292688877,-0.391923617624727,
300.549117591814));
#8119=CARTESIAN_POINT('Ctrl Pts',(-3.92557798633627,-0.270414119568538,
300.542946601953));
#8120=CARTESIAN_POINT('Ctrl Pts',(-3.93018200398618,-0.148857030546762,
300.536775612093));
#8121=CARTESIAN_POINT('Ctrl Pts',(-3.93478602163608,-0.0272999415249911,
300.530604622233));
#8122=CARTESIAN_POINT('Ctrl Pts',(-3.9337390725465,0.0943042179038661,300.524433632373));
#8123=CARTESIAN_POINT('Ctrl Pts',(-3.92709733580095,0.215396181825655,300.518262642513));
#8124=CARTESIAN_POINT('Ctrl Pts',(-3.92076713854647,0.330808166209259,300.512381111135));
#8125=CARTESIAN_POINT('Ctrl Pts',(-3.90933474442532,0.446126778362399,300.506499579757));
#8126=CARTESIAN_POINT('Ctrl Pts',(-3.89280348111259,0.560865453952848,300.50061804838));
#8127=CARTESIAN_POINT('Ctrl Pts',(-3.87629310999253,0.67545912292934,300.494743950075));
#8128=CARTESIAN_POINT('Ctrl Pts',(-3.85469674392071,0.789473908932605,300.488869851771));
#8129=CARTESIAN_POINT('Ctrl Pts',(-3.82806966980634,0.902425400301178,300.482995753466));
#8130=CARTESIAN_POINT('Ctrl Pts',(-3.80146919228729,1.0152640694688,300.477127522536));
#8131=CARTESIAN_POINT('Ctrl Pts',(-3.76984809661646,1.12704115817196,300.471259291606));
#8132=CARTESIAN_POINT('Ctrl Pts',(-3.7333131120623,1.23728016524299,300.465391060676));
#8133=CARTESIAN_POINT('Ctrl Pts',(-3.69607585718077,1.3496381709814,300.459410031437));
#8134=CARTESIAN_POINT('Ctrl Pts',(-3.65373391493465,1.46039792426789,300.453429002199));
#8135=CARTESIAN_POINT('Ctrl Pts',(-3.60645441286819,1.56906837578977,300.44744797296));
#8136=CARTESIAN_POINT('Ctrl Pts',(-3.56011760594133,1.67557207212198,300.441586198091));
#8137=CARTESIAN_POINT('Ctrl Pts',(-3.50903848509052,1.78006861691531,300.435724423222));
#8138=CARTESIAN_POINT('Ctrl Pts',(-3.45342355262258,1.88211444024842,300.429862648352));
#8139=CARTESIAN_POINT('Ctrl Pts',(-3.39781631165343,1.98414615072926,300.424001684162));
#8140=CARTESIAN_POINT('Ctrl Pts',(-3.33767470359273,2.08372745228817,300.418140719971));
#8141=CARTESIAN_POINT('Ctrl Pts',(-3.27325131613854,2.18043913499032,300.41227975578));
#8142=CARTESIAN_POINT('Ctrl Pts',(-3.20882138309925,2.27716064385303,300.4064181961));
#8143=CARTESIAN_POINT('Ctrl Pts',(-3.14010903414613,2.37101161153109,300.40055663642));
#8144=CARTESIAN_POINT('Ctrl Pts',(-3.06740993958069,2.46160217390251,300.39469507674));
#8145=CARTESIAN_POINT('Ctrl Pts',(-2.99211661447514,2.55542541482317,300.388624350257));
#8146=CARTESIAN_POINT('Ctrl Pts',(-2.91254699513114,2.64575083864331,300.382553623775));
#8147=CARTESIAN_POINT('Ctrl Pts',(-2.82907379728921,2.73218419025724,300.376482897293));
#8148=CARTESIAN_POINT('Ctrl Pts',(-2.74835787123007,2.81576249081697,300.370612697965));
#8149=CARTESIAN_POINT('Ctrl Pts',(-2.66399252507181,2.8957015404752,300.364742498637));
#8150=CARTESIAN_POINT('Ctrl Pts',(-2.57635019690619,2.97168448239403,300.358872299309));
#8151=CARTESIAN_POINT('Ctrl Pts',(-2.48421705019534,3.05156081249447,300.352701309249));
#8152=CARTESIAN_POINT('Ctrl Pts',(-2.38846261491229,3.12706454378054,300.34653031919));
#8153=CARTESIAN_POINT('Ctrl Pts',(-2.28955502976753,3.19787847887724,300.34035932913));
#8154=CARTESIAN_POINT('Ctrl Pts',(-2.19064744462277,3.26869241397394,300.334188339071));
#8155=CARTESIAN_POINT('Ctrl Pts',(-2.08858718539605,3.33481632871924,300.328017349011));
#8156=CARTESIAN_POINT('Ctrl Pts',(-1.98387193327471,3.39598898001228,300.321846358952));
#8157=CARTESIAN_POINT('Ctrl Pts',(-1.88406849122799,3.45429224562534,300.315964827501));
#8158=CARTESIAN_POINT('Ctrl Pts',(-1.78153192407064,3.50828608442161,300.31008329605));
#8159=CARTESIAN_POINT('Ctrl Pts',(-1.67667012221064,3.55770520157112,300.304201764598));
#8160=CARTESIAN_POINT('Ctrl Pts',(-1.57194084459013,3.60706186289017,300.298327666221));
#8161=CARTESIAN_POINT('Ctrl Pts',(-1.46489254604916,3.65185512709511,300.292453567843));
#8162=CARTESIAN_POINT('Ctrl Pts',(-1.35595994737082,3.69186424738588,300.286579469465));
#8163=CARTESIAN_POINT('Ctrl Pts',(-1.24713615661101,3.73183340434929,300.280711238463));
#8164=CARTESIAN_POINT('Ctrl Pts',(-1.13643219418239,3.76702778222883,300.27484300746));
#8165=CARTESIAN_POINT('Ctrl Pts',(-1.02430452134268,3.79727392316606,300.268974776457));
#8166=CARTESIAN_POINT('Ctrl Pts',(-0.910021548104855,3.82810145064198,300.262993747246));
#8167=CARTESIAN_POINT('Ctrl Pts',(-0.794259959272325,3.85378836150439,300.257012718035));
#8168=CARTESIAN_POINT('Ctrl Pts',(-0.677521633416676,3.87420358735217,300.251031688824));
#8169=CARTESIAN_POINT('Ctrl Pts',(-0.563110924343218,3.89421175903031,300.245169913884));
#8170=CARTESIAN_POINT('Ctrl Pts',(-0.447762491068235,3.90915644642779,300.239308138944));
#8171=CARTESIAN_POINT('Ctrl Pts',(-0.331960282241142,3.9189655996212,300.233446364005));
#8172=CARTESIAN_POINT('Ctrl Pts',(-0.216174088779671,3.92877339621549,300.227585399744));
#8173=CARTESIAN_POINT('Ctrl Pts',(-0.0999346547999836,3.93344703631298,
300.221724435484));
#8174=CARTESIAN_POINT('Ctrl Pts',(0.0162690097339698,3.93296635115561,300.215863471223));
#8175=CARTESIAN_POINT('Ctrl Pts',(0.132484480846329,3.93248561715945,300.210001911474));
#8176=CARTESIAN_POINT('Ctrl Pts',(0.24866376348413,3.92684951855367,300.204140351725));
#8177=CARTESIAN_POINT('Ctrl Pts',(0.364318601617826,3.91609000873515,300.198278791977));
#8178=CARTESIAN_POINT('Ctrl Pts',(0.484100520961988,3.90494655154769,300.192208065595));
#8179=CARTESIAN_POINT('Ctrl Pts',(0.603319392767887,3.88830724208551,300.186137339213));
#8180=CARTESIAN_POINT('Ctrl Pts',(0.721440848529659,3.8662659119715,300.18006661283));
#8181=CARTESIAN_POINT('Ctrl Pts',(0.835660540600444,3.84495264655145,300.174196413437));
#8182=CARTESIAN_POINT('Ctrl Pts',(0.948853777666821,3.81858875686659,300.168326214043));
#8183=CARTESIAN_POINT('Ctrl Pts',(1.06055093603876,3.78731048530053,300.162456014649));
#8184=CARTESIAN_POINT('Ctrl Pts',(1.1779714846907,3.75442950729085,300.156285024773));
#8185=CARTESIAN_POINT('Ctrl Pts',(1.29373807183774,3.71611734535367,300.150114034897));
#8186=CARTESIAN_POINT('Ctrl Pts',(1.40732806354347,3.67258992014668,300.143943045021));
#8187=CARTESIAN_POINT('Ctrl Pts',(1.5209180552492,3.62906249493968,300.137772055144));
#8188=CARTESIAN_POINT('Ctrl Pts',(1.63233100231152,3.58032008001792,300.131601065268));
#8189=CARTESIAN_POINT('Ctrl Pts',(1.74107469043959,3.52663407831188,300.125430075392));
#8190=CARTESIAN_POINT('Ctrl Pts',(1.84471761549434,3.47546628782131,300.119548543762));
#8191=CARTESIAN_POINT('Ctrl Pts',(1.94626996586553,3.41964332459357,300.113667012133));
#8192=CARTESIAN_POINT('Ctrl Pts',(2.04528561597544,3.35935942540895,300.107785480503));
#8193=CARTESIAN_POINT('Ctrl Pts',(2.14417613023306,3.29915171293921,300.101911381946));
#8194=CARTESIAN_POINT('Ctrl Pts',(2.24053597152125,3.23449448939036,300.096037283388));
#8195=CARTESIAN_POINT('Ctrl Pts',(2.33394140918747,3.16562892621356,300.090163184831));
#8196=CARTESIAN_POINT('Ctrl Pts',(2.42725354834476,3.09683214976397,300.084294953647));
#8197=CARTESIAN_POINT('Ctrl Pts',(2.51761682462389,3.02383563859343,300.078426722464));
#8198=CARTESIAN_POINT('Ctrl Pts',(2.60463499396856,2.94692476120351,300.07255849128));
#8199=CARTESIAN_POINT('Ctrl Pts',(2.69332580907198,2.86853551838904,300.066577462136));
#8200=CARTESIAN_POINT('Ctrl Pts',(2.77854121907186,2.78608009786493,300.060596432993));
#8201=CARTESIAN_POINT('Ctrl Pts',(2.85989533302364,2.69990512502747,300.054615403849));
#8202=CARTESIAN_POINT('Ctrl Pts',(2.93962735067599,2.61544837020939,300.048753628727));
#8203=CARTESIAN_POINT('Ctrl Pts',(3.01565032958605,2.52741932838689,300.042891853604));
#8204=CARTESIAN_POINT('Ctrl Pts',(3.08763751046008,2.43618217791688,300.037030078482));
#8205=CARTESIAN_POINT('Ctrl Pts',(3.15961473555994,2.34495764547769,300.031169114039));
#8206=CARTESIAN_POINT('Ctrl Pts',(3.22755701759814,2.25052620994329,300.025308149596));
#8207=CARTESIAN_POINT('Ctrl Pts',(3.29117810562532,2.15328485738708,300.019447185153));
#8208=CARTESIAN_POINT('Ctrl Pts',(3.35480565771185,2.05603362486979,300.013585625221));
#8209=CARTESIAN_POINT('Ctrl Pts',(3.41411091754167,1.95597225239564,300.00772406529));
#8210=CARTESIAN_POINT('Ctrl Pts',(3.46885154752756,1.85352581347433,300.001862505358));
#8211=CARTESIAN_POINT('Ctrl Pts',(3.5255455635491,1.74742363578561,299.995791779231));
#8212=CARTESIAN_POINT('Ctrl Pts',(3.57734286546249,1.63876341190897,299.989721053104));
#8213=CARTESIAN_POINT('Ctrl Pts',(3.62402734993076,1.52804278963446,299.983650326976));
#8214=CARTESIAN_POINT('Ctrl Pts',(3.66916976537472,1.42097946043933,299.977780127402));
#8215=CARTESIAN_POINT('Ctrl Pts',(3.70953171259698,1.31199011410391,299.971909927827));
#8216=CARTESIAN_POINT('Ctrl Pts',(3.7449681527168,1.20154173258232,299.966039728252));
#8217=CARTESIAN_POINT('Ctrl Pts',(3.78222036087105,1.08543396089785,299.959868738849));
#8218=CARTESIAN_POINT('Ctrl Pts',(3.8140287861813,0.967714182437371,299.953697749445));
#8219=CARTESIAN_POINT('Ctrl Pts',(3.84028567852364,0.848937516738543,299.947526760042));
#8220=CARTESIAN_POINT('Ctrl Pts',(3.86654257086599,0.73016085103972,299.941355770639));
#8221=CARTESIAN_POINT('Ctrl Pts',(3.8872479110456,0.610327823693746,299.935184781235));
#8222=CARTESIAN_POINT('Ctrl Pts',(3.90235701070326,0.489998735728107,299.929013791832));
#8223=CARTESIAN_POINT('Ctrl Pts',(3.92263821027235,0.328478969342776,299.920730368567));
#8224=CARTESIAN_POINT('Ctrl Pts',(3.93289389566743,0.165674836823054,299.912446945301));
#8225=CARTESIAN_POINT('Ctrl Pts',(3.93299918091997,0.00253828344068463,
299.904163522035));
#8226=CARTESIAN_POINT('',(3.93299999531041,0.000192063329847205,298.65416352207));
#8227=CARTESIAN_POINT('Ctrl Pts',(3.93299918092051,0.00253828261004938,
299.904163521993));
#8228=CARTESIAN_POINT('Ctrl Pts',(3.93307284838121,-0.111607424191687,299.898367658443));
#8229=CARTESIAN_POINT('Ctrl Pts',(3.92817312010893,-0.225939896070615,299.892571794893));
#8230=CARTESIAN_POINT('Ctrl Pts',(3.91827769750935,-0.339983654314229,299.886775931344));
#8231=CARTESIAN_POINT('Ctrl Pts',(3.90839302762208,-0.453903488621041,299.880986365782));
#8232=CARTESIAN_POINT('Ctrl Pts',(3.89352349123848,-0.567534813198981,299.87519680022));
#8233=CARTESIAN_POINT('Ctrl Pts',(3.87369882539846,-0.680401653515468,299.869407234658));
#8234=CARTESIAN_POINT('Ctrl Pts',(3.85389011836459,-0.793177636309329,299.863622329682));
#8235=CARTESIAN_POINT('Ctrl Pts',(3.82913428684059,-0.90518994231623,299.857837424706));
#8236=CARTESIAN_POINT('Ctrl Pts',(3.79951285333144,-1.01596804938404,299.85205251973));
#8237=CARTESIAN_POINT('Ctrl Pts',(3.76990412234892,-1.12669865159845,299.846270095489));
#8238=CARTESIAN_POINT('Ctrl Pts',(3.73543404440196,-1.23619569720181,299.840487671247));
#8239=CARTESIAN_POINT('Ctrl Pts',(3.69623502513004,-1.34399986570011,299.834705247006));
#8240=CARTESIAN_POINT('Ctrl Pts',(3.65704277323311,-1.45178542273193,299.82892382105));
#8241=CARTESIAN_POINT('Ctrl Pts',(3.61312334777438,-1.55787828487982,299.823142395094));
#8242=CARTESIAN_POINT('Ctrl Pts',(3.56465843411753,-1.66183610746511,299.817360969139));
#8243=CARTESIAN_POINT('Ctrl Pts',(3.51618947118613,-1.76580261579298,299.811579060141));
#8244=CARTESIAN_POINT('Ctrl Pts',(3.46317444555771,-1.86763334583981,299.805797151144));
#8245=CARTESIAN_POINT('Ctrl Pts',(3.40584204794065,-1.96690847384403,299.800015242147));
#8246=CARTESIAN_POINT('Ctrl Pts',(3.34845515127121,-2.06627797083725,299.79422783698));
#8247=CARTESIAN_POINT('Ctrl Pts',(3.28674289880943,-2.16308664588207,299.788440431813));
#8248=CARTESIAN_POINT('Ctrl Pts',(3.22097858646294,-2.25694172400335,299.782653026647));
#8249=CARTESIAN_POINT('Ctrl Pts',(3.15518287829366,-2.35084160845339,299.776862858578));
#8250=CARTESIAN_POINT('Ctrl Pts',(3.0853315172225,-2.44178475207879,299.771072690509));
#8251=CARTESIAN_POINT('Ctrl Pts',(3.01173836458176,-2.52941120091345,299.765282522441));
#8252=CARTESIAN_POINT('Ctrl Pts',(2.93802850167194,-2.61717661520962,299.759483171832));
#8253=CARTESIAN_POINT('Ctrl Pts',(2.86056528084323,-2.7016145152527,299.753683821223));
#8254=CARTESIAN_POINT('Ctrl Pts',(2.77969994058407,-2.78240134421994,299.747884470615));
#8255=CARTESIAN_POINT('Ctrl Pts',(2.70864684660833,-2.85338545350848,299.7427888165));
#8256=CARTESIAN_POINT('Ctrl Pts',(2.63496785311061,-2.92155124361669,299.737693162386));
#8257=CARTESIAN_POINT('Ctrl Pts',(2.55892100415829,-2.98670592701684,299.732597508272));
#8258=CARTESIAN_POINT('Ctrl Pts',(2.47114582301482,-3.06190909738593,299.726715976438));
#8259=CARTESIAN_POINT('Ctrl Pts',(2.37991126581068,-3.13336075403482,299.720834444605));
#8260=CARTESIAN_POINT('Ctrl Pts',(2.28557123593582,-3.20072696827811,299.714952912772));
#8261=CARTESIAN_POINT('Ctrl Pts',(2.19135043294819,-3.26800804513021,299.709078814016));
#8262=CARTESIAN_POINT('Ctrl Pts',(2.09403229515043,-3.33121371110383,299.70320471526));
#8263=CARTESIAN_POINT('Ctrl Pts',(1.99400508672333,-3.3900490725241,299.697330616504));
#8264=CARTESIAN_POINT('Ctrl Pts',(1.89407779108197,-3.44882566588563,299.691462385128));
#8265=CARTESIAN_POINT('Ctrl Pts',(1.79144716066328,-3.50324043080484,299.685594153751));
#8266=CARTESIAN_POINT('Ctrl Pts',(1.68653130241257,-3.5530411151551,299.679725922374));
#8267=CARTESIAN_POINT('Ctrl Pts',(1.57959877747443,-3.60379905594698,299.673744893305));
#8268=CARTESIAN_POINT('Ctrl Pts',(1.47029261830429,-3.64976344901614,299.667763864236));
#8269=CARTESIAN_POINT('Ctrl Pts',(1.35908319432061,-3.69071563127198,299.661782835166));
#8270=CARTESIAN_POINT('Ctrl Pts',(1.25009113839858,-3.73085128145942,299.655921059865));
#8271=CARTESIAN_POINT('Ctrl Pts',(1.13927141555826,-3.76617259484685,299.650059284564));
#8272=CARTESIAN_POINT('Ctrl Pts',(1.02708730306685,-3.79652218113879,299.644197509262));
#8273=CARTESIAN_POINT('Ctrl Pts',(0.914918705661378,-3.82686757007668,299.638336544646));
#8274=CARTESIAN_POINT('Ctrl Pts',(0.801386491275514,-3.85224249181793,299.632475580029));
#8275=CARTESIAN_POINT('Ctrl Pts',(0.686968190187093,-3.87253969710719,299.626614615412));
#8276=CARTESIAN_POINT('Ctrl Pts',(0.57253826402901,-3.89283896462272,299.620753055313));
#8277=CARTESIAN_POINT('Ctrl Pts',(0.457222477677544,-3.90805941818161,299.614891495214));
#8278=CARTESIAN_POINT('Ctrl Pts',(0.341506935893272,-3.91814522609063,299.609029935114));
#8279=CARTESIAN_POINT('Ctrl Pts',(0.221662164058092,-3.92859093916418,299.602959209248));
#8280=CARTESIAN_POINT('Ctrl Pts',(0.10138904847765,-3.93352866481383,299.596888483381));
#8281=CARTESIAN_POINT('Ctrl Pts',(-0.018769876342918,-3.93295521100127,
299.590817757514));
#8282=CARTESIAN_POINT('Ctrl Pts',(-0.134959752667976,-3.93240069931886,
299.584947557787));
#8283=CARTESIAN_POINT('Ctrl Pts',(-0.251042448199745,-3.92669342784198,
299.57907735806));
#8284=CARTESIAN_POINT('Ctrl Pts',(-0.366531549930758,-3.91588350476688,
299.573207158333));
#8285=CARTESIAN_POINT('Ctrl Pts',(-0.487938316693847,-3.90451968090961,
299.567036169396));
#8286=CARTESIAN_POINT('Ctrl Pts',(-0.608688522382004,-3.88751650818293,
299.560865180459));
#8287=CARTESIAN_POINT('Ctrl Pts',(-0.72822935608746,-3.86499301486205,299.554694191522));
#8288=CARTESIAN_POINT('Ctrl Pts',(-0.847770189792916,-3.84246952154117,
299.548523202586));
#8289=CARTESIAN_POINT('Ctrl Pts',(-0.966101160652827,-3.81442589648558,
299.542352213649));
#8290=CARTESIAN_POINT('Ctrl Pts',(-1.08268947065561,-3.78104119392152,299.536181224712));
#8291=CARTESIAN_POINT('Ctrl Pts',(-1.19380909825172,-3.74922243167823,299.530299691713));
#8292=CARTESIAN_POINT('Ctrl Pts',(-1.30370387739374,-3.71244979142711,299.524418158714));
#8293=CARTESIAN_POINT('Ctrl Pts',(-1.4119001488038,-3.67083464212266,299.518536625715));
#8294=CARTESIAN_POINT('Ctrl Pts',(-1.51995968209177,-3.62927208591862,299.51266252578));
#8295=CARTESIAN_POINT('Ctrl Pts',(-1.62632459580339,-3.58287933886022,299.506788425845));
#8296=CARTESIAN_POINT('Ctrl Pts',(-1.73053487590191,-3.53181795160611,299.50091432591));
#8297=CARTESIAN_POINT('Ctrl Pts',(-1.83464106516137,-3.48080756721503,299.495046093342));
#8298=CARTESIAN_POINT('Ctrl Pts',(-1.93659653428927,-3.42513799930513,299.489177860774));
#8299=CARTESIAN_POINT('Ctrl Pts',(-2.0359604134839,-3.36501919678424,299.483309628206));
#8300=CARTESIAN_POINT('Ctrl Pts',(-2.13723421255566,-3.30374482247153,299.477328599579));
#8301=CARTESIAN_POINT('Ctrl Pts',(-2.23581535812041,-3.23784856028069,299.471347570952));
#8302=CARTESIAN_POINT('Ctrl Pts',(-2.33126221818643,-3.16760247980337,299.465366542324));
#8303=CARTESIAN_POINT('Ctrl Pts',(-2.42480602102345,-3.09875699344899,299.45950476581));
#8304=CARTESIAN_POINT('Ctrl Pts',(-2.51533901974359,-3.0257337942245,299.453642989296));
#8305=CARTESIAN_POINT('Ctrl Pts',(-2.60247462395827,-2.94883279140294,299.447781212782));
#8306=CARTESIAN_POINT('Ctrl Pts',(-2.68959817738942,-2.87194242392783,299.441920246947));
#8307=CARTESIAN_POINT('Ctrl Pts',(-2.7733249620421,-2.79117559181146,299.436059281112));
#8308=CARTESIAN_POINT('Ctrl Pts',(-2.8533023795244,-2.70687172414956,299.430198315277));
#8309=CARTESIAN_POINT('Ctrl Pts',(-2.93328792288949,-2.62255929102794,299.424336753955));
#8310=CARTESIAN_POINT('Ctrl Pts',(-3.00952305837299,-2.53470940671756,299.418475192632));
#8311=CARTESIAN_POINT('Ctrl Pts',(-3.08169337346136,-2.44369698448157,299.41261363131));
#8312=CARTESIAN_POINT('Ctrl Pts',(-3.15643900057268,-2.34943689199591,299.40654290713));
#8313=CARTESIAN_POINT('Ctrl Pts',(-3.22682399373476,-2.25178471465513,299.40047218295));
#8314=CARTESIAN_POINT('Ctrl Pts',(-3.29254678082895,-2.15119145964578,299.39440145877));
#8315=CARTESIAN_POINT('Ctrl Pts',(-3.35609866619722,-2.05392091933815,299.388531257821));
#8316=CARTESIAN_POINT('Ctrl Pts',(-3.41529131848942,-1.9539009192602,299.382661056872));
#8317=CARTESIAN_POINT('Ctrl Pts',(-3.46989856633695,-1.85156499732869,299.376790855923));
#8318=CARTESIAN_POINT('Ctrl Pts',(-3.52730385002353,-1.743985456858,299.370619870127));
#8319=CARTESIAN_POINT('Ctrl Pts',(-3.5796411496913,-1.63384685421397,299.364448884332));
#8320=CARTESIAN_POINT('Ctrl Pts',(-3.62670522905839,-1.52167610926915,299.358277898537));
#8321=CARTESIAN_POINT('Ctrl Pts',(-3.67376930842548,-1.40950536432434,299.352106912741));
#8322=CARTESIAN_POINT('Ctrl Pts',(-3.7155600546627,-1.29530299077279,299.345935926946));
#8323=CARTESIAN_POINT('Ctrl Pts',(-3.75193335139576,-1.17961227811693,299.339764941151));
#8324=CARTESIAN_POINT('Ctrl Pts',(-3.78660050105938,-1.06934822149961,299.333883415214));
#8325=CARTESIAN_POINT('Ctrl Pts',(-3.816458629075,-0.95737701844418,299.328001889278));
#8326=CARTESIAN_POINT('Ctrl Pts',(-3.84133971506152,-0.844155313607069,
299.322120363341));
#8327=CARTESIAN_POINT('Ctrl Pts',(-3.86618935631761,-0.731076698424104,
299.31624627048));
#8328=CARTESIAN_POINT('Ctrl Pts',(-3.8860743777425,-0.616751123344073,299.310372177619));
#8329=CARTESIAN_POINT('Ctrl Pts',(-3.90087615535629,-0.501651493143109,
299.304498084758));
#8330=CARTESIAN_POINT('Ctrl Pts',(-3.91566314813149,-0.386666830853354,
299.298629859268));
#8331=CARTESIAN_POINT('Ctrl Pts',(-3.92537694518395,-0.270910057636561,
299.292761633778));
#8332=CARTESIAN_POINT('Ctrl Pts',(-3.92994986024603,-0.154864766658676,
299.286893408288));
#8333=CARTESIAN_POINT('Ctrl Pts',(-3.93461068114802,-0.03658871944896,299.280912377009));
#8334=CARTESIAN_POINT('Ctrl Pts',(-3.93393083611978,0.0819866281317321,
299.274931345729));
#8335=CARTESIAN_POINT('Ctrl Pts',(-3.92789406105627,0.200342818985095,299.26895031445));
#8336=CARTESIAN_POINT('Ctrl Pts',(-3.92197765932922,0.316338986575359,299.263088544976));
#8337=CARTESIAN_POINT('Ctrl Pts',(-3.91091600534963,0.432124226900779,299.257226775502));
#8338=CARTESIAN_POINT('Ctrl Pts',(-3.89474639354974,0.547210681485,299.251365006028));
#8339=CARTESIAN_POINT('Ctrl Pts',(-3.87857901792365,0.662281220206955,299.245504047207));
#8340=CARTESIAN_POINT('Ctrl Pts',(-3.85730514658442,0.776652757677666,299.239643088385));
#8341=CARTESIAN_POINT('Ctrl Pts',(-3.83101378264864,0.889844029679433,299.233782129564));
#8342=CARTESIAN_POINT('Ctrl Pts',(-3.80471974729484,1.00304680284201,299.227920575221));
#8343=CARTESIAN_POINT('Ctrl Pts',(-3.77340729903819,1.11506867100497,299.222059020878));
#8344=CARTESIAN_POINT('Ctrl Pts',(-3.73721609237713,1.22544068762116,299.216197466535));
#8345=CARTESIAN_POINT('Ctrl Pts',(-3.69973333972014,1.33975152112892,299.210126732456));
#8346=CARTESIAN_POINT('Ctrl Pts',(-3.65701725589882,1.45229209397296,299.204055998377));
#8347=CARTESIAN_POINT('Ctrl Pts',(-3.60927807499095,1.56256224752476,299.197985264299));
#8348=CARTESIAN_POINT('Ctrl Pts',(-3.56311590490991,1.66918974900922,299.192115070179));
#8349=CARTESIAN_POINT('Ctrl Pts',(-3.51225750028227,1.77369411483187,299.186244876059));
#8350=CARTESIAN_POINT('Ctrl Pts',(-3.45694005662018,1.87564774009804,299.180374681939));
#8351=CARTESIAN_POINT('Ctrl Pts',(-3.39878794744905,1.98282583717512,299.174203677881));
#8352=CARTESIAN_POINT('Ctrl Pts',(-3.33570797303367,2.08718439722229,299.168032673823));
#8353=CARTESIAN_POINT('Ctrl Pts',(-3.26802679801522,2.18826183247215,299.161861669765));
#8354=CARTESIAN_POINT('Ctrl Pts',(-3.20034562299678,2.28933926772201,299.155690665707));
#8355=CARTESIAN_POINT('Ctrl Pts',(-3.12806361391963,2.3871352009875,299.149519661649));
#8356=CARTESIAN_POINT('Ctrl Pts',(-3.05155477111898,2.48123003344329,299.143348657591));
#8357=CARTESIAN_POINT('Ctrl Pts',(-2.97863477264787,2.57091110542987,299.137467120373));
#8358=CARTESIAN_POINT('Ctrl Pts',(-2.90164055790344,2.65751939637476,299.131585583154));
#8359=CARTESIAN_POINT('Ctrl Pts',(-2.82086064564473,2.74066309820321,299.125704045936));
#8360=CARTESIAN_POINT('Ctrl Pts',(-2.74018282334396,2.82370172270753,299.119829941826));
#8361=CARTESIAN_POINT('Ctrl Pts',(-2.6557291034131,2.90328417357108,299.113955837717));
#8362=CARTESIAN_POINT('Ctrl Pts',(-2.56782878914213,2.97905090752959,299.108081733607));
#8363=CARTESIAN_POINT('Ctrl Pts',(-2.48001627511971,3.05474196100699,299.102213496914));
#8364=CARTESIAN_POINT('Ctrl Pts',(-2.38876432530163,3.12662461202969,299.096345260222));
#8365=CARTESIAN_POINT('Ctrl Pts',(-2.29443922687332,3.19437593814268,299.090477023529));
#8366=CARTESIAN_POINT('Ctrl Pts',(-2.19830115407132,3.2634294777712,299.084495996467));
#8367=CARTESIAN_POINT('Ctrl Pts',(-2.09897087987745,3.32819092747019,299.078514969405));
#8368=CARTESIAN_POINT('Ctrl Pts',(-1.99687211445838,3.38836107262767,299.072533942342));
#8369=CARTESIAN_POINT('Ctrl Pts',(-1.89680894051811,3.44733157708178,299.066672161851));
#8370=CARTESIAN_POINT('Ctrl Pts',(-1.79408701708441,3.50189194129735,299.06081038136));
#8371=CARTESIAN_POINT('Ctrl Pts',(-1.6891340297507,3.55180450328254,299.054948600869));
#8372=CARTESIAN_POINT('Ctrl Pts',(-1.58419555842818,3.60171016187864,299.049087631119));
#8373=CARTESIAN_POINT('Ctrl Pts',(-1.4770270086691,3.6469691198377,299.043226661369));
#8374=CARTESIAN_POINT('Ctrl Pts',(-1.36807905174343,3.68739050117841,299.037365691618));
#8375=CARTESIAN_POINT('Ctrl Pts',(-1.25912002669872,3.72781598896291,299.031504126447));
#8376=CARTESIAN_POINT('Ctrl Pts',(-1.14838162121822,3.76340277991293,299.025642561276));
#8377=CARTESIAN_POINT('Ctrl Pts',(-1.0363321333408,3.7940090549978,299.019780996105));
#8378=CARTESIAN_POINT('Ctrl Pts',(-0.920284477162809,3.82570742823645,299.013710277599));
#8379=CARTESIAN_POINT('Ctrl Pts',(-0.802830885538338,3.85206308744197,299.007639559092));
#8380=CARTESIAN_POINT('Ctrl Pts',(-0.684504583102838,3.87297591984655,299.001568840586));
#8381=CARTESIAN_POINT('Ctrl Pts',(-0.570086560908655,3.89319800802947,298.995698635987));
#8382=CARTESIAN_POINT('Ctrl Pts',(-0.45485299105735,3.90833114852157,298.989828431388));
#8383=CARTESIAN_POINT('Ctrl Pts',(-0.339291410563918,3.91833770095401,298.983958226788));
#8384=CARTESIAN_POINT('Ctrl Pts',(-0.217808817370258,3.92885695772802,298.977787251329));
#8385=CARTESIAN_POINT('Ctrl Pts',(-0.0959642399790542,3.93371035044302,
298.971616275869));
#8386=CARTESIAN_POINT('Ctrl Pts',(0.0256771420902181,3.93291618069519,298.96544530041));
#8387=CARTESIAN_POINT('Ctrl Pts',(0.147318524159488,3.93212201094737,298.95927432495));
#8388=CARTESIAN_POINT('Ctrl Pts',(0.268756194200433,3.92568037681522,298.953103349491));
#8389=CARTESIAN_POINT('Ctrl Pts',(0.38943393405726,3.91367221558023,298.946932374031));
#8390=CARTESIAN_POINT('Ctrl Pts',(0.504451614871845,3.90222726427658,298.941050831283));
#8391=CARTESIAN_POINT('Ctrl Pts',(0.61914961719036,3.8856892634248,298.935169288535));
#8392=CARTESIAN_POINT('Ctrl Pts',(0.733042001889961,3.86408312843618,298.929287745786));
#8393=CARTESIAN_POINT('Ctrl Pts',(0.846790451664222,3.84250429885025,298.923413636015));
#8394=CARTESIAN_POINT('Ctrl Pts',(0.959734907611862,3.81587014979798,298.917539526243));
#8395=CARTESIAN_POINT('Ctrl Pts',(1.07139388683557,3.78425740922197,298.911665416471));
#8396=CARTESIAN_POINT('Ctrl Pts',(1.18294133665201,3.75267624470229,298.905797173993));
#8397=CARTESIAN_POINT('Ctrl Pts',(1.2932054699101,3.71612649243231,298.899928931514));
#8398=CARTESIAN_POINT('Ctrl Pts',(1.4017149891287,3.67473592102234,298.894060689036));
#8399=CARTESIAN_POINT('Ctrl Pts',(1.51230996591828,3.63254985921544,298.888079664096));
#8400=CARTESIAN_POINT('Ctrl Pts',(1.62108176049001,3.58533506396183,298.882098639155));
#8401=CARTESIAN_POINT('Ctrl Pts',(1.72754722542983,3.53328028663304,298.876117614215));
#8402=CARTESIAN_POINT('Ctrl Pts',(1.83189018265554,3.48226327931258,298.870255827674));
#8403=CARTESIAN_POINT('Ctrl Pts',(1.9340175308548,3.42659767280112,298.864394041133));
#8404=CARTESIAN_POINT('Ctrl Pts',(2.03349529856749,3.36650944907391,298.858532254591));
#8405=CARTESIAN_POINT('Ctrl Pts',(2.13295930903918,3.30642953522531,298.852671278703));
#8406=CARTESIAN_POINT('Ctrl Pts',(2.22977411533169,3.24192843335955,298.846810302816));
#8407=CARTESIAN_POINT('Ctrl Pts',(2.32353212690091,3.17327708453884,298.840949326928));
#8408=CARTESIAN_POINT('Ctrl Pts',(2.41729966469621,3.10461876043935,298.835087755539));
#8409=CARTESIAN_POINT('Ctrl Pts',(2.50800945809351,3.03180959439804,298.829226184151));
#8410=CARTESIAN_POINT('Ctrl Pts',(2.59528514511845,2.95516226551564,298.823364612762));
#8411=CARTESIAN_POINT('Ctrl Pts',(2.68567479791148,2.87578018693958,298.817293902571));
#8412=CARTESIAN_POINT('Ctrl Pts',(2.77238035214324,2.7922812540297,298.81122319238));
#8413=CARTESIAN_POINT('Ctrl Pts',(2.85502448286709,2.7050553048375,298.805152482189));
#8414=CARTESIAN_POINT('Ctrl Pts',(2.93493910016204,2.62071019421887,298.799282271233));
#8415=CARTESIAN_POINT('Ctrl Pts',(3.01105610668511,2.53288072346202,298.793412060277));
#8416=CARTESIAN_POINT('Ctrl Pts',(3.08307548192846,2.441953024268,298.787541849322));
#8417=CARTESIAN_POINT('Ctrl Pts',(3.15878462992905,2.34636682107791,298.781370889513));
#8418=CARTESIAN_POINT('Ctrl Pts',(3.22996484918045,2.24735694818931,298.775199929705));
#8419=CARTESIAN_POINT('Ctrl Pts',(3.29632003099506,2.14540514897787,298.769028969896));
#8420=CARTESIAN_POINT('Ctrl Pts',(3.36267521280966,2.04345334976642,298.762858010088));
#8421=CARTESIAN_POINT('Ctrl Pts',(3.42420515436349,1.93856010947014,298.756687050279));
#8422=CARTESIAN_POINT('Ctrl Pts',(3.4806709553237,1.83123420150618,298.750516090471));
#8423=CARTESIAN_POINT('Ctrl Pts',(3.53742991076748,1.72335108775417,298.744313092783));
#8424=CARTESIAN_POINT('Ctrl Pts',(3.58923891626138,1.61269480481861,298.738110095095));
#8425=CARTESIAN_POINT('Ctrl Pts',(3.63583421788449,1.49973282289222,298.731907097407));
#8426=CARTESIAN_POINT('Ctrl Pts',(3.68450000718221,1.38175131360728,298.725428466129));
#8427=CARTESIAN_POINT('Ctrl Pts',(3.7274778434829,1.26125475726895,298.71894983485));
#8428=CARTESIAN_POINT('Ctrl Pts',(3.76451967885686,1.13880665062135,298.712471203572));
#8429=CARTESIAN_POINT('Ctrl Pts',(3.79983468351734,1.02206687751698,298.706294595652));
#8430=CARTESIAN_POINT('Ctrl Pts',(3.82975445226548,0.903553774660709,298.700117987731));
#8431=CARTESIAN_POINT('Ctrl Pts',(3.85411226710301,0.783777795402547,298.69394137981));
#8432=CARTESIAN_POINT('Ctrl Pts',(3.87843452805374,0.664176647164188,298.687773787575));
#8433=CARTESIAN_POINT('Ctrl Pts',(3.89721093602318,0.543316630173132,298.681606195341));
#8434=CARTESIAN_POINT('Ctrl Pts',(3.91032465648131,0.421722753612261,298.675438603106));
#8435=CARTESIAN_POINT('Ctrl Pts',(3.92341474746994,0.300347975728007,298.669282124188));
#8436=CARTESIAN_POINT('Ctrl Pts',(3.93086245247844,0.178242315916746,298.663125645271));
#8437=CARTESIAN_POINT('Ctrl Pts',(3.93260215939012,0.0559397529508584,298.656969166353));
#8438=CARTESIAN_POINT('Ctrl Pts',(3.9328664337595,0.037361087495771,298.656033951592));
#8439=CARTESIAN_POINT('Ctrl Pts',(3.93299908769365,0.0187778949398582,298.655098736831));
#8440=CARTESIAN_POINT('Ctrl Pts',(3.93299999531041,0.00019206332985904,
298.65416352207));
#8441=CARTESIAN_POINT('',(3.93299891020702,-0.00292785080898043,297.404163522073));
#8442=CARTESIAN_POINT('Ctrl Pts',(3.93299999531044,0.000192062627323755,
298.654163522035));
#8443=CARTESIAN_POINT('Ctrl Pts',(3.93300592546174,-0.121243769823802,298.648053029623));
#8444=CARTESIAN_POINT('Ctrl Pts',(3.92738333505017,-0.242584282912523,298.641942537212));
#8445=CARTESIAN_POINT('Ctrl Pts',(3.91618452274351,-0.363301230144049,298.6358320448));
#8446=CARTESIAN_POINT('Ctrl Pts',(3.90497215809457,-0.484164264062538,298.629714157721));
#8447=CARTESIAN_POINT('Ctrl Pts',(3.88817014637699,-0.604401871430454,298.623596270643));
#8448=CARTESIAN_POINT('Ctrl Pts',(3.86588221445863,-0.723494093916756,298.617478383565));
#8449=CARTESIAN_POINT('Ctrl Pts',(3.84354528529558,-0.842848125833726,298.611347047073));
#8450=CARTESIAN_POINT('Ctrl Pts',(3.81569839813161,-0.961051387962721,298.605215710581));
#8451=CARTESIAN_POINT('Ctrl Pts',(3.78249599553529,-1.07759595570858,298.599084374089));
#8452=CARTESIAN_POINT('Ctrl Pts',(3.74925373452515,-1.19428043145043,298.592945677126));
#8453=CARTESIAN_POINT('Ctrl Pts',(3.71064324573644,-1.3093019018455,298.586806980162));
#8454=CARTESIAN_POINT('Ctrl Pts',(3.66686763707445,-1.42217113322414,298.580668283198));
#8455=CARTESIAN_POINT('Ctrl Pts',(3.62299912652175,-1.53527989902203,298.574516558511));
#8456=CARTESIAN_POINT('Ctrl Pts',(3.57394373112134,-1.6462269692045,298.568364833823));
#8457=CARTESIAN_POINT('Ctrl Pts',(3.51995162947914,-1.75454539015871,298.562213109135));
#8458=CARTESIAN_POINT('Ctrl Pts',(3.49621550882068,-1.8021645609467,298.55950867506));
#8459=CARTESIAN_POINT('Ctrl Pts',(3.47152586032443,-1.84927605671103,298.556804240986));
#8460=CARTESIAN_POINT('Ctrl Pts',(3.44590658279842,-1.89584198250447,298.554099806911));
#8461=CARTESIAN_POINT('Ctrl Pts',(3.39018977189996,-1.99711356907094,298.548218203037));
#8462=CARTESIAN_POINT('Ctrl Pts',(3.32991504275857,-2.09609001452669,298.542336599164));
#8463=CARTESIAN_POINT('Ctrl Pts',(3.26529624385002,-2.1923342445665,298.536454995291));
#8464=CARTESIAN_POINT('Ctrl Pts',(3.2007591122629,-2.28845683804536,298.530580824778));
#8465=CARTESIAN_POINT('Ctrl Pts',(3.1318890575964,-2.38185374478624,298.524706654265));
#8466=CARTESIAN_POINT('Ctrl Pts',(3.05894582285887,-2.47211234631727,298.518832483753));
#8467=CARTESIAN_POINT('Ctrl Pts',(2.98607545158111,-2.56228078795882,298.512964180986));
#8468=CARTESIAN_POINT('Ctrl Pts',(2.90914025137754,-2.64931684198198,298.50709587822));
#8469=CARTESIAN_POINT('Ctrl Pts',(2.82844289897526,-2.73283731078827,298.501227575453));
#8470=CARTESIAN_POINT('Ctrl Pts',(2.74619577248773,-2.81796177098077,298.495246573282));
#8471=CARTESIAN_POINT('Ctrl Pts',(2.66004074138595,-2.89943385882113,298.489265571111));
#8472=CARTESIAN_POINT('Ctrl Pts',(2.57034120142409,-2.97688345560618,298.48328456894));
#8473=CARTESIAN_POINT('Ctrl Pts',(2.48242870531812,-3.05279005867983,298.477422723603));
#8474=CARTESIAN_POINT('Ctrl Pts',(2.3911119504255,-3.12483268317989,298.471560878266));
#8475=CARTESIAN_POINT('Ctrl Pts',(2.29676926178821,-3.19270104427346,298.465699032929));
#8476=CARTESIAN_POINT('Ctrl Pts',(2.20243963070255,-3.26056001200925,298.459837998904));
#8477=CARTESIAN_POINT('Ctrl Pts',(2.10508523294911,-3.32424562487915,298.453976964878));
#8478=CARTESIAN_POINT('Ctrl Pts',(2.00511537172842,-3.38348952208491,298.448115930853));
#8479=CARTESIAN_POINT('Ctrl Pts',(1.90513536553249,-3.44273943138134,298.442254302048));
#8480=CARTESIAN_POINT('Ctrl Pts',(1.80253972250091,-3.49754651902391,298.436392673244));
#8481=CARTESIAN_POINT('Ctrl Pts',(1.69776385742003,-3.54768754041816,298.430531044439));
#8482=CARTESIAN_POINT('Ctrl Pts',(1.58925218067232,-3.59961635342422,298.424460417681));
#8483=CARTESIAN_POINT('Ctrl Pts',(1.47840233594215,-3.64653994187821,298.418389790924));
#8484=CARTESIAN_POINT('Ctrl Pts',(1.36572103526904,-3.68826450431957,298.412319164166));
#8485=CARTESIAN_POINT('Ctrl Pts',(1.25675877473323,-3.72861194987016,298.406448898112));
#8486=CARTESIAN_POINT('Ctrl Pts',(1.14608446214156,-3.76409807287149,298.400578632057));
#8487=CARTESIAN_POINT('Ctrl Pts',(1.03417106279053,-3.79459868930651,298.394708366002));
#8488=CARTESIAN_POINT('Ctrl Pts',(0.916528013255468,-3.82666085121851,298.388537558893));
#8489=CARTESIAN_POINT('Ctrl Pts',(0.797516160316329,-3.85321339277487,298.382366751785));
#8490=CARTESIAN_POINT('Ctrl Pts',(0.677694799480092,-3.87417330004191,298.376195944676));
#8491=CARTESIAN_POINT('Ctrl Pts',(0.557873438643857,-3.89513320730896,298.370025137567));
#8492=CARTESIAN_POINT('Ctrl Pts',(0.437243095715267,-3.91050048441079,298.363854330459));
#8493=CARTESIAN_POINT('Ctrl Pts',(0.316365446062836,-3.92025533665059,298.35768352335));
#8494=CARTESIAN_POINT('Ctrl Pts',(0.201152958180538,-3.92955300912109,298.351801922895));
#8495=CARTESIAN_POINT('Ctrl Pts',(0.0853446993142111,-3.93378238818516,
298.345920322439));
#8496=CARTESIAN_POINT('Ctrl Pts',(-0.0305767527499009,-3.9328811401047,
298.340038721984));
#8497=CARTESIAN_POINT('Ctrl Pts',(-0.146351724133139,-3.93198103085947,
298.334164553637));
#8498=CARTESIAN_POINT('Ctrl Pts',(-0.262239196010664,-3.92596319167233,
298.328290385291));
#8499=CARTESIAN_POINT('Ctrl Pts',(-0.377751715330621,-3.91481706361418,
298.322416216944));
#8500=CARTESIAN_POINT('Ctrl Pts',(-0.493148872743679,-3.90368206715107,
298.316547915107));
#8501=CARTESIAN_POINT('Ctrl Pts',(-0.608171414906144,-3.88742900935181,
298.31067961327));
#8502=CARTESIAN_POINT('Ctrl Pts',(-0.722332788267097,-3.86609937055351,
298.304811311433));
#8503=CARTESIAN_POINT('Ctrl Pts',(-0.838686638799827,-3.84436009454808,
298.298830308447));
#8504=CARTESIAN_POINT('Ctrl Pts',(-0.954145466794198,-3.81734723524644,
298.292849305462));
#8505=CARTESIAN_POINT('Ctrl Pts',(-1.06820018125089,-3.78516015153594,298.286868302477));
#8506=CARTESIAN_POINT('Ctrl Pts',(-1.17998265929118,-3.75361430974246,298.281006455047));
#8507=CARTESIAN_POINT('Ctrl Pts',(-1.29041603865742,-3.71709861804354,298.275144607617));
#8508=CARTESIAN_POINT('Ctrl Pts',(-1.39903293763322,-3.67575785919276,298.269282760187));
#8509=CARTESIAN_POINT('Ctrl Pts',(-1.50763482412505,-3.6344228142547,298.263421722952));
#8510=CARTESIAN_POINT('Ctrl Pts',(-1.61442034475976,-3.58826417486692,298.257560685717));
#8511=CARTESIAN_POINT('Ctrl Pts',(-1.71894003852442,-3.53747567397398,298.251699648482));
#8512=CARTESIAN_POINT('Ctrl Pts',(-1.82347035873041,-3.48668200945105,298.245838015359));
#8513=CARTESIAN_POINT('Ctrl Pts',(-1.92573402373538,-3.43125772765636,298.239976382237));
#8514=CARTESIAN_POINT('Ctrl Pts',(-2.02530483839693,-3.37144320900797,298.234114749114));
#8515=CARTESIAN_POINT('Ctrl Pts',(-2.12842578464202,-3.30949604323273,298.228044123337));
#8516=CARTESIAN_POINT('Ctrl Pts',(-2.22865786308579,-3.24283997869521,298.22197349756));
#8517=CARTESIAN_POINT('Ctrl Pts',(-2.32556017139335,-3.17179111689735,298.215902871783));
#8518=CARTESIAN_POINT('Ctrl Pts',(-2.41926435143361,-3.10308712569383,298.210032598714));
#8519=CARTESIAN_POINT('Ctrl Pts',(-2.50985479538895,-3.03027602921799,298.204162325646));
#8520=CARTESIAN_POINT('Ctrl Pts',(-2.59696729089442,-2.95368412157165,298.198292052577));
#8521=CARTESIAN_POINT('Ctrl Pts',(-2.68853951702541,-2.87317108557035,298.192121250446));
#8522=CARTESIAN_POINT('Ctrl Pts',(-2.77626788162017,-2.78848024315026,298.185950448315));
#8523=CARTESIAN_POINT('Ctrl Pts',(-2.859774970519,-2.70003261424618,298.179779646183));
#8524=CARTESIAN_POINT('Ctrl Pts',(-2.94328205941782,-2.6115849853421,298.173608844052));
#8525=CARTESIAN_POINT('Ctrl Pts',(-3.02256758638687,-2.51938101103282,298.167438041921));
#8526=CARTESIAN_POINT('Ctrl Pts',(-3.09730558529359,-2.42387852651677,298.16126723979));
#8527=CARTESIAN_POINT('Ctrl Pts',(-3.16853413426333,-2.33286052369905,298.155386198175));
#8528=CARTESIAN_POINT('Ctrl Pts',(-3.23586214076153,-2.23855339493931,298.149505156561));
#8529=CARTESIAN_POINT('Ctrl Pts',(-3.29897171895252,-2.1413254300903,298.143624114946));
#8530=CARTESIAN_POINT('Ctrl Pts',(-3.36200152243356,-2.04422036786429,298.137750507359));
#8531=CARTESIAN_POINT('Ctrl Pts',(-3.42082328052744,-1.9442021551057,298.131876899773));
#8532=CARTESIAN_POINT('Ctrl Pts',(-3.4751596251509,-1.8416716807621,298.126003292186));
#8533=CARTESIAN_POINT('Ctrl Pts',(-3.52944168790985,-1.73924363409106,298.120135552318));
#8534=CARTESIAN_POINT('Ctrl Pts',(-3.57924705908134,-1.63430868024482,298.11426781245));
#8535=CARTESIAN_POINT('Ctrl Pts',(-3.6243422919032,-1.52729563317711,298.108400072582));
#8536=CARTESIAN_POINT('Ctrl Pts',(-3.67030959908303,-1.41821311382871,298.1024188594));
#8537=CARTESIAN_POINT('Ctrl Pts',(-3.71138246354779,-1.30697165608777,298.096437646219));
#8538=CARTESIAN_POINT('Ctrl Pts',(-3.74736324720497,-1.19405095933861,298.090456433038));
#8539=CARTESIAN_POINT('Ctrl Pts',(-3.78262259370264,-1.0833943930066,298.084595146912));
#8540=CARTESIAN_POINT('Ctrl Pts',(-3.81299202521437,-0.971125709909917,
298.078733860787));
#8541=CARTESIAN_POINT('Ctrl Pts',(-3.83833487108371,-0.857714648016914,
298.072872574661));
#8542=CARTESIAN_POINT('Ctrl Pts',(-3.8636742192528,-0.744319238584625,298.067012097483));
#8543=CARTESIAN_POINT('Ctrl Pts',(-3.88398827162279,-0.629782165769389,
298.061151620304));
#8544=CARTESIAN_POINT('Ctrl Pts',(-3.89919108151134,-0.514585182319152,
298.055291143126));
#8545=CARTESIAN_POINT('Ctrl Pts',(-3.91439544207652,-0.399376448852254,
298.049430068182));
#8546=CARTESIAN_POINT('Ctrl Pts',(-3.92448746988109,-0.283508079287484,
298.043568993239));
#8547=CARTESIAN_POINT('Ctrl Pts',(-3.92943296570268,-0.16746811054364,298.037707918296));
#8548=CARTESIAN_POINT('Ctrl Pts',(-3.93455594236022,-0.0472637725635806,
298.03163650479));
#8549=CARTESIAN_POINT('Ctrl Pts',(-3.93415603527685,0.0731242358104111,
298.025565091285));
#8550=CARTESIAN_POINT('Ctrl Pts',(-3.92825415593846,0.193153530519733,298.019493677779));
#8551=CARTESIAN_POINT('Ctrl Pts',(-3.92254833354875,0.309195522892783,298.013623953047));
#8552=CARTESIAN_POINT('Ctrl Pts',(-3.91170037762075,0.42490184480052,298.007754228316));
#8553=CARTESIAN_POINT('Ctrl Pts',(-3.89578194842871,0.539788857144138,298.001884503584));
#8554=CARTESIAN_POINT('Ctrl Pts',(-3.87904306292674,0.660597293836267,297.995712245691));
#8555=CARTESIAN_POINT('Ctrl Pts',(-3.85669719999763,0.780499192984246,297.989539987799));
#8556=CARTESIAN_POINT('Ctrl Pts',(-3.82888795165656,0.898947191807865,297.983367729907));
#8557=CARTESIAN_POINT('Ctrl Pts',(-3.80107870331549,1.01739519063148,297.977195472014));
#8558=CARTESIAN_POINT('Ctrl Pts',(-3.76780628045255,1.13438880639514,297.971023214122));
#8559=CARTESIAN_POINT('Ctrl Pts',(-3.7292734174472,1.24940336878114,297.96485095623));
#8560=CARTESIAN_POINT('Ctrl Pts',(-3.69255030673762,1.35901610394514,297.958968587461));
#8561=CARTESIAN_POINT('Ctrl Pts',(-3.6509313368372,1.46718474982083,297.953086218692));
#8562=CARTESIAN_POINT('Ctrl Pts',(-3.60454886705646,1.57344096330368,297.947203849924));
#8563=CARTESIAN_POINT('Ctrl Pts',(-3.55822502384188,1.67956287093865,297.941328916358));
#8564=CARTESIAN_POINT('Ctrl Pts',(-3.50714981889474,1.78377677975772,297.935453982793));
#8565=CARTESIAN_POINT('Ctrl Pts',(-3.45150513642287,1.88563021116193,297.929579049227));
#8566=CARTESIAN_POINT('Ctrl Pts',(-3.39591605660351,1.98738186606743,297.923709986158));
#8567=CARTESIAN_POINT('Ctrl Pts',(-3.33576677859773,2.08677737638179,297.917840923088));
#8568=CARTESIAN_POINT('Ctrl Pts',(-3.27128668580881,2.18338554067988,297.911971860019));
#8569=CARTESIAN_POINT('Ctrl Pts',(-3.2055799235782,2.28183157893004,297.905991143879));
#8570=CARTESIAN_POINT('Ctrl Pts',(-3.13537605516695,2.37738273490431,297.900010427739));
#8571=CARTESIAN_POINT('Ctrl Pts',(-3.06096638708415,2.46961004556206,297.8940297116));
#8572=CARTESIAN_POINT('Ctrl Pts',(-2.98802634681497,2.56001582113692,297.888167117567));
#8573=CARTESIAN_POINT('Ctrl Pts',(-2.91104538687808,2.64722750833493,297.882304523535));
#8574=CARTESIAN_POINT('Ctrl Pts',(-2.83034034309815,2.7308721211787,297.876441929502));
#8575=CARTESIAN_POINT('Ctrl Pts',(-2.74964654562697,2.81450507808255,297.870580152427));
#8576=CARTESIAN_POINT('Ctrl Pts',(-2.6652299821397,2.89457165299403,297.864718375351));
#8577=CARTESIAN_POINT('Ctrl Pts',(-2.57744546206122,2.97073457079222,297.858856598276));
#8578=CARTESIAN_POINT('Ctrl Pts',(-2.48965213151049,3.04690513266334,297.852994232884));
#8579=CARTESIAN_POINT('Ctrl Pts',(-2.39849048336277,3.11917098878944,297.847131867493));
#8580=CARTESIAN_POINT('Ctrl Pts',(-2.30434908434721,3.18723458463104,297.841269502102));
#8581=CARTESIAN_POINT('Ctrl Pts',(-2.20688028290387,3.25770386996115,297.835199932982));
#8582=CARTESIAN_POINT('Ctrl Pts',(-2.10621757909698,3.32366806059187,297.829130363863));
#8583=CARTESIAN_POINT('Ctrl Pts',(-2.00282454310868,3.38484605994446,297.823060794743));
#8584=CARTESIAN_POINT('Ctrl Pts',(-1.90281440835841,3.44402238551146,297.817189814946));
#8585=CARTESIAN_POINT('Ctrl Pts',(-1.8002502124232,3.49872067762816,297.811318835148));
#8586=CARTESIAN_POINT('Ctrl Pts',(-1.69557517532176,3.54873411582674,297.80544785535));
#8587=CARTESIAN_POINT('Ctrl Pts',(-1.58558909679209,3.60128515467582,297.79927899157));
#8588=CARTESIAN_POINT('Ctrl Pts',(-1.47327284269019,3.64866325818106,297.79311012779));
#8589=CARTESIAN_POINT('Ctrl Pts',(-1.35916125131522,3.69068688632932,297.78694126401));
#8590=CARTESIAN_POINT('Ctrl Pts',(-1.24504965994025,3.73271051447759,297.780772400229));
#8591=CARTESIAN_POINT('Ctrl Pts',(-1.12914324806311,3.76937957736814,297.774603536449));
#8592=CARTESIAN_POINT('Ctrl Pts',(-1.0119904910506,3.80057419951554,297.768434672669));
#8593=CARTESIAN_POINT('Ctrl Pts',(-0.900289521454252,3.83031715758936,297.762552881381));
#8594=CARTESIAN_POINT('Ctrl Pts',(-0.787096555945675,3.85517935855739,297.756671090093));
#8595=CARTESIAN_POINT('Ctrl Pts',(-0.672875318114343,3.87501326530278,297.750789298805));
#8596=CARTESIAN_POINT('Ctrl Pts',(-0.558798247404457,3.89482213819898,297.744914931363));
#8597=CARTESIAN_POINT('Ctrl Pts',(-0.443695887817354,3.90961526946071,297.739040563922));
#8598=CARTESIAN_POINT('Ctrl Pts',(-0.328046006161694,3.91929519401657,297.73316619648));
#8599=CARTESIAN_POINT('Ctrl Pts',(-0.212511464138736,3.92896546461578,297.727297687647));
#8600=CARTESIAN_POINT('Ctrl Pts',(-0.0964308943236152,3.93353263860112,
297.721429178814));
#8601=CARTESIAN_POINT('Ctrl Pts',(0.0197095274428665,3.93295061430066,297.715560669981));
#8602=CARTESIAN_POINT('Ctrl Pts',(0.138074782256221,3.93235744050653,297.709579741611));
#8603=CARTESIAN_POINT('Ctrl Pts',(0.256501777629808,3.92641568171508,297.703598813241));
#8604=CARTESIAN_POINT('Ctrl Pts',(0.374471899212748,3.91513215571326,297.697617884872));
#8605=CARTESIAN_POINT('Ctrl Pts',(0.490097659054271,3.90407286162977,297.691755812526));
#8606=CARTESIAN_POINT('Ctrl Pts',(0.605284107964331,3.88788219072501,297.685893740181));
#8607=CARTESIAN_POINT('Ctrl Pts',(0.719545481487535,3.8666191046017,297.680031667836));
#8608=CARTESIAN_POINT('Ctrl Pts',(0.833791184565131,3.84535893461728,297.674170399448));
#8609=CARTESIAN_POINT('Ctrl Pts',(0.947111659863042,3.81902780818591,297.66830913106));
#8610=CARTESIAN_POINT('Ctrl Pts',(1.05903003137945,3.78773605107806,297.662447862673));
#8611=CARTESIAN_POINT('Ctrl Pts',(1.17095989457509,3.75644108096032,297.656585992455));
#8612=CARTESIAN_POINT('Ctrl Pts',(1.28148697124422,3.72018457847325,297.650724122237));
#8613=CARTESIAN_POINT('Ctrl Pts',(1.3901489438384,3.67912692278276,297.64486225202));
#8614=CARTESIAN_POINT('Ctrl Pts',(1.50267500266412,3.63660923173433,297.63879193011));
#8615=CARTESIAN_POINT('Ctrl Pts',(1.61320039289943,3.5889427325439,297.632721608201));
#8616=CARTESIAN_POINT('Ctrl Pts',(1.72123492817387,3.53635961435404,297.626651286292));
#8617=CARTESIAN_POINT('Ctrl Pts',(1.82571360206621,3.4855072230919,297.620780763671));
#8618=CARTESIAN_POINT('Ctrl Pts',(1.92786247186775,3.43005702704061,297.61491024105));
#8619=CARTESIAN_POINT('Ctrl Pts',(2.0272648534531,3.37026500648744,297.609039718429));
#8620=CARTESIAN_POINT('Ctrl Pts',(2.13174187482091,3.30742051413899,297.602869496876));
#8621=CARTESIAN_POINT('Ctrl Pts',(2.23318414193663,3.23977947730182,297.596699275322));
#8622=CARTESIAN_POINT('Ctrl Pts',(2.33114523187613,3.16768857495512,297.590529053769));
#8623=CARTESIAN_POINT('Ctrl Pts',(2.42910632181563,3.09559767260841,297.584358832216));
#8624=CARTESIAN_POINT('Ctrl Pts',(2.52358587443011,3.01905728729746,297.578188610662));
#8625=CARTESIAN_POINT('Ctrl Pts',(2.61418148415182,2.93845948890193,297.572018389109));
#8626=CARTESIAN_POINT('Ctrl Pts',(2.69924849442303,2.86278017325948,297.566224705487));
#8627=CARTESIAN_POINT('Ctrl Pts',(2.7811840106951,2.7832633871791,297.560431021865));
#8628=CARTESIAN_POINT('Ctrl Pts',(2.85961492825546,2.70020211504593,297.554637338244));
#8629=CARTESIAN_POINT('Ctrl Pts',(2.93794564118625,2.61724696335945,297.548851056727));
#8630=CARTESIAN_POINT('Ctrl Pts',(3.01278036575709,2.53075663294805,297.543064775211));
#8631=CARTESIAN_POINT('Ctrl Pts',(3.08377951424885,2.44106388845092,297.537278493694));
#8632=CARTESIAN_POINT('Ctrl Pts',(3.15470070274579,2.35146963028841,297.531498565754));
#8633=CARTESIAN_POINT('Ctrl Pts',(3.22179443066285,2.25868028457932,297.525718637813));
#8634=CARTESIAN_POINT('Ctrl Pts',(3.28475908251103,2.16306420844628,297.519938709873));
#8635=CARTESIAN_POINT('Ctrl Pts',(3.34768560904992,2.06750602817017,297.514162281698));
#8636=CARTESIAN_POINT('Ctrl Pts',(3.40648779386134,1.96912487228284,297.508385853524));
#8637=CARTESIAN_POINT('Ctrl Pts',(3.46090566195918,1.86832036841086,297.502609425349));
#8638=CARTESIAN_POINT('Ctrl Pts',(3.51530458690881,1.76755095512078,297.49683500798));
#8639=CARTESIAN_POINT('Ctrl Pts',(3.56532202691158,1.66436024449566,297.49106059061));
#8640=CARTESIAN_POINT('Ctrl Pts',(3.61074299468598,1.55917414881281,297.485286173241));
#8641=CARTESIAN_POINT('Ctrl Pts',(3.65615984121502,1.45399759712978,297.47951227981));
#8642=CARTESIAN_POINT('Ctrl Pts',(3.69698087751575,1.34682641140872,297.473738386379));
#8643=CARTESIAN_POINT('Ctrl Pts',(3.73303883802,1.23810744034365,297.467964492948));
#8644=CARTESIAN_POINT('Ctrl Pts',(3.76911983671521,1.1293190064365,297.462186910455));
#8645=CARTESIAN_POINT('Ctrl Pts',(3.80043154588862,1.01898121590954,297.456409327962));
#8646=CARTESIAN_POINT('Ctrl Pts',(3.82685634873196,0.90755687765004,297.450631745468));
#8647=CARTESIAN_POINT('Ctrl Pts',(3.85328991848953,0.796095572317501,297.444852246156));
#8648=CARTESIAN_POINT('Ctrl Pts',(3.87483327108257,0.683547418900585,297.439072746844));
#8649=CARTESIAN_POINT('Ctrl Pts',(3.8914201055522,0.570384573865847,297.433293247531));
#8650=CARTESIAN_POINT('Ctrl Pts',(3.90802739377755,0.45708218411007,297.427506621334));
#8651=CARTESIAN_POINT('Ctrl Pts',(3.91966591310782,0.343164012069071,297.421719995136));
#8652=CARTESIAN_POINT('Ctrl Pts',(3.92632133292992,0.229106504882301,297.415933368938));
#8653=CARTESIAN_POINT('Ctrl Pts',(3.93083364974762,0.151776505931063,297.41201008665));
#8654=CARTESIAN_POINT('Ctrl Pts',(3.93305646252219,0.0743825067181312,297.408086804362));
#8655=CARTESIAN_POINT('Ctrl Pts',(3.93299891020702,-0.00292785080896812,
297.404163522073));
#8656=CARTESIAN_POINT('',(-1.75029459251059,-3.52206726787383,297.));
#8657=CARTESIAN_POINT('Ctrl Pts',(3.93299891020646,-0.00292785156004575,
297.404163522035));
#8658=CARTESIAN_POINT('Ctrl Pts',(3.93285925027004,-0.190533803048494,297.394643049873));
#8659=CARTESIAN_POINT('Ctrl Pts',(3.91929411197807,-0.37765441708386,297.385122577711));
#8660=CARTESIAN_POINT('Ctrl Pts',(3.89252247461753,-0.56281238845409,297.375602105549));
#8661=CARTESIAN_POINT('Ctrl Pts',(3.87595824961153,-0.677373864770567,297.369711571439));
#8662=CARTESIAN_POINT('Ctrl Pts',(3.85430595318971,-0.791385302525627,297.363821037329));
#8663=CARTESIAN_POINT('Ctrl Pts',(3.82761280904807,-0.904361202181478,297.357930503219));
#8664=CARTESIAN_POINT('Ctrl Pts',(3.80095340004707,-1.01719432143485,297.352047413642));
#8665=CARTESIAN_POINT('Ctrl Pts',(3.76926590808212,-1.12899410958632,297.346164324065));
#8666=CARTESIAN_POINT('Ctrl Pts',(3.73264911103967,-1.23928189442707,297.340281234488));
#8667=CARTESIAN_POINT('Ctrl Pts',(3.69606897287334,-1.34945926474311,297.334404034761));
#8668=CARTESIAN_POINT('Ctrl Pts',(3.65456947581911,-1.45812725580961,297.328526835035));
#8669=CARTESIAN_POINT('Ctrl Pts',(3.60829992222045,-1.56481969290519,297.322649635308));
#8670=CARTESIAN_POINT('Ctrl Pts',(3.56123948167204,-1.67333582721792,297.31667197642));
#8671=CARTESIAN_POINT('Ctrl Pts',(3.50924450677633,-1.77980782725634,297.310694317531));
#8672=CARTESIAN_POINT('Ctrl Pts',(3.45252441188082,-1.8837633039655,297.304716658643));
#8673=CARTESIAN_POINT('Ctrl Pts',(3.39681987633037,-1.98585748343887,297.298846028267));
#8674=CARTESIAN_POINT('Ctrl Pts',(3.33655823173306,-2.0855241361153,297.29297539789));
#8675=CARTESIAN_POINT('Ctrl Pts',(3.27198511558443,-2.18233874625228,297.287104767514));
#8676=CARTESIAN_POINT('Ctrl Pts',(3.20742155668761,-2.27913902718131,297.28123500603));
#8677=CARTESIAN_POINT('Ctrl Pts',(3.13854802308323,-2.37308776380244,297.275365244546));
#8678=CARTESIAN_POINT('Ctrl Pts',(3.06565390023675,-2.46378878233569,297.269495483062));
#8679=CARTESIAN_POINT('Ctrl Pts',(2.99275322829802,-2.55449794980214,297.263625194215));
#8680=CARTESIAN_POINT('Ctrl Pts',(2.91583150616474,-2.64195849925863,297.257754905369));
#8681=CARTESIAN_POINT('Ctrl Pts',(2.83521844734992,-2.72580728515549,297.251884616523));
#8682=CARTESIAN_POINT('Ctrl Pts',(2.75202446898228,-2.81234058611954,297.245826383645));
#8683=CARTESIAN_POINT('Ctrl Pts',(2.66489913319049,-2.89502662274155,297.239768150767));
#8684=CARTESIAN_POINT('Ctrl Pts',(2.57424503439676,-2.97350828195982,297.233709917889));
#8685=CARTESIAN_POINT('Ctrl Pts',(2.48627774869555,-3.04966389577787,297.227831239379));
#8686=CARTESIAN_POINT('Ctrl Pts',(2.39498828486449,-3.12186062420929,297.22195256087));
#8687=CARTESIAN_POINT('Ctrl Pts',(2.30077631500182,-3.18981462601303,297.21607388236));
#8688=CARTESIAN_POINT('Ctrl Pts',(2.20224802540595,-3.26088193920771,297.209925872298));
#8689=CARTESIAN_POINT('Ctrl Pts',(2.10052350874328,-3.32730824867743,297.203777862236));
#8690=CARTESIAN_POINT('Ctrl Pts',(1.99609032587457,-3.38882168473792,297.197629852174));
#8691=CARTESIAN_POINT('Ctrl Pts',(1.89165714300586,-3.45033512079841,297.191481842113));
#8692=CARTESIAN_POINT('Ctrl Pts',(1.78451577278856,-3.50693550549097,297.185333832051));
#8693=CARTESIAN_POINT('Ctrl Pts',(1.67517794669337,-3.5584080495233,297.179185821989));
#8694=CARTESIAN_POINT('Ctrl Pts',(1.57185472735803,-3.60704912047498,297.17337601019));
#8695=CARTESIAN_POINT('Ctrl Pts',(1.46622640852283,-3.65127306702064,297.167566198392));
#8696=CARTESIAN_POINT('Ctrl Pts',(1.35871188831538,-3.69085234120121,297.161756386593));
#8697=CARTESIAN_POINT('Ctrl Pts',(1.25133220858134,-3.73038197661617,297.155953861231));
#8698=CARTESIAN_POINT('Ctrl Pts',(1.14207142311045,-3.76527837434843,297.15015133587));
#8699=CARTESIAN_POINT('Ctrl Pts',(1.03137166586317,-3.79536052132793,297.144348810508));
#8700=CARTESIAN_POINT('Ctrl Pts',(0.916627242200359,-3.82654178769685,297.138334276737));
#8701=CARTESIAN_POINT('Ctrl Pts',(0.80033708804374,-3.85255006284705,297.132319742966));
#8702=CARTESIAN_POINT('Ctrl Pts',(0.683015242738371,-3.87323884858487,297.126305209194));
#8703=CARTESIAN_POINT('Ctrl Pts',(0.570016091063465,-3.89316536126009,297.120512279394));
#8704=CARTESIAN_POINT('Ctrl Pts',(0.456060386669762,-3.90815736014175,297.114719349594));
#8705=CARTESIAN_POINT('Ctrl Pts',(0.341620584758718,-3.9181353187542,297.108926419794));
#8706=CARTESIAN_POINT('Ctrl Pts',(0.227217569652898,-3.92811006994045,297.103135352138));
#8707=CARTESIAN_POINT('Ctrl Pts',(0.112331187183536,-3.9330739474982,297.097344284482));
#8708=CARTESIAN_POINT('Ctrl Pts',(-0.00255992000503504,-3.93299916689663,
297.091553216826));
#8709=CARTESIAN_POINT('Ctrl Pts',(-0.117443336562963,-3.93292439130075,
297.085762536815));
#8710=CARTESIAN_POINT('Ctrl Pts',(-0.232331054333504,-3.92781162915625,
297.079971856804));
#8711=CARTESIAN_POINT('Ctrl Pts',(-0.346744203551527,-3.91768521671961,
297.074181176793));
#8712=CARTESIAN_POINT('Ctrl Pts',(-0.461178814918284,-3.9075569047236,297.068389410539));
#8713=CARTESIAN_POINT('Ctrl Pts',(-0.575138259774275,-3.89241311188772,
297.062597644286));
#8714=CARTESIAN_POINT('Ctrl Pts',(-0.688149404645904,-3.872329970042,297.056805878032));
#8715=CARTESIAN_POINT('Ctrl Pts',(-0.801268442345112,-3.8522276546275,297.051008582323));
#8716=CARTESIAN_POINT('Ctrl Pts',(-0.913436956617779,-3.82717665357635,
297.045211286614));
#8717=CARTESIAN_POINT('Ctrl Pts',(-1.02419272669782,-3.7973040777082,297.039413990906));
#8718=CARTESIAN_POINT('Ctrl Pts',(-1.1350116354853,-3.76741447233605,297.033613390324));
#8719=CARTESIAN_POINT('Ctrl Pts',(-1.24441579482542,-3.73269794898566,297.027812789742));
#8720=CARTESIAN_POINT('Ctrl Pts',(-1.35196052638055,-3.6933307102274,297.022012189161));
#8721=CARTESIAN_POINT('Ctrl Pts',(-1.45965001674123,-3.65391048184912,297.016203780776));
#8722=CARTESIAN_POINT('Ctrl Pts',(-1.56547469669027,-3.60982721005101,297.010395372392));
#8723=CARTESIAN_POINT('Ctrl Pts',(-1.6690122428726,-3.56130413376075,297.004586964008));
#8724=CARTESIAN_POINT('Ctrl Pts',(-1.6962671560051,-3.54853106468604,297.003057976006));
#8725=CARTESIAN_POINT('Ctrl Pts',(-1.72336373148895,-3.53545058421414,297.001528988003));
#8726=CARTESIAN_POINT('Ctrl Pts',(-1.75029459251059,-3.52206726787383,297.));
#8727=CARTESIAN_POINT('Ctrl Pts',(-1.75029459251059,-3.52206726787383,297.));
#8728=CARTESIAN_POINT('Ctrl Pts',(-1.77179842669062,-3.5111330638087,297.));
#8729=CARTESIAN_POINT('Ctrl Pts',(-1.79330226087066,-3.50019885974357,297.));
#8730=CARTESIAN_POINT('Ctrl Pts',(-1.8148060950507,-3.48926465567845,297.));
#8731=CARTESIAN_POINT('Origin',(0.,0.,294.689226550727));
#8732=CARTESIAN_POINT('',(-1.83773660687461,2.64742171296018,307.));
#8733=CARTESIAN_POINT('Ctrl Pts',(-1.83773660687461,2.64742171296018,307.));
#8734=CARTESIAN_POINT('Ctrl Pts',(-1.61287070412985,2.80351482766456,306.981925201061));
#8735=CARTESIAN_POINT('Ctrl Pts',(-1.36896672511014,2.93037193689488,306.963084112479));
#8736=CARTESIAN_POINT('Ctrl Pts',(-1.05017572288253,3.04755119987033,306.940809548134));
#8737=CARTESIAN_POINT('Ctrl Pts',(-0.987803804135199,3.06833536507446,306.936547798351));
#8738=CARTESIAN_POINT('Ctrl Pts',(-0.871840468484198,3.1030746666412,306.928803430231));
#8739=CARTESIAN_POINT('Ctrl Pts',(-0.818442098850674,3.11758421031641,306.925305496342));
#8740=CARTESIAN_POINT('Ctrl Pts',(-0.728882018453243,3.13945975844889,306.919548036367));
#8741=CARTESIAN_POINT('Ctrl Pts',(-0.692921543180439,3.1475921720448,306.917265149125));
#8742=CARTESIAN_POINT('Ctrl Pts',(-0.620633318897018,3.1626410950454,306.912730943104));
#8743=CARTESIAN_POINT('Ctrl Pts',(-0.584310338013351,3.16955296720124,306.910480077154));
#8744=CARTESIAN_POINT('Ctrl Pts',(-0.492739779393588,3.18535013274941,306.9048694953));
#8745=CARTESIAN_POINT('Ctrl Pts',(-0.437363761211979,3.19342471899757,306.901534730072));
#8746=CARTESIAN_POINT('Ctrl Pts',(-0.164547752393253,3.22597479512708,306.885344468204));
#8747=CARTESIAN_POINT('Ctrl Pts',(0.0547837142037089,3.22970538388019,306.873117270049));
#8748=CARTESIAN_POINT('Ctrl Pts',(0.380689913146888,3.20201715200492,306.854682802465));
#8749=CARTESIAN_POINT('Ctrl Pts',(0.488029488352053,3.1874226923407,306.848557386198));
#8750=CARTESIAN_POINT('Ctrl Pts',(0.638836058752621,3.15912137709952,306.839643332122));
#8751=CARTESIAN_POINT('Ctrl Pts',(0.683065213441602,3.14985411486993,306.836990481927));
#8752=CARTESIAN_POINT('Ctrl Pts',(0.761855729305654,3.13160779863767,306.832172485715));
#8753=CARTESIAN_POINT('Ctrl Pts',(0.796490807200217,3.12297834146815,306.830022269894));
#8754=CARTESIAN_POINT('Ctrl Pts',(0.851768223127815,3.10822644914928,306.826528210933));
#8755=CARTESIAN_POINT('Ctrl Pts',(0.872505836561738,3.10246906040753,306.825203193745));
#8756=CARTESIAN_POINT('Ctrl Pts',(0.91403557023949,3.09048985150914,306.82251821819));
#8757=CARTESIAN_POINT('Ctrl Pts',(0.934825550593697,3.08426485055132,306.821158100424));
#8758=CARTESIAN_POINT('Ctrl Pts',(0.990984156166277,3.06682972145306,306.817443537762));
#8759=CARTESIAN_POINT('Ctrl Pts',(1.02622371080723,3.05521828511104,306.815068765204));
#8760=CARTESIAN_POINT('Ctrl Pts',(1.23466757292442,2.98252305104199,306.800790453124));
#8761=CARTESIAN_POINT('Ctrl Pts',(1.40258282254529,2.90733561485834,306.788350032493));
#8762=CARTESIAN_POINT('Ctrl Pts',(1.73915739230668,2.72065238146191,306.762428562735));
#8763=CARTESIAN_POINT('Ctrl Pts',(1.90563882353315,2.60675666300069,306.749030436459));
#8764=CARTESIAN_POINT('Ctrl Pts',(2.10080242353114,2.44448445893484,306.732834129059));
#8765=CARTESIAN_POINT('Ctrl Pts',(2.14035554269547,2.40992816212038,306.729520558536));
#8766=CARTESIAN_POINT('Ctrl Pts',(2.20580482506759,2.34986414217837,306.723980701444));
#8767=CARTESIAN_POINT('Ctrl Pts',(2.23214511916507,2.32485800576727,306.721734693006));
#8768=CARTESIAN_POINT('Ctrl Pts',(2.28162669112034,2.27626632300347,306.717481060624));
#8769=CARTESIAN_POINT('Ctrl Pts',(2.30483879201089,2.2527598619761,306.715470504151));
#8770=CARTESIAN_POINT('Ctrl Pts',(2.36549664247051,2.18941362276678,306.710172082117));
#8771=CARTESIAN_POINT('Ctrl Pts',(2.40229783085265,2.14896998990693,306.706911093949));
#8772=CARTESIAN_POINT('Ctrl Pts',(2.59380992471914,1.92743124043834,306.689640868596));
#8773=CARTESIAN_POINT('Ctrl Pts',(2.72911359781551,1.73054601380094,306.676412443957));
#8774=CARTESIAN_POINT('Ctrl Pts',(2.88999641078797,1.42989734306044,306.65721659348));
#8775=CARTESIAN_POINT('Ctrl Pts',(2.93413220223388,1.33699348973775,306.651396244909));
#8776=CARTESIAN_POINT('Ctrl Pts',(2.99067309033731,1.20163210406146,306.642870217234));
#8777=CARTESIAN_POINT('Ctrl Pts',(3.00676516545293,1.16077911378317,306.640291048985));
#8778=CARTESIAN_POINT('Ctrl Pts',(3.03414481857618,1.0868769260064,306.635593691662));
#8779=CARTESIAN_POINT('Ctrl Pts',(3.04573944202751,1.05394841661457,306.633489605921));
#8780=CARTESIAN_POINT('Ctrl Pts',(3.06351637601019,1.00071726389996,306.630060821614));
#8781=CARTESIAN_POINT('Ctrl Pts',(3.07003729912584,0.98052973061205,306.628754220295));
#8782=CARTESIAN_POINT('Ctrl Pts',(3.08276120522064,0.939767353358554,306.626100664425));
#8783=CARTESIAN_POINT('Ctrl Pts',(3.08895863951121,0.919191921180365,306.624753465552));
#8784=CARTESIAN_POINT('Ctrl Pts',(3.10519172891196,0.863279377217664,306.621074413987));
#8785=CARTESIAN_POINT('Ctrl Pts',(3.11482942403955,0.827831116045951,306.618722444911));
#8786=CARTESIAN_POINT('Ctrl Pts',(3.17032298187014,0.609012655509117,306.60411652629));
#8787=CARTESIAN_POINT('Ctrl Pts',(3.20057583201716,0.422077655409949,306.591287083847));
#8788=CARTESIAN_POINT('Ctrl Pts',(3.22389613507508,0.101173973082913,306.569606783471));
#8789=CARTESIAN_POINT('Ctrl Pts',(3.22532816999698,-0.0317127598530274,
306.560722540597));
#8790=CARTESIAN_POINT('Ctrl Pts',(3.21538154062596,-0.226541299232325,306.547960786327));
#8791=CARTESIAN_POINT('Ctrl Pts',(3.21040093963496,-0.288662434806583,306.543929938373));
#8792=CARTESIAN_POINT('Ctrl Pts',(3.19785373624608,-0.403311926627462,306.536564443814));
#8793=CARTESIAN_POINT('Ctrl Pts',(3.19078516043562,-0.455872363121254,306.533216631283));
#8794=CARTESIAN_POINT('Ctrl Pts',(3.1767224450102,-0.543928727000493,306.527653573156));
#8795=CARTESIAN_POINT('Ctrl Pts',(3.17042222253808,-0.579523122859388,306.525417464515));
#8796=CARTESIAN_POINT('Ctrl Pts',(3.15649363764549,-0.65117035338417,306.520939473213));
#8797=CARTESIAN_POINT('Ctrl Pts',(3.14884309553138,-0.687213390501681,306.518698648962));
#8798=CARTESIAN_POINT('Ctrl Pts',(3.1278179843444,-0.778527551955302,306.513047107254));
#8799=CARTESIAN_POINT('Ctrl Pts',(3.11359538902554,-0.833591517412508,306.509663286526));
#8800=CARTESIAN_POINT('Ctrl Pts',(3.03787008771021,-1.09769549607522,306.493504476644));
#8801=CARTESIAN_POINT('Ctrl Pts',(2.95673330280883,-1.30051054264951,306.481360031334));
#8802=CARTESIAN_POINT('Ctrl Pts',(2.7789395820027,-1.64045011348556,306.459829428575));
#8803=CARTESIAN_POINT('Ctrl Pts',(2.69092958273882,-1.78114222663982,306.450494482124));
#8804=CARTESIAN_POINT('Ctrl Pts',(2.57258227108704,-1.94140745585752,306.43860712754));
#8805=CARTESIAN_POINT('Ctrl Pts',(2.55223961579672,-1.96807398148679,306.43658376302));
#8806=CARTESIAN_POINT('Ctrl Pts',(2.51860192680313,-2.0107698268558,306.433260970514));
#8807=CARTESIAN_POINT('Ctrl Pts',(2.50556052904555,-2.026997131263,306.431978046634));
#8808=CARTESIAN_POINT('Ctrl Pts',(2.47854663321916,-2.0599512410396,306.429328855182));
#8809=CARTESIAN_POINT('Ctrl Pts',(2.46456011484081,-2.07666461090596,306.427961788277));
#8810=CARTESIAN_POINT('Ctrl Pts',(2.42571484417746,-2.12213810179588,306.424180373945));
#8811=CARTESIAN_POINT('Ctrl Pts',(2.40051576363387,-2.1506014074319,306.421744235517));
#8812=CARTESIAN_POINT('Ctrl Pts',(2.26342559396227,-2.30003815802544,306.408609366423));
#8813=CARTESIAN_POINT('Ctrl Pts',(2.14288977364294,-2.41273426330881,306.397482752757));
#8814=CARTESIAN_POINT('Ctrl Pts',(1.89959055234895,-2.60753877182522,306.376464665738));
#8815=CARTESIAN_POINT('Ctrl Pts',(1.77875099969262,-2.69142224501287,306.366593040309));
#8816=CARTESIAN_POINT('Ctrl Pts',(1.59613125004096,-2.80050159449724,306.352642675542));
#8817=CARTESIAN_POINT('Ctrl Pts',(1.53863893246068,-2.83249629952332,306.348377331761));
#8818=CARTESIAN_POINT('Ctrl Pts',(1.43113267567081,-2.88808391054059,306.340634354899));
#8819=CARTESIAN_POINT('Ctrl Pts',(1.38141437204418,-2.91219235790896,306.337141198978));
#8820=CARTESIAN_POINT('Ctrl Pts',(1.29768657491515,-2.95016492355461,306.33139954886));
#8821=CARTESIAN_POINT('Ctrl Pts',(1.26401748154344,-2.96474678555149,306.329127536149));
#8822=CARTESIAN_POINT('Ctrl Pts',(1.19620664627505,-2.99274996149709,306.32462220454));
#8823=CARTESIAN_POINT('Ctrl Pts',(1.16207017945549,-3.00616961239103,306.322389208966));
#8824=CARTESIAN_POINT('Ctrl Pts',(1.07601618947093,-3.03831399744688,306.316842589215));
#8825=CARTESIAN_POINT('Ctrl Pts',(1.02383193274198,-3.05629374959402,306.313553256359));
#8826=CARTESIAN_POINT('Ctrl Pts',(0.720205987844388,-3.15225584394364,306.29478903629));
#8827=CARTESIAN_POINT('Ctrl Pts',(0.460437782574308,-3.20053370881745,306.280298475396));
#8828=CARTESIAN_POINT('Ctrl Pts',(0.112490426482024,-3.22191689234664,306.260584485301));
#8829=CARTESIAN_POINT('Ctrl Pts',(0.0271290448312729,-3.22376565431938,
306.255714483836));
#8830=CARTESIAN_POINT('Ctrl Pts',(-0.113940200882418,-3.22121765483144,
306.247474244329));
#8831=CARTESIAN_POINT('Ctrl Pts',(-0.169641527447385,-3.21876475248769,
306.24417080106));
#8832=CARTESIAN_POINT('Ctrl Pts',(-0.250279827510826,-3.21311488396034,
306.23928090679));
#8833=CARTESIAN_POINT('Ctrl Pts',(-0.275289797258755,-3.21106877645816,
306.237749244342));
#8834=CARTESIAN_POINT('Ctrl Pts',(-0.32011990641438,-3.20687358346846,306.234972670186));
#8835=CARTESIAN_POINT('Ctrl Pts',(-0.339948087770548,-3.20483231558631,
306.233733381659));
#8836=CARTESIAN_POINT('Ctrl Pts',(-0.385993150355525,-3.19965996883413,
306.230829534818));
#8837=CARTESIAN_POINT('Ctrl Pts',(-0.412191956711931,-3.1963905134471,306.229158052042));
#8838=CARTESIAN_POINT('Ctrl Pts',(-0.497754600274649,-3.18464342612453,
306.223642456298));
#8839=CARTESIAN_POINT('Ctrl Pts',(-0.556919617412703,-3.17483117603528,
306.219739095561));
#8840=CARTESIAN_POINT('Ctrl Pts',(-0.814290122059809,-3.12473226156958,
306.202460057997));
#8841=CARTESIAN_POINT('Ctrl Pts',(-1.00872586434939,-3.06748952045082,306.188656788649));
#8842=CARTESIAN_POINT('Ctrl Pts',(-1.2911322661333,-2.95456919024241,306.168317470085));
#8843=CARTESIAN_POINT('Ctrl Pts',(-1.3839091307744,-2.91226714546435,306.161577908947));
#8844=CARTESIAN_POINT('Ctrl Pts',(-1.47484249366466,-2.86547680213046,306.154940145955));
#8845=CARTESIAN_POINT('Ctrl Pts',(-1.47515326121876,-2.86531683075061,306.154917460778));
#8846=CARTESIAN_POINT('Ctrl Pts',(-1.47546400238914,-2.86515680899909,306.154894777109));
#8847=CARTESIAN_POINT('',(1.87158653173908,2.62360084935054,307.));
#8848=CARTESIAN_POINT('Origin',(0.,0.,307.));
#8849=CARTESIAN_POINT('',(3.22274974449961,-0.00128328785181631,306.810773449319));
#8850=CARTESIAN_POINT('Ctrl Pts',(3.22274974449961,-0.00128328785181409,
306.810773449319));
#8851=CARTESIAN_POINT('Ctrl Pts',(3.2227900185038,0.0998577278200301,306.817062136975));
#8852=CARTESIAN_POINT('Ctrl Pts',(3.21806481467562,0.201159732219282,306.823350824632));
#8853=CARTESIAN_POINT('Ctrl Pts',(3.20855495035338,0.302146807136616,306.829639512289));
#8854=CARTESIAN_POINT('Ctrl Pts',(3.19905935199351,0.402982389060622,306.835918766144));
#8855=CARTESIAN_POINT('Ctrl Pts',(3.1847934102067,0.503503571635619,306.842198019998));
#8856=CARTESIAN_POINT('Ctrl Pts',(3.16578993983136,0.603234298894355,306.848477273852));
#8857=CARTESIAN_POINT('Ctrl Pts',(3.1466829878995,0.703508100164581,306.854790720775));
#8858=CARTESIAN_POINT('Ctrl Pts',(3.12278673719962,0.802982385591739,306.861104167698));
#8859=CARTESIAN_POINT('Ctrl Pts',(3.09418761530848,0.901177320937233,306.867417614621));
#8860=CARTESIAN_POINT('Ctrl Pts',(3.06581086092608,0.998608758605197,306.873681972433));
#8861=CARTESIAN_POINT('Ctrl Pts',(3.03280421803192,1.09478026340372,306.879946330245));
#8862=CARTESIAN_POINT('Ctrl Pts',(2.9953032935351,1.18923325812803,306.886210688057));
#8863=CARTESIAN_POINT('Ctrl Pts',(2.95782620525254,1.28362621695055,306.892471064138));
#8864=CARTESIAN_POINT('Ctrl Pts',(2.91586067103949,1.37630245420618,306.89873144022));
#8865=CARTESIAN_POINT('Ctrl Pts',(2.86959151116524,1.46682041216653,306.904991816301));
#8866=CARTESIAN_POINT('Ctrl Pts',(2.82334098226624,1.55730192170554,306.911249671548));
#8867=CARTESIAN_POINT('Ctrl Pts',(2.77279046509754,1.64562651266173,306.917507526795));
#8868=CARTESIAN_POINT('Ctrl Pts',(2.71817178259418,1.73137509593062,306.923765382041));
#8869=CARTESIAN_POINT('Ctrl Pts',(2.66272368003668,1.81842582695039,306.930118266871));
#8870=CARTESIAN_POINT('Ctrl Pts',(2.60308303061169,1.90282127450765,306.936471151701));
#8871=CARTESIAN_POINT('Ctrl Pts',(2.53953908698161,1.98415190653151,306.942824036531));
#8872=CARTESIAN_POINT('Ctrl Pts',(2.47693440670235,2.06428036447558,306.949083017339));
#8873=CARTESIAN_POINT('Ctrl Pts',(2.41054134049455,2.14143369306294,306.955341998146));
#8874=CARTESIAN_POINT('Ctrl Pts',(2.34067753745869,2.21525308444347,306.961600978954));
#8875=CARTESIAN_POINT('Ctrl Pts',(2.26924147554104,2.2907337537491,306.968000815795));
#8876=CARTESIAN_POINT('Ctrl Pts',(2.19417688390513,2.36272828260635,306.974400652636));
#8877=CARTESIAN_POINT('Ctrl Pts',(2.11586276660478,2.43089331633364,306.980800489477));
#8878=CARTESIAN_POINT('Ctrl Pts',(2.03754864930444,2.49905835006092,306.987200326318));
#8879=CARTESIAN_POINT('Ctrl Pts',(1.95598538003388,2.56339361630214,306.993600163159));
#8880=CARTESIAN_POINT('Ctrl Pts',(1.87158653173908,2.62360084935054,307.));
#8881=CARTESIAN_POINT('Ctrl Pts',(-1.47546400239267,-2.86515680899727,306.403639991207));
#8882=CARTESIAN_POINT('Ctrl Pts',(-1.44148025683963,-2.88265734965617,306.406010377244));
#8883=CARTESIAN_POINT('Ctrl Pts',(-1.4072048219913,-2.89954303224035,306.408380763282));
#8884=CARTESIAN_POINT('Ctrl Pts',(-1.37266201798484,-2.91580461397567,306.410751149319));
#8885=CARTESIAN_POINT('Ctrl Pts',(-1.28260809080463,-2.95819895165459,306.416930803164));
#8886=CARTESIAN_POINT('Ctrl Pts',(-1.19043722760257,-2.99648857823904,306.42311045701));
#8887=CARTESIAN_POINT('Ctrl Pts',(-1.09655907514793,-3.03045801112814,306.429290110855));
#8888=CARTESIAN_POINT('Ctrl Pts',(-1.00280319052376,-3.06438320189324,306.435461716258));
#8889=CARTESIAN_POINT('Ctrl Pts',(-0.907344840639183,-3.09399923764599,
306.441633321662));
#8890=CARTESIAN_POINT('Ctrl Pts',(-0.810616121734273,-3.11913755158128,
306.447804927065));
#8891=CARTESIAN_POINT('Ctrl Pts',(-0.713985031579461,-3.14425049329831,
306.453970303438));
#8892=CARTESIAN_POINT('Ctrl Pts',(-0.616086538789796,-3.16489459080302,
306.460135679811));
#8893=CARTESIAN_POINT('Ctrl Pts',(-0.517369577501691,-3.18095053133112,
306.466301056184));
#8894=CARTESIAN_POINT('Ctrl Pts',(-0.41871866805352,-3.19699572877718,306.472462307283));
#8895=CARTESIAN_POINT('Ctrl Pts',(-0.31925080513799,-3.20845880339074,306.478623558383));
#8896=CARTESIAN_POINT('Ctrl Pts',(-0.219425976298026,-3.21527134211495,
306.484784809483));
#8897=CARTESIAN_POINT('Ctrl Pts',(-0.119634950830539,-3.22208157393028,
306.490943974217));
#8898=CARTESIAN_POINT('Ctrl Pts',(-0.0194876312642712,-3.22424436990655,
306.497103138951));
#8899=CARTESIAN_POINT('Ctrl Pts',(0.0805508922861619,-3.22174317974787,
306.503262303685));
#8900=CARTESIAN_POINT('Ctrl Pts',(0.180582091152676,-3.21924217272291,306.509421017454));
#8901=CARTESIAN_POINT('Ctrl Pts',(0.280504076959468,-3.21207786961416,306.515579731223));
#8902=CARTESIAN_POINT('Ctrl Pts',(0.379852771505078,-3.20028583637148,306.521738444991));
#8903=CARTESIAN_POINT('Ctrl Pts',(0.479220559436792,-3.1884915368701,306.527898342376));
#8904=CARTESIAN_POINT('Ctrl Pts',(0.5780144072396,-3.17206779140419,306.53405823976));
#8905=CARTESIAN_POINT('Ctrl Pts',(0.675777349248666,-3.1511017972675,306.540218137145));
#8906=CARTESIAN_POINT('Ctrl Pts',(0.773645906311291,-3.13011315319261,306.546384689177));
#8907=CARTESIAN_POINT('Ctrl Pts',(0.870480909905088,-3.10457255410761,306.552551241208));
#8908=CARTESIAN_POINT('Ctrl Pts',(0.965837679616123,-3.07461788506047,306.55871779324));
#8909=CARTESIAN_POINT('Ctrl Pts',(1.06125042793634,-3.04464563130785,306.564887965309));
#8910=CARTESIAN_POINT('Ctrl Pts',(1.1551828078156,-3.01025429615689,306.571058137377));
#8911=CARTESIAN_POINT('Ctrl Pts',(1.24720927533731,-2.97163029093671,306.577228309446));
#8912=CARTESIAN_POINT('Ctrl Pts',(1.3393842130672,-2.93294397196864,306.583408436115));
#8913=CARTESIAN_POINT('Ctrl Pts',(1.42964670704646,-2.89001153183243,306.589588562784));
#8914=CARTESIAN_POINT('Ctrl Pts',(1.51759496417796,-2.84306579016415,306.595768689453));
#8915=CARTESIAN_POINT('Ctrl Pts',(1.57166611144707,-2.81420324991383,306.599568270595));
#8916=CARTESIAN_POINT('Ctrl Pts',(1.62486303875039,-2.78382461569644,306.603367851737));
#8917=CARTESIAN_POINT('Ctrl Pts',(1.67709810690495,-2.75199191537981,306.607167432879));
#8918=CARTESIAN_POINT('Ctrl Pts',(1.76153937550061,-2.7005323558822,306.61330969445));
#8919=CARTESIAN_POINT('Ctrl Pts',(1.84376394271427,-2.64508882172917,306.61945195602));
#8920=CARTESIAN_POINT('Ctrl Pts',(1.92336899553465,-2.58587881957296,306.625594217591));
#8921=CARTESIAN_POINT('Ctrl Pts',(2.00286782485598,-2.52674782614025,306.631728283042));
#8922=CARTESIAN_POINT('Ctrl Pts',(2.0797537364873,-2.46386061159534,306.637862348493));
#8923=CARTESIAN_POINT('Ctrl Pts',(2.15365030406937,-2.39747949527872,306.643996413945));
#8924=CARTESIAN_POINT('Ctrl Pts',(2.22747066260521,-2.33116683737266,306.650124153374));
#8925=CARTESIAN_POINT('Ctrl Pts',(2.29830747988894,-2.26136773151431,306.656251892804));
#8926=CARTESIAN_POINT('Ctrl Pts',(2.36581585552691,-2.1883859120908,306.662379632234));
#8927=CARTESIAN_POINT('Ctrl Pts',(2.43327891022544,-2.11545308813765,306.668503257879));
#8928=CARTESIAN_POINT('Ctrl Pts',(2.49741766648453,-2.03934211823852,306.674626883524));
#8929=CARTESIAN_POINT('Ctrl Pts',(2.55792339060626,-1.96039421808201,306.680750509169));
#8930=CARTESIAN_POINT('Ctrl Pts',(2.61840867311654,-1.8814729901507,306.686872065973));
#8931=CARTESIAN_POINT('Ctrl Pts',(2.675263094699,-1.79971708409036,306.692993622776));
#8932=CARTESIAN_POINT('Ctrl Pts',(2.72821825743358,-1.71550071474951,306.69911517958));
#8933=CARTESIAN_POINT('Ctrl Pts',(2.781170055598,-1.6312896961973,306.705236347442));
#8934=CARTESIAN_POINT('Ctrl Pts',(2.83022285364238,-1.54461889699493,306.711357515305));
#8935=CARTESIAN_POINT('Ctrl Pts',(2.87515223598542,-1.45589051182018,306.717478683168));
#8936=CARTESIAN_POINT('Ctrl Pts',(2.92009108854134,-1.36714342448101,306.72360114125));
#8937=CARTESIAN_POINT('Ctrl Pts',(2.96090460081192,-1.2763382816299,306.729723599333));
#8938=CARTESIAN_POINT('Ctrl Pts',(2.99741534562876,-1.18389983034429,306.735846057415));
#8939=CARTESIAN_POINT('Ctrl Pts',(3.03396812778423,-1.09135494829429,306.741975564705));
#8940=CARTESIAN_POINT('Ctrl Pts',(3.06620809057851,-0.997173412699476,306.748105071996));
#8941=CARTESIAN_POINT('Ctrl Pts',(3.09400687590812,-0.901797657090131,306.754234579286));
#8942=CARTESIAN_POINT('Ctrl Pts',(3.12182281687966,-0.806363041631609,306.760367869319));
#8943=CARTESIAN_POINT('Ctrl Pts',(3.14519202204811,-0.709733165797646,306.766501159351));
#8944=CARTESIAN_POINT('Ctrl Pts',(3.16403720627626,-0.612361102454695,306.772634449384));
#8945=CARTESIAN_POINT('Ctrl Pts',(3.18291493122178,-0.514820902957957,306.778778330008));
#8946=CARTESIAN_POINT('Ctrl Pts',(3.197252973546,-0.416536391159208,306.784922210633));
#8947=CARTESIAN_POINT('Ctrl Pts',(3.20702588338914,-0.317966265147866,306.791066091258));
#8948=CARTESIAN_POINT('Ctrl Pts',(3.21366303612879,-0.2510235641096,306.795238632985));
#8949=CARTESIAN_POINT('Ctrl Pts',(3.21819571122489,-0.183949193495648,306.799411174712));
#8950=CARTESIAN_POINT('Ctrl Pts',(3.2206296272874,-0.116886125517962,306.80358371644));
#8951=CARTESIAN_POINT('Ctrl Pts',(3.22202759263413,-0.0783671944331345,
306.805980294051));
#8952=CARTESIAN_POINT('Ctrl Pts',(3.22273439633175,-0.0398274661541265,
306.808376871662));
#8953=CARTESIAN_POINT('Ctrl Pts',(3.22274974449932,-0.00128328858516614,
306.810773449273));
#8954=CARTESIAN_POINT('Ctrl Pts',(1.43037091239959,-2.88157788358434,296.586649784659));
#8955=CARTESIAN_POINT('Ctrl Pts',(2.37869428028674,-2.41084475896467,296.652121879179));
#8956=CARTESIAN_POINT('Ctrl Pts',(3.75821890350017,-0.46632426907627,296.783066068219));
#8957=CARTESIAN_POINT('Ctrl Pts',(2.46052379546342,2.88456422682259,296.97948235178));
#8958=CARTESIAN_POINT('Ctrl Pts',(-1.05164585738147,3.64025694602008,297.17589863534));
#8959=CARTESIAN_POINT('Ctrl Pts',(-3.61728260103292,1.12907581019222,297.3723149189));
#8960=CARTESIAN_POINT('Ctrl Pts',(-2.93521143642197,-2.39722873440577,297.56873120246));
#8961=CARTESIAN_POINT('Ctrl Pts',(0.383440535871874,-3.77005108800603,297.765147486021));
#8962=CARTESIAN_POINT('Ctrl Pts',(3.35750728960981,-1.75722429176289,297.96156376958));
#8963=CARTESIAN_POINT('Ctrl Pts',(3.3162883264954,1.8338860675821,298.157980053141));
#8964=CARTESIAN_POINT('Ctrl Pts',(0.296653368432913,3.77792383424779,298.354396336701));
#8965=CARTESIAN_POINT('Ctrl Pts',(-2.98938444913632,2.32902251834708,298.550812620261));
#8966=CARTESIAN_POINT('Ctrl Pts',(-3.59065782085272,-1.21159272548526,298.747228903822));
#8967=CARTESIAN_POINT('Ctrl Pts',(-0.96714588876518,-3.66406736193667,298.943645187382));
#8968=CARTESIAN_POINT('Ctrl Pts',(2.5249602887996,-2.82583495365449,299.140061470942));
#8969=CARTESIAN_POINT('Ctrl Pts',(3.74939329087914,0.550289383578493,299.336477754502));
#8970=CARTESIAN_POINT('Ctrl Pts',(1.6064846293266,3.43219662332693,299.532894038062));
#8971=CARTESIAN_POINT('Ctrl Pts',(-1.97921236533452,3.23163824688042,299.729310321623));
#8972=CARTESIAN_POINT('Ctrl Pts',(-3.78737302228878,0.128735920266949,299.925726605183));
#8973=CARTESIAN_POINT('Ctrl Pts',(-2.19408276686631,-3.08978445485654,300.122142888743));
#8974=CARTESIAN_POINT('Ctrl Pts',(1.36971965459014,-3.53336034491094,300.318559172303));
#8975=CARTESIAN_POINT('Ctrl Pts',(3.70337283434201,-0.803614895688885,300.514975455864));
#8976=CARTESIAN_POINT('Ctrl Pts',(2.71101596545655,2.64785945046433,300.711391739424));
#8977=CARTESIAN_POINT('Ctrl Pts',(-0.716112319080844,3.72128343332825,300.907808022984));
#8978=CARTESIAN_POINT('Ctrl Pts',(-3.50009802324731,1.45261181002151,301.104224306544));
#8979=CARTESIAN_POINT('Ctrl Pts',(-3.14063538989392,-2.12065475486385,301.300640590105));
#8980=CARTESIAN_POINT('Ctrl Pts',(0.0394411310795686,-3.78935504273392,
301.497056873665));
#8981=CARTESIAN_POINT('Ctrl Pts',(3.18409545625435,-2.05482441288724,301.693473157225));
#8982=CARTESIAN_POINT('Ctrl Pts',(3.46910427998845,1.5251500702891,301.889889440785));
#8983=CARTESIAN_POINT('Ctrl Pts',(0.638500338801349,3.73538278628368,302.086305724345));
#8984=CARTESIAN_POINT('Ctrl Pts',(-2.76554263595121,2.5908572269264,302.282722007906));
#8985=CARTESIAN_POINT('Ctrl Pts',(-3.68584362940364,-0.880524833572776,
302.479138291466));
#8986=CARTESIAN_POINT('Ctrl Pts',(-1.29587760982979,-3.56110495001826,302.675554575026));
#8987=CARTESIAN_POINT('Ctrl Pts',(2.25791990446593,-3.04344622745171,302.871970858586));
#8988=CARTESIAN_POINT('Ctrl Pts',(3.78387290864046,0.207540506822766,303.068387142146));
#8989=CARTESIAN_POINT('Ctrl Pts',(1.91151851156535,3.2721345081006,303.264803425707));
#8990=CARTESIAN_POINT('Ctrl Pts',(-1.67757627766529,3.39801486134882,303.461219709267));
#8991=CARTESIAN_POINT('Ctrl Pts',(-3.76003489430519,0.472128097803197,303.657635992827));
#8992=CARTESIAN_POINT('Ctrl Pts',(-2.46559506200593,-2.87777836811756,303.854052276388));
#8993=CARTESIAN_POINT('Ctrl Pts',(1.04320286127918,-3.643143466247,304.050468559947));
#8994=CARTESIAN_POINT('Ctrl Pts',(3.61509741898655,-1.13659100234235,304.246884843508));
#8995=CARTESIAN_POINT('Ctrl Pts',(2.94026192950194,2.39073784243107,304.443301127068));
#8996=CARTESIAN_POINT('Ctrl Pts',(-0.375230571251665,3.77093659736716,304.639717410628));
#8997=CARTESIAN_POINT('Ctrl Pts',(-3.35372926879606,1.7644490671369,304.836133694189));
#8998=CARTESIAN_POINT('Ctrl Pts',(-3.32022984313726,-1.82670169005412,305.032549977749));
#8999=CARTESIAN_POINT('Ctrl Pts',(-0.304830726285696,-3.77727281867384,
305.228966261309));
#9000=CARTESIAN_POINT('Ctrl Pts',(2.98435586070458,-2.33549276813259,305.425382544869));
#9001=CARTESIAN_POINT('Ctrl Pts',(3.59324514050816,1.20386119281218,305.621798828429));
#9002=CARTESIAN_POINT('Ctrl Pts',(0.975112331956289,3.66189401687049,305.81821511199));
#9003=CARTESIAN_POINT('Ctrl Pts',(-2.51894641698954,2.83144498973554,306.01463139555));
#9004=CARTESIAN_POINT('Ctrl Pts',(-3.75036188556599,-0.542523113047413,
306.21104767911));
#9005=CARTESIAN_POINT('Ctrl Pts',(-1.61436456647499,-3.42801060221597,306.40746396267));
#9006=CARTESIAN_POINT('Ctrl Pts',(1.97313131176253,-3.23753624740303,306.60388024623));
#9007=CARTESIAN_POINT('Ctrl Pts',(3.78506371541952,-0.133490475520108,306.800340127458));
#9008=CARTESIAN_POINT('Ctrl Pts',(2.72947568708186,2.00554125229389,306.931327914165));
#9009=CARTESIAN_POINT('Ctrl Pts',(1.8665577825944,2.62019345361895,306.996843606352));
#9010=CARTESIAN_POINT('Ctrl Pts',(1.53690913862227,-3.0962062668787,296.724992037258));
#9011=CARTESIAN_POINT('Ctrl Pts',(2.55586641595513,-2.5904115567035,296.790464131778));
#9012=CARTESIAN_POINT('Ctrl Pts',(4.03814208444891,-0.501057470123149,296.921408320818));
#9013=CARTESIAN_POINT('Ctrl Pts',(2.64379083373645,3.09941504173152,297.117824604378));
#9014=CARTESIAN_POINT('Ctrl Pts',(-1.12997552927888,3.91139397394884,297.314240887938));
#9015=CARTESIAN_POINT('Ctrl Pts',(-3.88670843227672,1.21317269236876,297.510657171498));
#9016=CARTESIAN_POINT('Ctrl Pts',(-3.15383460424095,-2.57578137064835,297.707073455059));
#9017=CARTESIAN_POINT('Ctrl Pts',(0.412000313059402,-4.05085556480515,297.903489738619));
#9018=CARTESIAN_POINT('Ctrl Pts',(3.60758429275907,-1.88810751757302,298.099906022179));
#9019=CARTESIAN_POINT('Ctrl Pts',(3.56329522022138,1.97047928759305,298.29632230574));
#9020=CARTESIAN_POINT('Ctrl Pts',(0.318748982515844,4.05931469630743,298.4927385893));
#9021=CARTESIAN_POINT('Ctrl Pts',(-3.21204258203581,2.50249495531178,298.68915487286));
#9022=CARTESIAN_POINT('Ctrl Pts',(-3.85810056027791,-1.30183570984583,298.88557115642));
#9023=CARTESIAN_POINT('Ctrl Pts',(-1.03918175484326,-3.93697785956856,299.08198743998));
#9024=CARTESIAN_POINT('Ctrl Pts',(2.71302674633131,-3.03631143982363,299.278403723541));
#9025=CARTESIAN_POINT('Ctrl Pts',(4.0286591142811,0.591276552939527,299.474820007101));
#9026=CARTESIAN_POINT('Ctrl Pts',(1.72614032239109,3.68783670739665,299.671236290661));
#9027=CARTESIAN_POINT('Ctrl Pts',(-2.12662991479166,3.47234015407905,299.867652574221));
#9028=CARTESIAN_POINT('Ctrl Pts',(-4.06946768762379,0.138324549675935,300.064068857781));
#9029=CARTESIAN_POINT('Ctrl Pts',(-2.35750449485402,-3.31992067503358,300.260485141342));
#9030=CARTESIAN_POINT('Ctrl Pts',(1.47174039701251,-3.7965354000586,300.456901424902));
#9031=CARTESIAN_POINT('Ctrl Pts',(3.97921091898969,-0.863470493150105,300.653317708462));
#9032=CARTESIAN_POINT('Ctrl Pts',(2.912940396188,2.84507979848314,300.849733992022));
#9033=CARTESIAN_POINT('Ctrl Pts',(-0.769450467661539,3.99845555198771,301.046150275583));
#9034=CARTESIAN_POINT('Ctrl Pts',(-3.76079560299375,1.56080660361544,301.242566559143));
#9035=CARTESIAN_POINT('Ctrl Pts',(-3.37455913704994,-2.27860734887659,301.438982842703));
#9036=CARTESIAN_POINT('Ctrl Pts',(0.0423788223518119,-4.07159733477241,
301.635399126263));
#9037=CARTESIAN_POINT('Ctrl Pts',(3.421256236785,-2.20787376970116,301.831815409824));
#9038=CARTESIAN_POINT('Ctrl Pts',(3.72749335471555,1.63874772653576,302.028231693384));
#9039=CARTESIAN_POINT('Ctrl Pts',(0.68605771916248,4.01360506615777,302.224647976944));
#9040=CARTESIAN_POINT('Ctrl Pts',(-2.97152837323328,2.78383188193381,302.421064260504));
#9041=CARTESIAN_POINT('Ctrl Pts',(-3.9603760873883,-0.946108909074201,302.617480544064));
#9042=CARTESIAN_POINT('Ctrl Pts',(-1.39239837990148,-3.82634650483378,302.813896827625));
#9043=CARTESIAN_POINT('Ctrl Pts',(2.4260964099369,-3.27013104036704,303.010313111185));
#9044=CARTESIAN_POINT('Ctrl Pts',(4.06570687523191,0.222998733269188,303.206729394745));
#9045=CARTESIAN_POINT('Ctrl Pts',(2.05389402399265,3.51585269576301,303.403145678305));
#9046=CARTESIAN_POINT('Ctrl Pts',(-1.8025270854777,3.65110898740253,303.599561961865));
#9047=CARTESIAN_POINT('Ctrl Pts',(-4.04009333558223,0.507293585058156,303.795978245426));
#9048=CARTESIAN_POINT('Ctrl Pts',(-2.64923982310418,-3.09212375234166,303.992394528986));
#9049=CARTESIAN_POINT('Ctrl Pts',(1.12090367403175,-3.9144954906793,304.188810812546));
#9050=CARTESIAN_POINT('Ctrl Pts',(3.88436049145415,-1.2212476381006,304.385227096106));
#9051=CARTESIAN_POINT('Ctrl Pts',(3.15926127287765,2.56880701797711,304.581643379667));
#9052=CARTESIAN_POINT('Ctrl Pts',(-0.403178846163521,4.05180702950403,304.778059663227));
#9053=CARTESIAN_POINT('Ctrl Pts',(-3.60352487385993,1.89587041543437,304.974475946787));
#9054=CARTESIAN_POINT('Ctrl Pts',(-3.56753031259803,-1.96275979652795,305.170892230348));
#9055=CARTESIAN_POINT('Ctrl Pts',(-0.327535413996504,-4.05861519118165,
305.367308513907));
#9056=CARTESIAN_POINT('Ctrl Pts',(3.20663944956988,-2.50944712830294,305.563724797468));
#9057=CARTESIAN_POINT('Ctrl Pts',(3.86088059109964,1.29352830991355,305.760141081028));
#9058=CARTESIAN_POINT('Ctrl Pts',(1.04774156211884,3.93464263737925,305.956557364589));
#9059=CARTESIAN_POINT('Ctrl Pts',(-2.70656494368751,3.04233932786737,306.152973648148));
#9060=CARTESIAN_POINT('Ctrl Pts',(-4.02969985274476,-0.582931827771558,
306.349389931709));
#9061=CARTESIAN_POINT('Ctrl Pts',(-1.73460718039984,-3.68333889913998,306.545806215269));
#9062=CARTESIAN_POINT('Ctrl Pts',(2.12009592649099,-3.47867745500165,306.742222498829));
#9063=CARTESIAN_POINT('Ctrl Pts',(4.066986376797,-0.14343323816737,306.938682380056));
#9064=CARTESIAN_POINT('Ctrl Pts',(2.93277505209188,2.15491985457359,307.069670166764));
#9065=CARTESIAN_POINT('Ctrl Pts',(2.00558448788872,2.81535315694411,307.135185858951));
#9066=CARTESIAN_POINT('Ctrl Pts',(1.64344736484494,-3.31083465017304,296.863334289856));
#9067=CARTESIAN_POINT('Ctrl Pts',(2.73303855162352,-2.76997835444232,296.928806384376));
#9068=CARTESIAN_POINT('Ctrl Pts',(4.31806526539767,-0.53579067117003,297.059750573417));
#9069=CARTESIAN_POINT('Ctrl Pts',(2.82705787200949,3.31426585664044,297.256166856977));
#9070=CARTESIAN_POINT('Ctrl Pts',(-1.20830520117628,4.1825310018776,297.452583140537));
#9071=CARTESIAN_POINT('Ctrl Pts',(-4.15613426352052,1.29726957454531,297.648999424097));
#9072=CARTESIAN_POINT('Ctrl Pts',(-3.37245777205994,-2.75433400689091,297.845415707658));
#9073=CARTESIAN_POINT('Ctrl Pts',(0.440560090246934,-4.33166004160428,298.041831991218));
#9074=CARTESIAN_POINT('Ctrl Pts',(3.85766129590832,-2.01899074338315,298.238248274778));
#9075=CARTESIAN_POINT('Ctrl Pts',(3.81030211394735,2.10707250760402,298.434664558338));
#9076=CARTESIAN_POINT('Ctrl Pts',(0.34084459659878,4.34070555836707,298.631080841898));
#9077=CARTESIAN_POINT('Ctrl Pts',(-3.43470071493533,2.67596739227649,298.827497125458));
#9078=CARTESIAN_POINT('Ctrl Pts',(-4.12554329970309,-1.3920786942064,299.023913409019));
#9079=CARTESIAN_POINT('Ctrl Pts',(-1.11121762092136,-4.20988835720045,299.220329692579));
#9080=CARTESIAN_POINT('Ctrl Pts',(2.90109320386305,-3.24678792599277,299.416745976139));
#9081=CARTESIAN_POINT('Ctrl Pts',(4.30792493768307,0.63226372230056,299.6131622597));
#9082=CARTESIAN_POINT('Ctrl Pts',(1.84579601545559,3.94347679146638,299.80957854326));
#9083=CARTESIAN_POINT('Ctrl Pts',(-2.27404746424881,3.71304206127767,300.00599482682));
#9084=CARTESIAN_POINT('Ctrl Pts',(-4.35156235295879,0.147913179084922,300.20241111038));
#9085=CARTESIAN_POINT('Ctrl Pts',(-2.52092622284173,-3.55005689521063,300.398827393941));
#9086=CARTESIAN_POINT('Ctrl Pts',(1.57376113943488,-4.05971045520627,300.595243677501));
#9087=CARTESIAN_POINT('Ctrl Pts',(4.25504900363738,-0.923326090611326,300.791659961061));
#9088=CARTESIAN_POINT('Ctrl Pts',(3.11486482691945,3.04230014650195,300.988076244621));
#9089=CARTESIAN_POINT('Ctrl Pts',(-0.822788616242238,4.27562767064716,301.184492528181));
#9090=CARTESIAN_POINT('Ctrl Pts',(-4.02149318274018,1.66900139720936,301.380908811742));
#9091=CARTESIAN_POINT('Ctrl Pts',(-3.60848288420596,-2.43655994288933,301.577325095302));
#9092=CARTESIAN_POINT('Ctrl Pts',(0.0453165136240533,-4.35383962681091,
301.773741378862));
#9093=CARTESIAN_POINT('Ctrl Pts',(3.65841701731566,-2.36092312651506,301.970157662422));
#9094=CARTESIAN_POINT('Ctrl Pts',(3.98588242944266,1.75234538278242,302.166573945982));
#9095=CARTESIAN_POINT('Ctrl Pts',(0.73361509952361,4.29182734603186,302.362990229543));
#9096=CARTESIAN_POINT('Ctrl Pts',(-3.17751411051533,2.97680653694124,302.559406513103));
#9097=CARTESIAN_POINT('Ctrl Pts',(-4.23490854537298,-1.01169298457562,302.755822796663));
#9098=CARTESIAN_POINT('Ctrl Pts',(-1.48891914997317,-4.09158805964929,302.952239080224));
#9099=CARTESIAN_POINT('Ctrl Pts',(2.59427291540787,-3.49681585328236,303.148655363783));
#9100=CARTESIAN_POINT('Ctrl Pts',(4.34754084182337,0.238456959715606,303.345071647344));
#9101=CARTESIAN_POINT('Ctrl Pts',(2.19626953641995,3.75957088342543,303.541487930904));
#9102=CARTESIAN_POINT('Ctrl Pts',(-1.92747789329011,3.90420311345624,303.737904214464));
#9103=CARTESIAN_POINT('Ctrl Pts',(-4.32015177685929,0.542459072313112,303.934320498024));
#9104=CARTESIAN_POINT('Ctrl Pts',(-2.83288458420245,-3.30646913656574,304.130736781585));
#9105=CARTESIAN_POINT('Ctrl Pts',(1.19860448678435,-4.18584751511162,304.327153065145));
#9106=CARTESIAN_POINT('Ctrl Pts',(4.15362356392177,-1.30590427385887,304.523569348705));
#9107=CARTESIAN_POINT('Ctrl Pts',(3.37826061625335,2.74687619352316,304.719985632265));
#9108=CARTESIAN_POINT('Ctrl Pts',(-0.431127121075381,4.33267746164092,304.916401915826));
#9109=CARTESIAN_POINT('Ctrl Pts',(-3.8533204789238,2.02729176373184,305.112818199386));
#9110=CARTESIAN_POINT('Ctrl Pts',(-3.81483078205882,-2.09881790300179,305.309234482946));
#9111=CARTESIAN_POINT('Ctrl Pts',(-0.350240101707314,-4.33995756368946,
305.505650766506));
#9112=CARTESIAN_POINT('Ctrl Pts',(3.42892303843518,-2.6834014884733,305.702067050067));
#9113=CARTESIAN_POINT('Ctrl Pts',(4.12851604169113,1.38319542701492,305.898483333627));
#9114=CARTESIAN_POINT('Ctrl Pts',(1.1203707922814,4.20739125788799,306.094899617187));
#9115=CARTESIAN_POINT('Ctrl Pts',(-2.89418347038547,3.2532336659992,306.291315900747));
#9116=CARTESIAN_POINT('Ctrl Pts',(-4.30903781992354,-0.623340542495704,
306.487732184307));
#9117=CARTESIAN_POINT('Ctrl Pts',(-1.8548497943247,-3.93866719606399,306.684148467868));
#9118=CARTESIAN_POINT('Ctrl Pts',(2.26706054121946,-3.71981866260025,306.880564751428));
#9119=CARTESIAN_POINT('Ctrl Pts',(4.34890903817448,-0.153376000814643,307.077024632655));
#9120=CARTESIAN_POINT('Ctrl Pts',(3.1360744171019,2.3042984568533,307.208012419362));
#9121=CARTESIAN_POINT('Ctrl Pts',(2.14461119318305,3.01051286026928,307.273528111549));
#9122=CARTESIAN_POINT('Ctrl Pts',(1.74998559106762,-3.5254630334674,297.001676542455));
#9123=CARTESIAN_POINT('Ctrl Pts',(2.91021068729191,-2.94954515218115,297.067148636975));
#9124=CARTESIAN_POINT('Ctrl Pts',(4.59798844634642,-0.570523872216909,297.198092826015));
#9125=CARTESIAN_POINT('Ctrl Pts',(3.01032491028253,3.52911667154937,297.394509109576));
#9126=CARTESIAN_POINT('Ctrl Pts',(-1.28663487307368,4.45366802980637,297.590925393136));
#9127=CARTESIAN_POINT('Ctrl Pts',(-4.42556009476432,1.38136645672185,297.787341676696));
#9128=CARTESIAN_POINT('Ctrl Pts',(-3.59108093987892,-2.93288664313347,297.983757960256));
#9129=CARTESIAN_POINT('Ctrl Pts',(0.469119867434461,-4.6124645184034,298.180174243816));
#9130=CARTESIAN_POINT('Ctrl Pts',(4.10773829905756,-2.14987396919328,298.376590527377));
#9131=CARTESIAN_POINT('Ctrl Pts',(4.05730900767332,2.24366572761499,298.573006810937));
#9132=CARTESIAN_POINT('Ctrl Pts',(0.362940210681713,4.62209642042671,298.769423094497));
#9133=CARTESIAN_POINT('Ctrl Pts',(-3.65735884783482,2.8494398292412,298.965839378057));
#9134=CARTESIAN_POINT('Ctrl Pts',(-4.39298603912828,-1.48232167856698,299.162255661618));
#9135=CARTESIAN_POINT('Ctrl Pts',(-1.18325348699944,-4.48279885483234,299.358671945178));
#9136=CARTESIAN_POINT('Ctrl Pts',(3.08915966139477,-3.4572644121619,299.555088228738));
#9137=CARTESIAN_POINT('Ctrl Pts',(4.58719076108503,0.673250891661594,299.751504512298));
#9138=CARTESIAN_POINT('Ctrl Pts',(1.96545170852008,4.19911687553611,299.947920795858));
#9139=CARTESIAN_POINT('Ctrl Pts',(-2.42146501370596,3.9537439684763,300.144337079419));
#9140=CARTESIAN_POINT('Ctrl Pts',(-4.63365701829379,0.157501808493909,300.340753362979));
#9141=CARTESIAN_POINT('Ctrl Pts',(-2.68434795082944,-3.78019311538766,300.537169646539));
#9142=CARTESIAN_POINT('Ctrl Pts',(1.67578188185725,-4.32288551035394,300.733585930099));
#9143=CARTESIAN_POINT('Ctrl Pts',(4.53088708828506,-0.983181688072545,300.93000221366));
#9144=CARTESIAN_POINT('Ctrl Pts',(3.31678925765091,3.23952049452076,301.12641849722));
#9145=CARTESIAN_POINT('Ctrl Pts',(-0.876126764822934,4.55279978930661,301.32283478078));
#9146=CARTESIAN_POINT('Ctrl Pts',(-4.28219076248663,1.77719619080327,301.51925106434));
#9147=CARTESIAN_POINT('Ctrl Pts',(-3.84240663136197,-2.59451253690207,301.7156673479));
#9148=CARTESIAN_POINT('Ctrl Pts',(0.0482542048962955,-4.6360819188494,301.912083631461));
#9149=CARTESIAN_POINT('Ctrl Pts',(3.89557779784632,-2.51397248332897,302.108499915021));
#9150=CARTESIAN_POINT('Ctrl Pts',(4.24427150416976,1.86594303902907,302.304916198581));
#9151=CARTESIAN_POINT('Ctrl Pts',(0.781172479884741,4.57004962590596,302.501332482141));
#9152=CARTESIAN_POINT('Ctrl Pts',(-3.38349984779739,3.16978119194865,302.697748765702));
#9153=CARTESIAN_POINT('Ctrl Pts',(-4.50944100335765,-1.07727706007705,302.894165049262));
#9154=CARTESIAN_POINT('Ctrl Pts',(-1.58543992004487,-4.3568296144648,303.090581332822));
#9155=CARTESIAN_POINT('Ctrl Pts',(2.76244942087883,-3.72350066619769,303.286997616382));
#9156=CARTESIAN_POINT('Ctrl Pts',(4.62937480841483,0.253915186162026,303.483413899943));
#9157=CARTESIAN_POINT('Ctrl Pts',(2.33864504884725,4.00328907108784,303.679830183503));
#9158=CARTESIAN_POINT('Ctrl Pts',(-2.05242870110252,4.15729723950994,303.876246467063));
#9159=CARTESIAN_POINT('Ctrl Pts',(-4.60021021813634,0.577624559568071,304.072662750623));
#9160=CARTESIAN_POINT('Ctrl Pts',(-3.01652934530071,-3.52081452078982,304.269079034184));
#9161=CARTESIAN_POINT('Ctrl Pts',(1.27630529953692,-4.45719953954392,304.465495317743));
#9162=CARTESIAN_POINT('Ctrl Pts',(4.42288663638938,-1.39056090961712,304.661911601304));
#9163=CARTESIAN_POINT('Ctrl Pts',(3.59725995962907,2.9249453690692,304.858327884864));
#9164=CARTESIAN_POINT('Ctrl Pts',(-0.459075395987237,4.61354789377779,305.054744168424));
#9165=CARTESIAN_POINT('Ctrl Pts',(-4.10311608398768,2.15871311202932,305.251160451984));
#9166=CARTESIAN_POINT('Ctrl Pts',(-4.0621312515196,-2.23487600947561,305.447576735545));
#9167=CARTESIAN_POINT('Ctrl Pts',(-0.372944789418124,-4.62129993619727,
305.643993019105));
#9168=CARTESIAN_POINT('Ctrl Pts',(3.6512066273005,-2.85735584864364,305.840409302665));
#9169=CARTESIAN_POINT('Ctrl Pts',(4.39615149228261,1.47286254411629,306.036825586225));
#9170=CARTESIAN_POINT('Ctrl Pts',(1.19300002244395,4.48013987839675,306.233241869786));
#9171=CARTESIAN_POINT('Ctrl Pts',(-3.08180199708344,3.46412800413103,306.429658153346));
#9172=CARTESIAN_POINT('Ctrl Pts',(-4.58837578710231,-0.663749257219848,
306.626074436906));
#9173=CARTESIAN_POINT('Ctrl Pts',(-1.97509240824956,-4.19399549298801,306.822490720466));
#9174=CARTESIAN_POINT('Ctrl Pts',(2.41402515594792,-3.96095987019886,307.018907004026));
#9175=CARTESIAN_POINT('Ctrl Pts',(4.63083169955196,-0.163318763461907,307.215366885254));
#9176=CARTESIAN_POINT('Ctrl Pts',(3.33937378211193,2.45367705913301,307.346354671961));
#9177=CARTESIAN_POINT('Ctrl Pts',(2.28363789847738,3.20567256359444,307.411870364148));
#9178=CARTESIAN_POINT('Ctrl Pts',(1.75295277484312,-3.52741701688456,307.));
#9179=CARTESIAN_POINT('Ctrl Pts',(1.84997325411491,-3.46888291556181,307.));
#9180=CARTESIAN_POINT('Ctrl Pts',(1.94403576147925,-3.40606933859778,307.));
#9181=CARTESIAN_POINT('Ctrl Pts',(2.03481898164511,-3.33898497869234,307.));
#9182=CARTESIAN_POINT('Ctrl Pts',(2.13159970155574,-3.26746875978613,307.));
#9183=CARTESIAN_POINT('Ctrl Pts',(2.2246543845738,-3.19109872939616,307.));
#9184=CARTESIAN_POINT('Ctrl Pts',(2.31382658373371,-3.110286348705,307.));
#9185=CARTESIAN_POINT('Ctrl Pts',(2.40455794825776,-3.02806097308767,307.));
#9186=CARTESIAN_POINT('Ctrl Pts',(2.49127034422638,-2.94123570859823,307.));
#9187=CARTESIAN_POINT('Ctrl Pts',(2.57375432305174,-2.85021295057718,307.));
#9188=CARTESIAN_POINT('Ctrl Pts',(2.65623830187711,-2.75919019255613,307.));
#9189=CARTESIAN_POINT('Ctrl Pts',(2.73449421814026,-2.66396901625497,307.));
#9190=CARTESIAN_POINT('Ctrl Pts',(2.80826230895727,-2.56493446116125,307.));
#9191=CARTESIAN_POINT('Ctrl Pts',(2.81895233475812,-2.55058297209054,307.));
#9192=CARTESIAN_POINT('Ctrl Pts',(2.82954802439101,-2.53615138610789,307.));
#9193=CARTESIAN_POINT('Ctrl Pts',(2.84004849278268,-2.52164086262617,307.));
#9194=CARTESIAN_POINT('Ctrl Pts',(2.85054939974663,-2.5071297330845,307.));
#9195=CARTESIAN_POINT('Ctrl Pts',(2.86095084159264,-2.49254545377891,307.));
#9196=CARTESIAN_POINT('Ctrl Pts',(2.87124786780565,-2.47789562877494,307.));
#9197=CARTESIAN_POINT('Ctrl Pts',(2.94008136874243,-2.37996456379809,307.));
#9198=CARTESIAN_POINT('Ctrl Pts',(3.00431541770822,-2.27902010980789,307.));
#9199=CARTESIAN_POINT('Ctrl Pts',(3.0637933403493,-2.17545767538768,307.));
#9200=CARTESIAN_POINT('Ctrl Pts',(3.12323362815573,-2.07196077040969,307.));
#9201=CARTESIAN_POINT('Ctrl Pts',(3.17792410148909,-1.96584830416904,307.));
#9202=CARTESIAN_POINT('Ctrl Pts',(3.2276602081122,-1.85749568873033,307.));
#9203=CARTESIAN_POINT('Ctrl Pts',(3.27649169173924,-1.75111384008994,307.));
#9204=CARTESIAN_POINT('Ctrl Pts',(3.3205475227483,-1.64257176239661,307.));
#9205=CARTESIAN_POINT('Ctrl Pts',(3.35958475361651,-1.5322189723795,307.));
#9206=CARTESIAN_POINT('Ctrl Pts',(3.37957181235439,-1.47571835369042,307.));
#9207=CARTESIAN_POINT('Ctrl Pts',(3.3982424616149,-1.4187430500264,307.));
#9208=CARTESIAN_POINT('Ctrl Pts',(3.41555877354041,-1.36134041511221,307.));
#9209=CARTESIAN_POINT('Ctrl Pts',(3.42952961902185,-1.3150278200248,307.));
#9210=CARTESIAN_POINT('Ctrl Pts',(3.44261881817217,-1.26843706414811,307.));
#9211=CARTESIAN_POINT('Ctrl Pts',(3.45480465835639,-1.22159339689648,307.));
#9212=CARTESIAN_POINT('Ctrl Pts',(3.45882230994349,-1.20614911638451,307.));
#9213=CARTESIAN_POINT('Ctrl Pts',(3.46274127720411,-1.19067897371837,307.));
#9214=CARTESIAN_POINT('Ctrl Pts',(3.46655813556577,-1.17519536513956,307.));
#9215=CARTESIAN_POINT('Ctrl Pts',(3.49407224813524,-1.06358060004956,307.));
#9216=CARTESIAN_POINT('Ctrl Pts',(3.51632768255355,-0.95110272169328,307.));
#9217=CARTESIAN_POINT('Ctrl Pts',(3.53314119320375,-0.83810325534612,307.));
#9218=CARTESIAN_POINT('Ctrl Pts',(3.54951998604572,-0.728025420380012,307.));
#9219=CARTESIAN_POINT('Ctrl Pts',(3.56073462608323,-0.617451900568752,307.));
#9220=CARTESIAN_POINT('Ctrl Pts',(3.56656734873009,-0.506699353783957,307.));
#9221=CARTESIAN_POINT('Ctrl Pts',(3.57237373653643,-0.39644685660448,307.));
#9222=CARTESIAN_POINT('Ctrl Pts',(3.57284686430163,-0.286016286590276,307.));
#9223=CARTESIAN_POINT('Ctrl Pts',(3.56772180702459,-0.175731148929752,307.));
#9224=CARTESIAN_POINT('Ctrl Pts',(3.56700386529454,-0.160281896706627,307.));
#9225=CARTESIAN_POINT('Ctrl Pts',(3.56617598339815,-0.144835525589673,307.));
#9226=CARTESIAN_POINT('Ctrl Pts',(3.56523735115947,-0.129392953786932,307.));
#9227=CARTESIAN_POINT('Ctrl Pts',(3.56100709348304,-0.059795879213749,307.));
#9228=CARTESIAN_POINT('Ctrl Pts',(3.55452777976943,0.00972434142671849,
307.));
#9229=CARTESIAN_POINT('Ctrl Pts',(3.54583829760014,0.0790805148444869,307.));
#9230=CARTESIAN_POINT('Ctrl Pts',(3.54239356966496,0.106575035621981,307.));
#9231=CARTESIAN_POINT('Ctrl Pts',(3.53860144372464,0.134043731144043,307.));
#9232=CARTESIAN_POINT('Ctrl Pts',(3.53446410048778,0.161480979003646,307.));
#9233=CARTESIAN_POINT('Ctrl Pts',(3.53224607865982,0.176190035315359,307.));
#9234=CARTESIAN_POINT('Ctrl Pts',(3.52992929936332,0.190886746487658,307.));
#9235=CARTESIAN_POINT('Ctrl Pts',(3.52751569347095,0.20556195564389,307.));
#9236=CARTESIAN_POINT('Ctrl Pts',(3.50945137554655,0.315396641018207,307.));
#9237=CARTESIAN_POINT('Ctrl Pts',(3.48594688677709,0.424166839182885,307.));
#9238=CARTESIAN_POINT('Ctrl Pts',(3.45725530888715,0.531549258372834,307.));
#9239=CARTESIAN_POINT('Ctrl Pts',(3.42830185569478,0.639911784115604,307.));
#9240=CARTESIAN_POINT('Ctrl Pts',(3.39406567191996,0.746861877867126,307.));
#9241=CARTESIAN_POINT('Ctrl Pts',(3.3547574652526,0.852046538270801,307.));
#9242=CARTESIAN_POINT('Ctrl Pts',(3.31573092144832,0.956477498236013,307.));
#9243=CARTESIAN_POINT('Ctrl Pts',(3.27170416736303,1.05916893424089,307.));
#9244=CARTESIAN_POINT('Ctrl Pts',(3.2228436680777,1.15974389177418,307.));
#9245=CARTESIAN_POINT('Ctrl Pts',(3.18636005117348,1.23484214648859,307.));
#9246=CARTESIAN_POINT('Ctrl Pts',(3.14718054401227,1.30875978471779,307.));
#9247=CARTESIAN_POINT('Ctrl Pts',(3.10536284645011,1.38132480753957,307.));
#9248=CARTESIAN_POINT('Ctrl Pts',(3.09616761950596,1.39728101488604,307.));
#9249=CARTESIAN_POINT('Ctrl Pts',(3.08684392630523,1.41317322762995,307.));
#9250=CARTESIAN_POINT('Ctrl Pts',(3.07739507132796,1.42899493090577,307.));
#9251=CARTESIAN_POINT('Ctrl Pts',(3.0208896010318,1.52361092264631,307.));
#9252=CARTESIAN_POINT('Ctrl Pts',(2.9600630238022,1.61545588204263,307.));
#9253=CARTESIAN_POINT('Ctrl Pts',(2.89510248933946,1.70417986891544,307.));
#9254=CARTESIAN_POINT('Ctrl Pts',(2.83126422465857,1.79137104436335,307.));
#9255=CARTESIAN_POINT('Ctrl Pts',(2.76343297954024,1.87554869262835,307.));
#9256=CARTESIAN_POINT('Ctrl Pts',(2.69175573855431,1.95634128855535,307.));
#9257=CARTESIAN_POINT('Ctrl Pts',(2.66214252473009,1.98972048096971,307.));
#9258=CARTESIAN_POINT('Ctrl Pts',(2.6318725241643,2.02252136225033,307.));
#9259=CARTESIAN_POINT('Ctrl Pts',(2.60095491029651,2.05471539319883,307.));
#9260=CARTESIAN_POINT('Ctrl Pts',(2.58369001395723,2.07269306150938,307.));
#9261=CARTESIAN_POINT('Ctrl Pts',(2.56622316200388,2.09048147053325,307.));
#9262=CARTESIAN_POINT('Ctrl Pts',(2.54855587341939,2.10807544530337,307.));
#9263=CARTESIAN_POINT('Ctrl Pts',(2.5342735759129,2.12229847566746,307.));
#9264=CARTESIAN_POINT('Ctrl Pts',(2.51986594619975,2.1363887535211,307.));
#9265=CARTESIAN_POINT('Ctrl Pts',(2.50533827639883,2.15033988947171,307.));
#9266=CARTESIAN_POINT('Ctrl Pts',(2.42916611523439,2.22348914125257,307.));
#9267=CARTESIAN_POINT('Ctrl Pts',(2.34965953843726,2.2928529993755,307.));
#9268=CARTESIAN_POINT('Ctrl Pts',(2.26696419899973,2.35808473048493,307.));
#9269=CARTESIAN_POINT('Ctrl Pts',(2.18652064639967,2.42154020727947,307.));
#9270=CARTESIAN_POINT('Ctrl Pts',(2.10305907939019,2.4810858444035,307.));
#9271=CARTESIAN_POINT('Ctrl Pts',(2.0166946005239,2.53635740752467,307.));
#9272=CARTESIAN_POINT('Ctrl Pts',(1.96919770923866,2.56675448117339,307.));
#9273=CARTESIAN_POINT('Ctrl Pts',(1.92082252976015,2.59585801512022,307.));
#9274=CARTESIAN_POINT('Ctrl Pts',(1.87158653173908,2.62360084935054,307.));
#9275=CARTESIAN_POINT('Ctrl Pts',(1.8756224353083,2.62673419576125,297.));
#9276=CARTESIAN_POINT('Ctrl Pts',(1.95765324669421,2.58118494599767,297.));
#9277=CARTESIAN_POINT('Ctrl Pts',(2.03738954822689,2.53196003294659,297.));
#9278=CARTESIAN_POINT('Ctrl Pts',(2.11454810562212,2.47911826575738,297.));
#9279=CARTESIAN_POINT('Ctrl Pts',(2.19986126849811,2.42069184562907,297.));
#9280=CARTESIAN_POINT('Ctrl Pts',(2.28202434826617,2.35784481146803,297.));
#9281=CARTESIAN_POINT('Ctrl Pts',(2.36094618439224,2.2909673251695,297.));
#9282=CARTESIAN_POINT('Ctrl Pts',(2.40953886514322,2.24979042786644,297.));
#9283=CARTESIAN_POINT('Ctrl Pts',(2.45690244537228,2.20708458165014,297.));
#9284=CARTESIAN_POINT('Ctrl Pts',(2.50301134826845,2.1629320969333,297.));
#9285=CARTESIAN_POINT('Ctrl Pts',(2.51681233550409,2.14971669080293,297.));
#9286=CARTESIAN_POINT('Ctrl Pts',(2.53050089340508,2.13637164146357,297.));
#9287=CARTESIAN_POINT('Ctrl Pts',(2.54407626948497,2.12289905300282,297.));
#9288=CARTESIAN_POINT('Ctrl Pts',(2.55828158733512,2.10880129245292,297.));
#9289=CARTESIAN_POINT('Ctrl Pts',(2.5723574584733,2.09456930457899,297.));
#9290=CARTESIAN_POINT('Ctrl Pts',(2.58629903742493,2.08021029150632,297.));
#9291=CARTESIAN_POINT('Ctrl Pts',(2.66022714209237,2.00406865611193,297.));
#9292=CARTESIAN_POINT('Ctrl Pts',(2.73041918130771,1.92432121396313,297.));
#9293=CARTESIAN_POINT('Ctrl Pts',(2.79678221780539,1.84137617106676,297.));
#9294=CARTESIAN_POINT('Ctrl Pts',(2.86479487312921,1.75636932220854,297.));
#9295=CARTESIAN_POINT('Ctrl Pts',(2.92878637777531,1.66800343120733,297.));
#9296=CARTESIAN_POINT('Ctrl Pts',(2.98862845706434,1.57667128181542,297.));
#9297=CARTESIAN_POINT('Ctrl Pts',(3.01039937231069,1.54344408604781,297.));
#9298=CARTESIAN_POINT('Ctrl Pts',(3.03162078208611,1.50982389187596,297.));
#9299=CARTESIAN_POINT('Ctrl Pts',(3.05228537984315,1.47582834566168,297.));
#9300=CARTESIAN_POINT('Ctrl Pts',(3.06150211787551,1.46066579338712,297.));
#9301=CARTESIAN_POINT('Ctrl Pts',(3.07060854300814,1.44542777629857,297.));
#9302=CARTESIAN_POINT('Ctrl Pts',(3.07960253589492,1.43011825637885,297.));
#9303=CARTESIAN_POINT('Ctrl Pts',(3.08792329757299,1.41595470652269,297.));
#9304=CARTESIAN_POINT('Ctrl Pts',(3.09614466223841,1.40173534905011,297.));
#9305=CARTESIAN_POINT('Ctrl Pts',(3.10426515935106,1.3874636942554,297.));
#9306=CARTESIAN_POINT('Ctrl Pts',(3.1594813980601,1.29042196306753,297.));
#9307=CARTESIAN_POINT('Ctrl Pts',(3.21005549239299,1.1909335558491,297.));
#9308=CARTESIAN_POINT('Ctrl Pts',(3.25588594072735,1.08943234816672,297.));
#9309=CARTESIAN_POINT('Ctrl Pts',(3.30225956579053,0.986728160894039,297.));
#9310=CARTESIAN_POINT('Ctrl Pts',(3.34377699428959,0.881962476690267,297.));
#9311=CARTESIAN_POINT('Ctrl Pts',(3.38029857606622,0.775543280911798,297.));
#9312=CARTESIAN_POINT('Ctrl Pts',(3.41675039082397,0.669327377260349,297.));
#9313=CARTESIAN_POINT('Ctrl Pts',(3.44822592417807,0.561463458521685,297.));
#9314=CARTESIAN_POINT('Ctrl Pts',(3.47454435174328,0.452327636711442,297.));
#9315=CARTESIAN_POINT('Ctrl Pts',(3.49204141362862,0.379771773585114,297.));
#9316=CARTESIAN_POINT('Ctrl Pts',(3.50725822641119,0.30665315370922,297.));
#9317=CARTESIAN_POINT('Ctrl Pts',(3.5201296905142,0.233077758113266,297.));
#9318=CARTESIAN_POINT('Ctrl Pts',(3.52324750007939,0.215255848319997,297.));
#9319=CARTESIAN_POINT('Ctrl Pts',(3.5262276519985,0.197407126484436,297.));
#9320=CARTESIAN_POINT('Ctrl Pts',(3.52906912818209,0.179533080052531,297.));
#9321=CARTESIAN_POINT('Ctrl Pts',(3.53130134307825,0.165491536107698,297.));
#9322=CARTESIAN_POINT('Ctrl Pts',(3.53344765401367,0.151436138428793,297.));
#9323=CARTESIAN_POINT('Ctrl Pts',(3.53550638032799,0.137376848547553,297.));
#9324=CARTESIAN_POINT('Ctrl Pts',(3.55229157977818,0.0227487004818831,297.));
#9325=CARTESIAN_POINT('Ctrl Pts',(3.56328560075331,-0.0923062269536467,
297.));
#9326=CARTESIAN_POINT('Ctrl Pts',(3.56835208320539,-0.207362631195156,297.));
#9327=CARTESIAN_POINT('Ctrl Pts',(3.57176836951555,-0.284944192450943,297.));
#9328=CARTESIAN_POINT('Ctrl Pts',(3.57248877647768,-0.362527172824792,297.));
#9329=CARTESIAN_POINT('Ctrl Pts',(3.57045975383798,-0.439987598678934,297.));
#9330=CARTESIAN_POINT('Ctrl Pts',(3.5675206935761,-0.55218982601893,297.));
#9331=CARTESIAN_POINT('Ctrl Pts',(3.55881561640657,-0.664134903948192,297.));
#9332=CARTESIAN_POINT('Ctrl Pts',(3.54461270917885,-0.77552871598842,297.));
#9333=CARTESIAN_POINT('Ctrl Pts',(3.53040980195112,-0.886922528028648,297.));
#9334=CARTESIAN_POINT('Ctrl Pts',(3.51070879796927,-0.997765757946331,297.));
#9335=CARTESIAN_POINT('Ctrl Pts',(3.48572532531809,-1.10776627052454,297.));
#9336=CARTESIAN_POINT('Ctrl Pts',(3.48023441116192,-1.13194238807772,297.));
#9337=CARTESIAN_POINT('Ctrl Pts',(3.47448813976633,-1.15607778380368,297.));
#9338=CARTESIAN_POINT('Ctrl Pts',(3.46848847990599,-1.18016931768953,297.));
#9339=CARTESIAN_POINT('Ctrl Pts',(3.46260502329978,-1.20379423935069,297.));
#9340=CARTESIAN_POINT('Ctrl Pts',(3.4564769563925,-1.22737979626238,297.));
#9341=CARTESIAN_POINT('Ctrl Pts',(3.4501156361031,-1.25088950819066,297.));
#9342=CARTESIAN_POINT('Ctrl Pts',(3.41996601999333,-1.3623143000959,297.));
#9343=CARTESIAN_POINT('Ctrl Pts',(3.38454132687335,-1.47220190710762,297.));
#9344=CARTESIAN_POINT('Ctrl Pts',(3.34415317658468,-1.58024732335799,297.));
#9345=CARTESIAN_POINT('Ctrl Pts',(3.30309881449456,-1.69007497352804,297.));
#9346=CARTESIAN_POINT('Ctrl Pts',(3.25691572359613,-1.7979998724566,297.));
#9347=CARTESIAN_POINT('Ctrl Pts',(3.20587623943613,-1.90370463532879,297.));
#9348=CARTESIAN_POINT('Ctrl Pts',(3.15419187937227,-2.01074496135608,297.));
#9349=CARTESIAN_POINT('Ctrl Pts',(3.09752739549888,-2.11550950113078,297.));
#9350=CARTESIAN_POINT('Ctrl Pts',(3.03611285331182,-2.21766010847631,297.));
#9351=CARTESIAN_POINT('Ctrl Pts',(2.98506113429581,-2.30257426590232,297.));
#9352=CARTESIAN_POINT('Ctrl Pts',(2.93072608037477,-2.38568227462021,297.));
#9353=CARTESIAN_POINT('Ctrl Pts',(2.87321456924896,-2.4667792858147,297.));
#9354=CARTESIAN_POINT('Ctrl Pts',(2.86373431057747,-2.48014740340644,297.));
#9355=CARTESIAN_POINT('Ctrl Pts',(2.85416769185057,-2.49346084869992,297.));
#9356=CARTESIAN_POINT('Ctrl Pts',(2.8445151364034,-2.50671866846762,297.));
#9357=CARTESIAN_POINT('Ctrl Pts',(2.83449211073775,-2.52048533041839,297.));
#9358=CARTESIAN_POINT('Ctrl Pts',(2.8243817964104,-2.5341846142502,297.));
#9359=CARTESIAN_POINT('Ctrl Pts',(2.81418689372382,-2.54781310286705,297.));
#9360=CARTESIAN_POINT('Ctrl Pts',(2.74077335186671,-2.64595191304319,297.));
#9361=CARTESIAN_POINT('Ctrl Pts',(2.66294685987612,-2.74046301248844,297.));
#9362=CARTESIAN_POINT('Ctrl Pts',(2.58099765137135,-2.83101116490618,297.));
#9363=CARTESIAN_POINT('Ctrl Pts',(2.49890799991651,-2.92171449697581,297.));
#9364=CARTESIAN_POINT('Ctrl Pts',(2.41268110510993,-3.00844211791462,297.));
#9365=CARTESIAN_POINT('Ctrl Pts',(2.32255885079943,-3.09084082744064,297.));
#9366=CARTESIAN_POINT('Ctrl Pts',(2.23414169014168,-3.17168057111874,297.));
#9367=CARTESIAN_POINT('Ctrl Pts',(2.14197466942637,-3.2483543632461,297.));
#9368=CARTESIAN_POINT('Ctrl Pts',(2.04624509609143,-3.3205018093572,297.));
#9369=CARTESIAN_POINT('Ctrl Pts',(1.95056982624481,-3.39260832916037,297.));
#9370=CARTESIAN_POINT('Ctrl Pts',(1.85133567663837,-3.46019442836626,297.));
#9371=CARTESIAN_POINT('Ctrl Pts',(1.74869447533122,-3.52286199445083,297.));
#9372=CARTESIAN_POINT('Origin',(-5.160062080289E-16,2.1385152528819E-16,
297.));
#9373=CARTESIAN_POINT('Ctrl Pts',(-1.81480609505069,-3.48926465567845,297.));
#9374=CARTESIAN_POINT('Ctrl Pts',(-1.89001899604713,-3.44184200468758,297.));
#9375=CARTESIAN_POINT('Ctrl Pts',(-1.96341204602375,-3.39175063166926,297.));
#9376=CARTESIAN_POINT('Ctrl Pts',(-2.03481909388391,-3.33898430436496,297.));
#9377=CARTESIAN_POINT('Ctrl Pts',(-2.1330728566162,-3.26637956353652,297.));
#9378=CARTESIAN_POINT('Ctrl Pts',(-2.22756835178525,-3.18871116509068,297.));
#9379=CARTESIAN_POINT('Ctrl Pts',(-2.31811726774695,-3.10639114222592,297.));
#9380=CARTESIAN_POINT('Ctrl Pts',(-2.38810348676451,-3.04276512209577,297.));
#9381=CARTESIAN_POINT('Ctrl Pts',(-2.45573128771564,-2.97635938300247,297.));
#9382=CARTESIAN_POINT('Ctrl Pts',(-2.5208950964127,-2.90735384839687,297.));
#9383=CARTESIAN_POINT('Ctrl Pts',(-2.53489034792619,-2.89253350821206,297.));
#9384=CARTESIAN_POINT('Ctrl Pts',(-2.54877166048973,-2.8775933504051,297.));
#9385=CARTESIAN_POINT('Ctrl Pts',(-2.56252866764529,-2.86254555233852,297.));
#9386=CARTESIAN_POINT('Ctrl Pts',(-2.64400028421257,-2.77342962614914,297.));
#9387=CARTESIAN_POINT('Ctrl Pts',(-2.7212018811122,-2.68045059264905,297.));
#9388=CARTESIAN_POINT('Ctrl Pts',(-2.79395934645943,-2.58401337193643,297.));
#9389=CARTESIAN_POINT('Ctrl Pts',(-2.86676825659545,-2.4875079631358,297.));
#9390=CARTESIAN_POINT('Ctrl Pts',(-2.93512707424484,-2.38753858357703,297.));
#9391=CARTESIAN_POINT('Ctrl Pts',(-2.99881400156226,-2.28449030256758,297.));
#9392=CARTESIAN_POINT('Ctrl Pts',(-3.03468906634645,-2.2264428521279,297.));
#9393=CARTESIAN_POINT('Ctrl Pts',(-3.06908080882254,-2.16741813460255,297.));
#9394=CARTESIAN_POINT('Ctrl Pts',(-3.10194238684353,-2.10748369667657,297.));
#9395=CARTESIAN_POINT('Ctrl Pts',(-3.11090507486663,-2.09113713934972,297.));
#9396=CARTESIAN_POINT('Ctrl Pts',(-3.11975419834814,-2.07472221701618,297.));
#9397=CARTESIAN_POINT('Ctrl Pts',(-3.12848132276822,-2.05825471066704,297.));
#9398=CARTESIAN_POINT('Ctrl Pts',(-3.18408615702895,-1.95333206751959,297.));
#9399=CARTESIAN_POINT('Ctrl Pts',(-3.23481830075119,-1.84613953636477,297.));
#9400=CARTESIAN_POINT('Ctrl Pts',(-3.28051179803537,-1.73705586719653,297.));
#9401=CARTESIAN_POINT('Ctrl Pts',(-3.32587389771413,-1.62876334050814,297.));
#9402=CARTESIAN_POINT('Ctrl Pts',(-3.36627038976648,-1.51860614079287,297.));
#9403=CARTESIAN_POINT('Ctrl Pts',(-3.40148946203064,-1.40694277436367,297.));
#9404=CARTESIAN_POINT('Ctrl Pts',(-3.43581642062762,-1.29810788719042,297.));
#9405=CARTESIAN_POINT('Ctrl Pts',(-3.4652249691995,-1.18784142279203,297.));
#9406=CARTESIAN_POINT('Ctrl Pts',(-3.48947021542989,-1.07647566774693,297.));
#9407=CARTESIAN_POINT('Ctrl Pts',(-3.50639009325733,-0.998757547187614,
297.));
#9408=CARTESIAN_POINT('Ctrl Pts',(-3.52079437228538,-0.920504057101386,
297.));
#9409=CARTESIAN_POINT('Ctrl Pts',(-3.53258497104414,-0.841831067608438,
297.));
#9410=CARTESIAN_POINT('Ctrl Pts',(-3.53678136293646,-0.813830564664707,
297.));
#9411=CARTESIAN_POINT('Ctrl Pts',(-3.54064655877754,-0.785776955752405,
297.));
#9412=CARTESIAN_POINT('Ctrl Pts',(-3.54417574632832,-0.757675588895275,
297.));
#9413=CARTESIAN_POINT('Ctrl Pts',(-3.54658855565722,-0.738463450369874,
297.));
#9414=CARTESIAN_POINT('Ctrl Pts',(-3.54884441401843,-0.719227172536132,
297.));
#9415=CARTESIAN_POINT('Ctrl Pts',(-3.55093961590336,-0.699990393966351,
297.));
#9416=CARTESIAN_POINT('Ctrl Pts',(-3.56306129535751,-0.588697031149804,
297.));
#9417=CARTESIAN_POINT('Ctrl Pts',(-3.56983156372365,-0.477223248990884,
297.));
#9418=CARTESIAN_POINT('Ctrl Pts',(-3.57106196810248,-0.365887824980338,
297.));
#9419=CARTESIAN_POINT('Ctrl Pts',(-3.57193436072074,-0.286947759642042,
297.));
#9420=CARTESIAN_POINT('Ctrl Pts',(-3.57002072133686,-0.208077152176203,
297.));
#9421=CARTESIAN_POINT('Ctrl Pts',(-3.56523803549323,-0.129391528174488,
297.));
#9422=CARTESIAN_POINT('Ctrl Pts',(-3.5583383934639,-0.0158773530401223,
297.));
#9423=CARTESIAN_POINT('Ctrl Pts',(-3.54546949243385,0.0972530756745339,
297.));
#9424=CARTESIAN_POINT('Ctrl Pts',(-3.52684415090893,0.209634660021319,297.));
#9425=CARTESIAN_POINT('Ctrl Pts',(-3.50828799890508,0.321598768640824,297.));
#9426=CARTESIAN_POINT('Ctrl Pts',(-3.48401750053588,0.432820345922119,297.));
#9427=CARTESIAN_POINT('Ctrl Pts',(-3.45419980180639,0.542910574102145,297.));
#9428=CARTESIAN_POINT('Ctrl Pts',(-3.44899732296649,0.562118699041036,297.));
#9429=CARTESIAN_POINT('Ctrl Pts',(-3.44362588238673,0.581292298646908,297.));
#9430=CARTESIAN_POINT('Ctrl Pts',(-3.43808625278056,0.600429194129876,297.));
#9431=CARTESIAN_POINT('Ctrl Pts',(-3.43195656329836,0.621604477551889,297.));
#9432=CARTESIAN_POINT('Ctrl Pts',(-3.42562070782981,0.642735019730582,297.));
#9433=CARTESIAN_POINT('Ctrl Pts',(-3.41908837506188,0.663791541218352,297.));
#9434=CARTESIAN_POINT('Ctrl Pts',(-3.38609238768416,0.770151817387931,297.));
#9435=CARTESIAN_POINT('Ctrl Pts',(-3.34803954138042,0.874794555533513,297.));
#9436=CARTESIAN_POINT('Ctrl Pts',(-3.30516552460409,0.977392176481827,297.));
#9437=CARTESIAN_POINT('Ctrl Pts',(-3.26223302087613,1.08012975684018,297.));
#9438=CARTESIAN_POINT('Ctrl Pts',(-3.2144655987723,1.1808173900939,297.));
#9439=CARTESIAN_POINT('Ctrl Pts',(-3.16205541704689,1.27909866910512,297.));
#9440=CARTESIAN_POINT('Ctrl Pts',(-3.11058511725006,1.37561745092552,297.));
#9441=CARTESIAN_POINT('Ctrl Pts',(-3.0546364418454,1.46981598829565,297.));
#9442=CARTESIAN_POINT('Ctrl Pts',(-2.99435779069831,1.5613205369265,297.));
#9443=CARTESIAN_POINT('Ctrl Pts',(-2.94203711605949,1.64074467176993,297.));
#9444=CARTESIAN_POINT('Ctrl Pts',(-2.88645356779812,1.71813888458468,297.));
#9445=CARTESIAN_POINT('Ctrl Pts',(-2.82768844580675,1.79323101137441,297.));
#9446=CARTESIAN_POINT('Ctrl Pts',(-2.81808060469522,1.80550824655191,297.));
#9447=CARTESIAN_POINT('Ctrl Pts',(-2.80839358794498,1.8177163353674,297.));
#9448=CARTESIAN_POINT('Ctrl Pts',(-2.7986290191487,1.8298530527289,297.));
#9449=CARTESIAN_POINT('Ctrl Pts',(-2.73124593785801,1.91360579487594,297.));
#9450=CARTESIAN_POINT('Ctrl Pts',(-2.66015654899076,1.99398334177554,297.));
#9451=CARTESIAN_POINT('Ctrl Pts',(-2.58553694647172,2.07066463497472,297.));
#9452=CARTESIAN_POINT('Ctrl Pts',(-2.51196902352116,2.14626519138864,297.));
#9453=CARTESIAN_POINT('Ctrl Pts',(-2.43496910430356,2.21827345872741,297.));
#9454=CARTESIAN_POINT('Ctrl Pts',(-2.35467764042612,2.28634088207263,297.));
#9455=CARTESIAN_POINT('Ctrl Pts',(-2.27685756127256,2.35231317871164,297.));
#9456=CARTESIAN_POINT('Ctrl Pts',(-2.19594490517152,2.41458378331137,297.));
#9457=CARTESIAN_POINT('Ctrl Pts',(-2.11204909346534,2.47279110641631,297.));
#9458=CARTESIAN_POINT('Ctrl Pts',(-2.03442340485464,2.5266481875544,297.));
#9459=CARTESIAN_POINT('Ctrl Pts',(-1.95424336070402,2.57702649732872,297.));
#9460=CARTESIAN_POINT('Ctrl Pts',(-1.87158653173917,2.62360084935051,297.));
#9461=CARTESIAN_POINT('Ctrl Pts',(-2.28393822976682,3.20620192138523,296.587776945939));
#9462=CARTESIAN_POINT('Ctrl Pts',(-3.33986665587357,2.45409656577389,296.653293691435));
#9463=CARTESIAN_POINT('Ctrl Pts',(-4.63155725221788,-0.163320862335666,
296.784282531451));
#9464=CARTESIAN_POINT('Ctrl Pts',(-2.41439620993322,-3.96156897885787,296.980743465989));
#9465=CARTESIAN_POINT('Ctrl Pts',(1.97539585625794,-4.19463976840236,297.177159749549));
#9466=CARTESIAN_POINT('Ctrl Pts',(4.58908114628793,-0.663851457345065,297.373576033109));
#9467=CARTESIAN_POINT('Ctrl Pts',(3.08227572751309,3.46466062107002,297.569992316669));
#9468=CARTESIAN_POINT('Ctrl Pts',(-1.19318341285997,4.48082852509293,297.766408600229));
#9469=CARTESIAN_POINT('Ctrl Pts',(-4.396827278237,1.47308898323638,297.96282488379));
#9470=CARTESIAN_POINT('Ctrl Pts',(-3.65176790097364,-2.85779510217247,298.15924116735));
#9471=CARTESIAN_POINT('Ctrl Pts',(0.373002120370937,-4.62201032653495,298.35565745091));
#9472=CARTESIAN_POINT('Ctrl Pts',(4.06275569155672,-2.23521956363059,298.55207373447));
#9473=CARTESIAN_POINT('Ctrl Pts',(4.10374682531429,2.15904495645791,298.748490018031));
#9474=CARTESIAN_POINT('Ctrl Pts',(0.459145965957643,4.61425709863479,298.944906301591));
#9475=CARTESIAN_POINT('Ctrl Pts',(-3.59781293903473,2.92539499921914,299.141322585151));
#9476=CARTESIAN_POINT('Ctrl Pts',(-4.42356653331032,-1.3907746702388,299.337738868711));
#9477=CARTESIAN_POINT('Ctrl Pts',(-1.27650149624862,-4.45788471095139,299.534155152271));
#9478=CARTESIAN_POINT('Ctrl Pts',(3.01699305348801,-3.52135574899054,299.730571435832));
#9479=CARTESIAN_POINT('Ctrl Pts',(4.600917373614,0.577713353443416,299.926987719392));
#9480=CARTESIAN_POINT('Ctrl Pts',(2.05274420541422,4.15793630930791,300.123404002952));
#9481=CARTESIAN_POINT('Ctrl Pts',(-2.33900455103209,4.00390446639706,300.319820286512));
#9482=CARTESIAN_POINT('Ctrl Pts',(-4.6300864471361,0.253954218616865,300.516236570073));
#9483=CARTESIAN_POINT('Ctrl Pts',(-2.76287407130117,-3.72407305174658,300.712652853633));
#9484=CARTESIAN_POINT('Ctrl Pts',(1.58568363771314,-4.35749935687765,300.909069137193));
#9485=CARTESIAN_POINT('Ctrl Pts',(4.51013420556256,-1.07744266171838,301.105485420753));
#9486=CARTESIAN_POINT('Ctrl Pts',(3.38401996759768,3.17026845839884,301.301901704314));
#9487=CARTESIAN_POINT('Ctrl Pts',(-0.781292563612361,4.57075214501524,301.498317987873));
#9488=CARTESIAN_POINT('Ctrl Pts',(-4.24492394387617,1.8662298763172,301.694734271434));
#9489=CARTESIAN_POINT('Ctrl Pts',(-3.89617663551077,-2.51435893727449,301.891150554994));
#9490=CARTESIAN_POINT('Ctrl Pts',(-0.0482616226496284,-4.63679458860285,
302.087566838554));
#9491=CARTESIAN_POINT('Ctrl Pts',(3.84299729542567,-2.5949113716598,302.283983122115));
#9492=CARTESIAN_POINT('Ctrl Pts',(4.28284903123359,1.77746938571041,302.480399405675));
#9493=CARTESIAN_POINT('Ctrl Pts',(0.876261445153081,4.55349965672981,302.676815689235));
#9494=CARTESIAN_POINT('Ctrl Pts',(-3.31729912253674,3.24001848146433,302.873231972795));
#9495=CARTESIAN_POINT('Ctrl Pts',(-4.53158358723572,-0.983332825142458,
303.069648256355));
#9496=CARTESIAN_POINT('Ctrl Pts',(-1.67603948710785,-4.32355003480224,303.266064539916));
#9497=CARTESIAN_POINT('Ctrl Pts',(2.68476059529826,-3.78077421582624,303.462480823476));
#9498=CARTESIAN_POINT('Ctrl Pts',(4.63436931529892,0.157526020028036,303.658897107036));
#9499=CARTESIAN_POINT('Ctrl Pts',(2.42183724715278,3.95435174763791,303.855313390597));
#9500=CARTESIAN_POINT('Ctrl Pts',(-1.96575384247124,4.19976237385744,304.051729674156));
#9501=CARTESIAN_POINT('Ctrl Pts',(-4.58789591526953,0.673354385635241,304.248145957717));
#9502=CARTESIAN_POINT('Ctrl Pts',(-3.08963453431999,-3.45779587166151,304.444562241277));
#9503=CARTESIAN_POINT('Ctrl Pts',(1.18343537924031,-4.48348796067515,304.640978524837));
#9504=CARTESIAN_POINT('Ctrl Pts',(4.39366134024968,-1.48254954638245,304.837394808398));
#9505=CARTESIAN_POINT('Ctrl Pts',(3.65792106471558,2.84987785549197,305.033811091958));
#9506=CARTESIAN_POINT('Ctrl Pts',(-0.3629960006453,4.62280693344557,305.230227375518));
#9507=CARTESIAN_POINT('Ctrl Pts',(-4.05793271056506,2.24401064282424,305.426643659078));
#9508=CARTESIAN_POINT('Ctrl Pts',(-4.10836974515988,-2.15020447963357,305.623059942638));
#9509=CARTESIAN_POINT('Ctrl Pts',(-0.469191989355248,-4.61317350694027,
305.819476226199));
#9510=CARTESIAN_POINT('Ctrl Pts',(3.59163297431157,-2.93333759691029,306.015892509759));
#9511=CARTESIAN_POINT('Ctrl Pts',(4.42624039881829,1.38157897222829,306.212308793319));
#9512=CARTESIAN_POINT('Ctrl Pts',(1.28683256078006,4.45435220162257,306.408725076879));
#9513=CARTESIAN_POINT('Ctrl Pts',(-3.0107876642197,3.52965939911648,306.60514136044));
#9514=CARTESIAN_POINT('Ctrl Pts',(-4.59869662196651,-0.570614468679802,
306.801557644));
#9515=CARTESIAN_POINT('Ctrl Pts',(-2.91065832330177,-2.94999883844826,306.93250183304));
#9516=CARTESIAN_POINT('Ctrl Pts',(-1.75025476627565,-3.5260053049299,306.99797392756));
#9517=CARTESIAN_POINT('Ctrl Pts',(-2.14477093771142,3.01083830192886,296.726262181086));
#9518=CARTESIAN_POINT('Ctrl Pts',(-3.13635843824042,2.30456100957975,296.791778926582));
#9519=CARTESIAN_POINT('Ctrl Pts',(-4.34934240402712,-0.153369226231343,
296.922767766599));
#9520=CARTESIAN_POINT('Ctrl Pts',(-2.26727971697993,-3.72017855073993,297.119228701135));
#9521=CARTESIAN_POINT('Ctrl Pts',(1.85502898798194,-3.9390476293032,297.315644984695));
#9522=CARTESIAN_POINT('Ctrl Pts',(4.30945449622017,-0.623400972107909,297.512061268256));
#9523=CARTESIAN_POINT('Ctrl Pts',(2.89446330738038,3.25354832817121,297.708477551816));
#9524=CARTESIAN_POINT('Ctrl Pts',(-1.12047912413229,4.20779803596913,297.904893835376));
#9525=CARTESIAN_POINT('Ctrl Pts',(-4.12891524017367,1.38332919810655,298.101310118936));
#9526=CARTESIAN_POINT('Ctrl Pts',(-3.42925459331503,-2.68366096823,298.297726402497));
#9527=CARTESIAN_POINT('Ctrl Pts',(0.350273968468058,-4.34037720151753,298.494142686057));
#9528=CARTESIAN_POINT('Ctrl Pts',(3.81519964975679,-2.09902084784856,298.690558969617));
#9529=CARTESIAN_POINT('Ctrl Pts',(3.85369306925529,2.02748779081302,298.886975253177));
#9530=CARTESIAN_POINT('Ctrl Pts',(0.431168807947103,4.33309640133782,299.083391536737));
#9531=CARTESIAN_POINT('Ctrl Pts',(-3.378587271054,2.74714179826662,299.279807820298));
#9532=CARTESIAN_POINT('Ctrl Pts',(-4.15402519123534,-1.3060305461667,299.476224103858));
#9533=CARTESIAN_POINT('Ctrl Pts',(-1.1987203836851,-4.18625225809752,299.672640387418));
#9534=CARTESIAN_POINT('Ctrl Pts',(2.83315850492985,-3.30678884977944,299.869056670978));
#9535=CARTESIAN_POINT('Ctrl Pts',(4.32056950627178,0.542511524455615,300.065472954539));
#9536=CARTESIAN_POINT('Ctrl Pts',(1.92766426733765,3.90458062343006,300.261889238099));
#9537=CARTESIAN_POINT('Ctrl Pts',(-2.19648190080015,3.75993440846169,300.458305521659));
#9538=CARTESIAN_POINT('Ctrl Pts',(-4.34796121956542,0.238480016884807,300.654721805219));
#9539=CARTESIAN_POINT('Ctrl Pts',(-2.59452376401972,-3.49715397167979,300.851138088779));
#9540=CARTESIAN_POINT('Ctrl Pts',(1.4890631183659,-4.09198368849123,301.047554372339));
#9541=CARTESIAN_POINT('Ctrl Pts',(4.23531803233416,-1.01179080843177,301.2439706559));
#9542=CARTESIAN_POINT('Ctrl Pts',(3.17782135459926,2.97709437396264,301.44038693946));
#9543=CARTESIAN_POINT('Ctrl Pts',(-0.733686035132803,4.29224233665535,301.63680322302));
#9544=CARTESIAN_POINT('Ctrl Pts',(-3.98626783726566,1.75251482270716,301.833219506581));
#9545=CARTESIAN_POINT('Ctrl Pts',(-3.6587707614522,-2.36115141178396,302.029635790141));
#9546=CARTESIAN_POINT('Ctrl Pts',(-0.0453208954238121,-4.35426061360174,
302.226052073701));
#9547=CARTESIAN_POINT('Ctrl Pts',(3.60883180005007,-2.43679554172575,302.422468357261));
#9548=CARTESIAN_POINT('Ctrl Pts',(4.02188203388193,1.66916277833516,302.618884640821));
#9549=CARTESIAN_POINT('Ctrl Pts',(0.822868174325886,4.27604109487238,302.815300924382));
#9550=CARTESIAN_POINT('Ctrl Pts',(-3.11516601324143,3.0425943163104,303.011717207942));
#9551=CARTESIAN_POINT('Ctrl Pts',(-4.25546043804587,-0.923415369985092,
303.208133491502));
#9552=CARTESIAN_POINT('Ctrl Pts',(-1.57391331147019,-4.06010300170498,303.404549775062));
#9553=CARTESIAN_POINT('Ctrl Pts',(2.52116997931962,-3.55040016164564,303.600966058622));
#9554=CARTESIAN_POINT('Ctrl Pts',(4.35198311956513,0.147927481262918,303.797382342183));
#9555=CARTESIAN_POINT('Ctrl Pts',(2.27426734920524,3.71340108733503,303.993798625743));
#9556=CARTESIAN_POINT('Ctrl Pts',(-1.8459744913755,3.9438580988519,304.190214909303));
#9557=CARTESIAN_POINT('Ctrl Pts',(-4.30834148492695,0.632324858119486,304.386631192864));
#9558=CARTESIAN_POINT('Ctrl Pts',(-2.9013737197418,-3.24710186879059,304.583047476424));
#9559=CARTESIAN_POINT('Ctrl Pts',(1.11132506780329,-4.21029542406532,304.779463759984));
#9560=CARTESIAN_POINT('Ctrl Pts',(4.12594221240204,-1.39221330041091,304.975880043544));
#9561=CARTESIAN_POINT('Ctrl Pts',(3.43503282610466,2.67622614343233,305.172296327104));
#9562=CARTESIAN_POINT('Ctrl Pts',(-0.340877552003241,4.34112526875001,305.368712610665));
#9563=CARTESIAN_POINT('Ctrl Pts',(-3.81067054764307,2.10727625989075,305.565128894225));
#9564=CARTESIAN_POINT('Ctrl Pts',(-3.8580343005561,-2.01918599108778,305.761545177785));
#9565=CARTESIAN_POINT('Ctrl Pts',(-0.440602696631977,-4.33207883617583,
305.957961461345));
#9566=CARTESIAN_POINT('Ctrl Pts',(3.37278387034834,-2.7546004293609,306.154377744905));
#9567=CARTESIAN_POINT('Ctrl Pts',(4.15653612999808,1.29739516996088,306.350794028466));
#9568=CARTESIAN_POINT('Ctrl Pts',(1.20842194508195,4.1829349952894,306.547210312026));
#9569=CARTESIAN_POINT('Ctrl Pts',(-2.8273312288738,3.31458653328722,306.743626595586));
#9570=CARTESIAN_POINT('Ctrl Pts',(-4.31848407176599,-0.535845196298082,
306.940042879146));
#9571=CARTESIAN_POINT('Ctrl Pts',(-2.73330307276428,-2.77024645085618,307.070987068187));
#9572=CARTESIAN_POINT('Ctrl Pts',(-1.64360642830614,-3.31115509415596,307.136459162707));
#9573=CARTESIAN_POINT('Ctrl Pts',(-2.00560364565601,2.81547468247249,296.864747416232));
#9574=CARTESIAN_POINT('Ctrl Pts',(-2.93285022060727,2.15502545338563,296.930264161729));
#9575=CARTESIAN_POINT('Ctrl Pts',(-4.06712755583635,-0.143417590127015,
297.061253001746));
#9576=CARTESIAN_POINT('Ctrl Pts',(-2.12016322402664,-3.478788122622,297.257713936283));
#9577=CARTESIAN_POINT('Ctrl Pts',(1.73466211970593,-3.68345549020403,297.454130219843));
#9578=CARTESIAN_POINT('Ctrl Pts',(4.0298278461524,-0.582950486870754,297.650546503403));
#9579=CARTESIAN_POINT('Ctrl Pts',(2.70665088724769,3.04243603527242,297.846962786964));
#9580=CARTESIAN_POINT('Ctrl Pts',(-1.04777483540462,3.93476754684532,298.043379070524));
#9581=CARTESIAN_POINT('Ctrl Pts',(-3.86100320211035,1.29356941297673,298.239795354084));
#9582=CARTESIAN_POINT('Ctrl Pts',(-3.20674128565643,-2.50952683428754,298.436211637644));
#9583=CARTESIAN_POINT('Ctrl Pts',(0.327545816565179,-4.05874407650011,298.632627921204));
#9584=CARTESIAN_POINT('Ctrl Pts',(3.56764360795687,-1.96282213206653,298.829044204765));
#9585=CARTESIAN_POINT('Ctrl Pts',(3.60363931319628,1.89593062516814,299.025460488325));
#9586=CARTESIAN_POINT('Ctrl Pts',(0.403191649936562,4.05193570404087,299.221876771885));
#9587=CARTESIAN_POINT('Ctrl Pts',(-3.15936160307328,2.56888859731411,299.418293055445));
#9588=CARTESIAN_POINT('Ctrl Pts',(-3.88448384916037,-1.2212864220946,299.614709339006));
#9589=CARTESIAN_POINT('Ctrl Pts',(-1.12093927112159,-3.91461980524366,299.811125622566));
#9590=CARTESIAN_POINT('Ctrl Pts',(2.64932395637171,-3.09222195056834,300.007541906126));
#9591=CARTESIAN_POINT('Ctrl Pts',(4.04022163892955,0.507309695467813,300.203958189686));
#9592=CARTESIAN_POINT('Ctrl Pts',(1.80258432926109,3.65122493755221,300.400374473246));
#9593=CARTESIAN_POINT('Ctrl Pts',(-2.05395925056823,3.51596435052632,300.596790756806));
#9594=CARTESIAN_POINT('Ctrl Pts',(-4.06583599199474,0.223005815152753,300.793207040367));
#9595=CARTESIAN_POINT('Ctrl Pts',(-2.42617345673829,-3.270234891613,300.989623323927));
#9596=CARTESIAN_POINT('Ctrl Pts',(1.39244259901866,-3.82646802010482,301.186039607487));
#9597=CARTESIAN_POINT('Ctrl Pts',(3.96050185910575,-0.946138955145171,301.382455891047));
#9598=CARTESIAN_POINT('Ctrl Pts',(2.97162274160084,2.78392028952646,301.578872174608));
#9599=CARTESIAN_POINT('Ctrl Pts',(-0.686079506653246,4.01373252829545,301.775288458168));
#9600=CARTESIAN_POINT('Ctrl Pts',(-3.72761173065515,1.63879976909712,301.971704741728));
#9601=CARTESIAN_POINT('Ctrl Pts',(-3.42136488739364,-2.20794388629344,302.168121025288));
#9602=CARTESIAN_POINT('Ctrl Pts',(-0.0423801681979951,-4.07172663860065,
302.364537308849));
#9603=CARTESIAN_POINT('Ctrl Pts',(3.37466630467447,-2.27867971179171,302.560953592409));
#9604=CARTESIAN_POINT('Ctrl Pts',(3.76091503653028,1.56085617095991,302.757369875969));
#9605=CARTESIAN_POINT('Ctrl Pts',(0.769474903498698,3.99858253301496,302.953786159529));
#9606=CARTESIAN_POINT('Ctrl Pts',(-2.91303290394612,2.84517015115646,303.150202443089));
#9607=CARTESIAN_POINT('Ctrl Pts',(-3.97933728885602,-0.86349791482772,303.34661872665));
#9608=CARTESIAN_POINT('Ctrl Pts',(-1.47178713583252,-3.79665596860773,303.54303501021));
#9609=CARTESIAN_POINT('Ctrl Pts',(2.35757936334099,-3.32002610746504,303.73945129377));
#9610=CARTESIAN_POINT('Ctrl Pts',(4.06959692383135,0.138328942497795,303.93586757733));
#9611=CARTESIAN_POINT('Ctrl Pts',(2.1266974512577,3.47245042703215,304.132283860891));
#9612=CARTESIAN_POINT('Ctrl Pts',(-1.72619514027976,3.68795382384636,304.328700144451));
#9613=CARTESIAN_POINT('Ctrl Pts',(-4.02878705458437,0.591295330603737,304.525116428011));
#9614=CARTESIAN_POINT('Ctrl Pts',(-2.7131129051636,-3.03640786591968,304.721532711571));
#9615=CARTESIAN_POINT('Ctrl Pts',(1.03921475636626,-3.93710288745548,304.917948995132));
#9616=CARTESIAN_POINT('Ctrl Pts',(3.8582230845544,-1.30187705443938,305.114365278692));
#9617=CARTESIAN_POINT('Ctrl Pts',(3.21214458749373,2.50257443137269,305.310781562252));
#9618=CARTESIAN_POINT('Ctrl Pts',(-0.318759103361179,4.05944360405444,305.507197845812));
#9619=CARTESIAN_POINT('Ctrl Pts',(-3.56340838472108,1.97054187695727,305.703614129372));
#9620=CARTESIAN_POINT('Ctrl Pts',(-3.60769885595232,-1.888167502542,305.900030412933));
#9621=CARTESIAN_POINT('Ctrl Pts',(-0.412013403908709,-4.05098416541141,
306.096446696493));
#9622=CARTESIAN_POINT('Ctrl Pts',(3.15393476638512,-2.57586326181149,306.292862980053));
#9623=CARTESIAN_POINT('Ctrl Pts',(3.88683186117788,1.21321136769346,306.489279263613));
#9624=CARTESIAN_POINT('Ctrl Pts',(1.13001132938383,3.91151778895623,306.685695547173));
#9625=CARTESIAN_POINT('Ctrl Pts',(-2.6438747935279,3.09951366745796,306.882111830734));
#9626=CARTESIAN_POINT('Ctrl Pts',(-4.03827152156548,-0.50107592391636,307.078528114294));
#9627=CARTESIAN_POINT('Ctrl Pts',(-2.5559478222268,-2.5904940632641,307.209472303334));
#9628=CARTESIAN_POINT('Ctrl Pts',(-1.53695809033663,-3.09630488338201,307.274944397854));
#9629=CARTESIAN_POINT('Ctrl Pts',(-1.86643635360062,2.62011106301612,297.00323265138));
#9630=CARTESIAN_POINT('Ctrl Pts',(-2.72934200297413,2.00548989719149,297.068749396876));
#9631=CARTESIAN_POINT('Ctrl Pts',(-3.7849127076456,-0.13346595402269,297.199738236893));
#9632=CARTESIAN_POINT('Ctrl Pts',(-1.97304673107334,-3.23739769450407,297.396199171429));
#9633=CARTESIAN_POINT('Ctrl Pts',(1.61429525142993,-3.42786335110486,297.59261545499));
#9634=CARTESIAN_POINT('Ctrl Pts',(3.75020119608464,-0.542500001633599,297.78903173855));
#9635=CARTESIAN_POINT('Ctrl Pts',(2.51883846711499,2.83132374237361,297.98544802211));
#9636=CARTESIAN_POINT('Ctrl Pts',(-0.97507054667695,3.66173705772152,298.18186430567));
#9637=CARTESIAN_POINT('Ctrl Pts',(-3.59309116404703,1.20380962784691,298.378280589231));
#9638=CARTESIAN_POINT('Ctrl Pts',(-2.98422797799783,-2.33539270034508,298.574696872791));
#9639=CARTESIAN_POINT('Ctrl Pts',(0.304817664662298,-3.7771109514827,298.771113156351));
#9640=CARTESIAN_POINT('Ctrl Pts',(3.32008756615693,-1.82662341628449,298.967529439911));
#9641=CARTESIAN_POINT('Ctrl Pts',(3.35358555713727,1.76437345952326,299.163945723471));
#9642=CARTESIAN_POINT('Ctrl Pts',(0.375214491926022,3.77077500674391,299.360362007032));
#9643=CARTESIAN_POINT('Ctrl Pts',(-2.94013593509256,2.39063539636159,299.556778290592));
#9644=CARTESIAN_POINT('Ctrl Pts',(-3.61494250708539,-1.13654229802251,299.753194574152));
#9645=CARTESIAN_POINT('Ctrl Pts',(-1.04315815855808,-3.64298735238979,299.949610857712));
#9646=CARTESIAN_POINT('Ctrl Pts',(2.46548940781356,-2.87765505135725,300.146027141273));
#9647=CARTESIAN_POINT('Ctrl Pts',(3.75987377158732,0.472107866480012,300.342443424833));
#9648=CARTESIAN_POINT('Ctrl Pts',(1.67750439118453,3.39786925167437,300.538859708393));
#9649=CARTESIAN_POINT('Ctrl Pts',(-1.9114366003363,3.27199429259095,300.735275991953));
#9650=CARTESIAN_POINT('Ctrl Pts',(-3.78371076442406,0.207531613420697,300.931692275514));
#9651=CARTESIAN_POINT('Ctrl Pts',(-2.25782314945684,-3.04331581154621,301.128108559074));
#9652=CARTESIAN_POINT('Ctrl Pts',(1.29582207967142,-3.5609523517184,301.324524842634));
#9653=CARTESIAN_POINT('Ctrl Pts',(3.68568568587734,-0.880487101858563,301.520941126194));
#9654=CARTESIAN_POINT('Ctrl Pts',(2.76542412860242,2.59074620509027,301.717357409755));
#9655=CARTESIAN_POINT('Ctrl Pts',(-0.638472978173689,3.73522271993555,301.913773693315));
#9656=CARTESIAN_POINT('Ctrl Pts',(-3.46895562404465,1.52508471548708,302.110189976875));
#9657=CARTESIAN_POINT('Ctrl Pts',(-3.18395901333507,-2.05473636080292,302.306606260435));
#9658=CARTESIAN_POINT('Ctrl Pts',(-0.0394394409721774,-3.78919266359954,
302.503022543995));
#9659=CARTESIAN_POINT('Ctrl Pts',(3.14050080929887,-2.12056388185767,302.699438827556));
#9660=CARTESIAN_POINT('Ctrl Pts',(3.49994803917864,1.45254956358465,302.895855111116));
#9661=CARTESIAN_POINT('Ctrl Pts',(0.716081632671503,3.72112397115754,303.092271394676));
#9662=CARTESIAN_POINT('Ctrl Pts',(-2.71089979465081,2.64774598600254,303.288687678236));
#9663=CARTESIAN_POINT('Ctrl Pts',(-3.70321413966617,-0.803580459670354,
303.485103961796));
#9664=CARTESIAN_POINT('Ctrl Pts',(-1.36966096019486,-3.53320893551047,303.681520245357));
#9665=CARTESIAN_POINT('Ctrl Pts',(2.19398874736236,-3.08965205328445,303.877936528917));
#9666=CARTESIAN_POINT('Ctrl Pts',(3.78721072809757,0.128730403732677,304.074352812477));
#9667=CARTESIAN_POINT('Ctrl Pts',(1.97912755331017,3.23149976672927,304.270769096037));
#9668=CARTESIAN_POINT('Ctrl Pts',(-1.60641578918403,3.43204954884082,304.467185379597));
#9669=CARTESIAN_POINT('Ctrl Pts',(-3.74923262424179,0.550265803087981,304.663601663158));
#9670=CARTESIAN_POINT('Ctrl Pts',(-2.52485209058541,-2.82571386304877,304.860017946718));
#9671=CARTESIAN_POINT('Ctrl Pts',(0.967104444929231,-3.66391035084566,305.056434230278));
#9672=CARTESIAN_POINT('Ctrl Pts',(3.59050395670676,-1.21154080846783,305.252850513839));
#9673=CARTESIAN_POINT('Ctrl Pts',(2.98925634888281,2.32892271931305,305.449266797398));
#9674=CARTESIAN_POINT('Ctrl Pts',(-0.29664065471912,3.77776193935887,305.645683080959));
#9675=CARTESIAN_POINT('Ctrl Pts',(-3.31614622179908,1.83380749402379,305.842099364519));
#9676=CARTESIAN_POINT('Ctrl Pts',(-3.35736341134853,-1.75714901399621,306.038515648079));
#9677=CARTESIAN_POINT('Ctrl Pts',(-0.383424111185439,-3.76988949464697,
306.23493193164));
#9678=CARTESIAN_POINT('Ctrl Pts',(2.93508566242189,-2.39712609426209,306.4313482152));
#9679=CARTESIAN_POINT('Ctrl Pts',(3.61712759235767,1.12902756542604,306.62776449876));
#9680=CARTESIAN_POINT('Ctrl Pts',(1.05160071368571,3.64010058262307,306.82418078232));
#9681=CARTESIAN_POINT('Ctrl Pts',(-2.460418358182,2.88444080162871,307.02059706588));
#9682=CARTESIAN_POINT('Ctrl Pts',(-3.75805897136496,-0.466306651534639,
307.217013349441));
#9683=CARTESIAN_POINT('Ctrl Pts',(-2.37859257168932,-2.41074167567201,307.347957538481));
#9684=CARTESIAN_POINT('Ctrl Pts',(-1.43030975236712,-2.88145467260807,307.413429633001));
#9685=CARTESIAN_POINT('',(-1.8740725398893,2.62480419192483,307.001415228007));
#9686=CARTESIAN_POINT('Ctrl Pts',(-1.87562241821632,2.62673369148108,307.));
#9687=CARTESIAN_POINT('Ctrl Pts',(-1.95770449094995,2.58115596232075,307.));
#9688=CARTESIAN_POINT('Ctrl Pts',(-2.03743863910024,2.53192586541867,307.));
#9689=CARTESIAN_POINT('Ctrl Pts',(-2.11454810906558,2.47911769610372,307.));
#9690=CARTESIAN_POINT('Ctrl Pts',(-2.19910585323819,2.42120860046132,307.));
#9691=CARTESIAN_POINT('Ctrl Pts',(-2.28050877294379,2.35899810945558,307.));
#9692=CARTESIAN_POINT('Ctrl Pts',(-2.35867943255216,2.29288564826134,307.));
#9693=CARTESIAN_POINT('Ctrl Pts',(-2.43922435958225,2.22476516175978,307.));
#9694=CARTESIAN_POINT('Ctrl Pts',(-2.51633824355233,2.1525017186583,307.));
#9695=CARTESIAN_POINT('Ctrl Pts',(-2.58991395366746,2.07648048712394,307.));
#9696=CARTESIAN_POINT('Ctrl Pts',(-2.66337435931201,2.00057839256892,307.));
#9697=CARTESIAN_POINT('Ctrl Pts',(-2.7333081306884,1.92092961365071,307.));
#9698=CARTESIAN_POINT('Ctrl Pts',(-2.79957919033415,1.83787484209342,307.));
#9699=CARTESIAN_POINT('Ctrl Pts',(-2.80893754976685,1.82614639819968,307.));
#9700=CARTESIAN_POINT('Ctrl Pts',(-2.81822281557543,1.8143499747194,307.));
#9701=CARTESIAN_POINT('Ctrl Pts',(-2.82743454884594,1.80248647431831,307.));
#9702=CARTESIAN_POINT('Ctrl Pts',(-2.83706693497037,1.79008122838958,307.));
#9703=CARTESIAN_POINT('Ctrl Pts',(-2.84661330232596,1.7776098546387,307.));
#9704=CARTESIAN_POINT('Ctrl Pts',(-2.85607185997111,1.76507574247541,307.));
#9705=CARTESIAN_POINT('Ctrl Pts',(-2.92166160942224,1.67815876134315,307.));
#9706=CARTESIAN_POINT('Ctrl Pts',(-2.98305537122714,1.58819739798644,307.));
#9707=CARTESIAN_POINT('Ctrl Pts',(-3.04016414393303,1.49562175005816,307.));
#9708=CARTESIAN_POINT('Ctrl Pts',(-3.09822312230499,1.40150578002114,307.));
#9709=CARTESIAN_POINT('Ctrl Pts',(-3.15185387969084,1.30468720717543,307.));
#9710=CARTESIAN_POINT('Ctrl Pts',(-3.20093354890556,1.20557190624194,307.));
#9711=CARTESIAN_POINT('Ctrl Pts',(-3.25050203129707,1.10546945796429,307.));
#9712=CARTESIAN_POINT('Ctrl Pts',(-3.29542889000202,1.00302358346718,307.));
#9713=CARTESIAN_POINT('Ctrl Pts',(-3.3355494236701,0.898615931380555,307.));
#9714=CARTESIAN_POINT('Ctrl Pts',(-3.35616396299268,0.844969694585103,307.));
#9715=CARTESIAN_POINT('Ctrl Pts',(-3.37550893595618,0.790805015894116,307.));
#9716=CARTESIAN_POINT('Ctrl Pts',(-3.39355738158136,0.736170952424262,307.));
#9717=CARTESIAN_POINT('Ctrl Pts',(-3.40458316148461,0.702795050058588,307.));
#9718=CARTESIAN_POINT('Ctrl Pts',(-3.41512501640732,0.669243942651207,307.));
#9719=CARTESIAN_POINT('Ctrl Pts',(-3.42517616166359,0.635528570480346,307.));
#9720=CARTESIAN_POINT('Ctrl Pts',(-3.4296359472032,0.62056874993885,307.));
#9721=CARTESIAN_POINT('Ctrl Pts',(-3.43399864147103,0.605577994095616,307.));
#9722=CARTESIAN_POINT('Ctrl Pts',(-3.43826050148757,0.59056902651178,307.));
#9723=CARTESIAN_POINT('Ctrl Pts',(-3.46965055336494,0.480022863743607,307.));
#9724=CARTESIAN_POINT('Ctrl Pts',(-3.49562521356327,0.368320523725974,307.));
#9725=CARTESIAN_POINT('Ctrl Pts',(-3.51606074258901,0.255892602399452,307.));
#9726=CARTESIAN_POINT('Ctrl Pts',(-3.53696881357864,0.140864948485883,307.));
#9727=CARTESIAN_POINT('Ctrl Pts',(-3.55207933732713,0.0250769828317131,
307.));
#9728=CARTESIAN_POINT('Ctrl Pts',(-3.56121413083353,-0.0910426031961557,
307.));
#9729=CARTESIAN_POINT('Ctrl Pts',(-3.57034892433994,-0.207162189224066,
307.));
#9730=CARTESIAN_POINT('Ctrl Pts',(-3.57350856690181,-0.323614351558602,
307.));
#9731=CARTESIAN_POINT('Ctrl Pts',(-3.57046020776024,-0.439989127307766,
307.));
#9732=CARTESIAN_POINT('Ctrl Pts',(-3.56844092581946,-0.51707764349632,307.));
#9733=CARTESIAN_POINT('Ctrl Pts',(-3.56369641416304,-0.594132558068256,
307.));
#9734=CARTESIAN_POINT('Ctrl Pts',(-3.5562979507555,-0.671059667724272,307.));
#9735=CARTESIAN_POINT('Ctrl Pts',(-3.55447014995795,-0.690064618433204,
307.));
#9736=CARTESIAN_POINT('Ctrl Pts',(-3.55248030988035,-0.70906176810033,307.));
#9737=CARTESIAN_POINT('Ctrl Pts',(-3.55032939438232,-0.72804969199813,307.));
#9738=CARTESIAN_POINT('Ctrl Pts',(-3.54825093279214,-0.746398004860717,
307.));
#9739=CARTESIAN_POINT('Ctrl Pts',(-3.54602283507798,-0.764730434923112,
307.));
#9740=CARTESIAN_POINT('Ctrl Pts',(-3.54364770171127,-0.78303604758736,307.));
#9741=CARTESIAN_POINT('Ctrl Pts',(-3.52915857158688,-0.894706578436623,
307.));
#9742=CARTESIAN_POINT('Ctrl Pts',(-3.50918968560073,-1.00548797552805,307.));
#9743=CARTESIAN_POINT('Ctrl Pts',(-3.48405567932025,-1.11508513485562,307.));
#9744=CARTESIAN_POINT('Ctrl Pts',(-3.45845720380376,-1.22670761829162,307.));
#9745=CARTESIAN_POINT('Ctrl Pts',(-3.42750082039565,-1.33710233523251,307.));
#9746=CARTESIAN_POINT('Ctrl Pts',(-3.39146415702186,-1.44596592372902,307.));
#9747=CARTESIAN_POINT('Ctrl Pts',(-3.3547045784688,-1.55701337535897,307.));
#9748=CARTESIAN_POINT('Ctrl Pts',(-3.31265870899318,-1.66646840900814,307.));
#9749=CARTESIAN_POINT('Ctrl Pts',(-3.26556674632985,-1.77400697166853,307.));
#9750=CARTESIAN_POINT('Ctrl Pts',(-3.22694700310801,-1.86219848974312,307.));
#9751=CARTESIAN_POINT('Ctrl Pts',(-3.18493241340503,-1.94910124535555,307.));
#9752=CARTESIAN_POINT('Ctrl Pts',(-3.13963017239118,-2.03452991644561,307.));
#9753=CARTESIAN_POINT('Ctrl Pts',(-3.13126875800696,-2.05029744810168,307.));
#9754=CARTESIAN_POINT('Ctrl Pts',(-3.12279528754488,-2.06601473950236,307.));
#9755=CARTESIAN_POINT('Ctrl Pts',(-3.11421035577053,-2.08168058964027,307.));
#9756=CARTESIAN_POINT('Ctrl Pts',(-3.10572159975257,-2.09717093751141,307.));
#9757=CARTESIAN_POINT('Ctrl Pts',(-3.09712808038243,-2.11260327499777,307.));
#9758=CARTESIAN_POINT('Ctrl Pts',(-3.08843198120147,-2.12797434134853,307.));
#9759=CARTESIAN_POINT('Ctrl Pts',(-3.02913621757971,-2.23278445194894,307.));
#9760=CARTESIAN_POINT('Ctrl Pts',(-2.96505698426078,-2.33477997371097,307.));
#9761=CARTESIAN_POINT('Ctrl Pts',(-2.8964711255631,-2.43362682562493,307.));
#9762=CARTESIAN_POINT('Ctrl Pts',(-2.82741050084661,-2.53315791664076,307.));
#9763=CARTESIAN_POINT('Ctrl Pts',(-2.75378032677603,-2.62949742827724,307.));
#9764=CARTESIAN_POINT('Ctrl Pts',(-2.67581266947912,-2.72228997936985,307.));
#9765=CARTESIAN_POINT('Ctrl Pts',(-2.6409583266364,-2.76377158214157,307.));
#9766=CARTESIAN_POINT('Ctrl Pts',(-2.60523653444311,-2.80454409027921,307.));
#9767=CARTESIAN_POINT('Ctrl Pts',(-2.56866505040167,-2.84457415493151,307.));
#9768=CARTESIAN_POINT('Ctrl Pts',(-2.54450137491384,-2.87102299936229,307.));
#9769=CARTESIAN_POINT('Ctrl Pts',(-2.51996073222418,-2.89715358568975,307.));
#9770=CARTESIAN_POINT('Ctrl Pts',(-2.49508271396498,-2.92292083144206,307.));
#9771=CARTESIAN_POINT('Ctrl Pts',(-2.40941490538101,-3.01165070750563,307.));
#9772=CARTESIAN_POINT('Ctrl Pts',(-2.31968801564158,-3.09614586137004,307.));
#9773=CARTESIAN_POINT('Ctrl Pts',(-2.22615742676719,-3.17605066264026,307.));
#9774=CARTESIAN_POINT('Ctrl Pts',(-2.13385009249119,-3.25491041633018,307.));
#9775=CARTESIAN_POINT('Ctrl Pts',(-2.03783742037138,-3.32929985577124,307.));
#9776=CARTESIAN_POINT('Ctrl Pts',(-1.93832242401188,-3.39885060197879,307.));
#9777=CARTESIAN_POINT('Ctrl Pts',(-1.87645376288492,-3.44209043221199,307.));
#9778=CARTESIAN_POINT('Ctrl Pts',(-1.81323059511134,-3.48345947870024,307.));
#9779=CARTESIAN_POINT('Ctrl Pts',(-1.74869447533109,-3.52286199445089,307.));
#9780=CARTESIAN_POINT('Ctrl Pts',(-1.83773660687461,2.64742171296018,307.));
#9781=CARTESIAN_POINT('Ctrl Pts',(-1.84943329741252,2.63930232787106,307.000471742669));
#9782=CARTESIAN_POINT('Ctrl Pts',(-1.86107617823706,2.63110542515543,307.000943485338));
#9783=CARTESIAN_POINT('Ctrl Pts',(-1.87266422666468,2.62283172481011,307.001415228007));
#9784=CARTESIAN_POINT('Origin',(0.,0.,307.));
#9785=CARTESIAN_POINT('Origin',(0.,0.,177.));
#19427=UNCERTAINTY_MEASURE_WITH_UNIT(LENGTH_MEASURE(0.01),#19444,
'DISTANCE_ACCURACY_VALUE',
'Maximum model space distance between geometric entities at asserted c
onnectivities');
#19433=UNCERTAINTY_MEASURE_WITH_UNIT(LENGTH_MEASURE(0.01),#19444,
'DISTANCE_ACCURACY_VALUE',
'Maximum model space distance between geometric entities at asserted c
onnectivities');
#19437=(
GEOMETRIC_REPRESENTATION_CONTEXT(3)
GLOBAL_UNCERTAINTY_ASSIGNED_CONTEXT((#19427))
GLOBAL_UNIT_ASSIGNED_CONTEXT((#19444,#19446,#19447))
REPRESENTATION_CONTEXT('','3D')
);
#19443=(
GEOMETRIC_REPRESENTATION_CONTEXT(3)
GLOBAL_UNCERTAINTY_ASSIGNED_CONTEXT((#19433))
GLOBAL_UNIT_ASSIGNED_CONTEXT((#19444,#19446,#19447))
REPRESENTATION_CONTEXT('','3D')
);
#19444=(
LENGTH_UNIT()
NAMED_UNIT(*)
SI_UNIT(.MILLI.,.METRE.)
);
#19446=(
NAMED_UNIT(*)
PLANE_ANGLE_UNIT()
SI_UNIT($,.RADIAN.)
);
#19447=(
NAMED_UNIT(*)
SI_UNIT($,.STERADIAN.)
SOLID_ANGLE_UNIT()
);
#19451=SHAPE_DEFINITION_REPRESENTATION(#19460,#19477);
#19460=PRODUCT_DEFINITION_SHAPE('',$,#19487);
#19477=SHAPE_REPRESENTATION('',(#2131),#19437);
#19483=PRODUCT_DEFINITION_CONTEXT('part definition',#19512,'design');
#19487=PRODUCT_DEFINITION('Rod','Rod',#19496,#19483);
#19496=PRODUCT_DEFINITION_FORMATION('',$,#19517);
#19512=APPLICATION_CONTEXT(
'Core Data for Automotive Mechanical Design Process');
#19513=PRODUCT_CONTEXT('part definition',#19512,'mechanical');
#19517=PRODUCT('Rod','Rod',$,(#19513));
#19524=PRESENTATION_STYLE_ASSIGNMENT((#19527));
#19527=SURFACE_STYLE_USAGE(.BOTH.,#19530);
#19530=SURFACE_SIDE_STYLE('',(#19533));
#19533=SURFACE_STYLE_FILL_AREA(#19536);
#19536=FILL_AREA_STYLE('Opaque(36,31,37)',(#19539));
#19539=FILL_AREA_STYLE_COLOUR('Opaque(36,31,37)',#19542);
#19542=COLOUR_RGB('Opaque(36,31,37)',0.141176470588235,0.12156862745098,
0.145098039215686);
ENDSEC;
END-ISO-10303-21;
